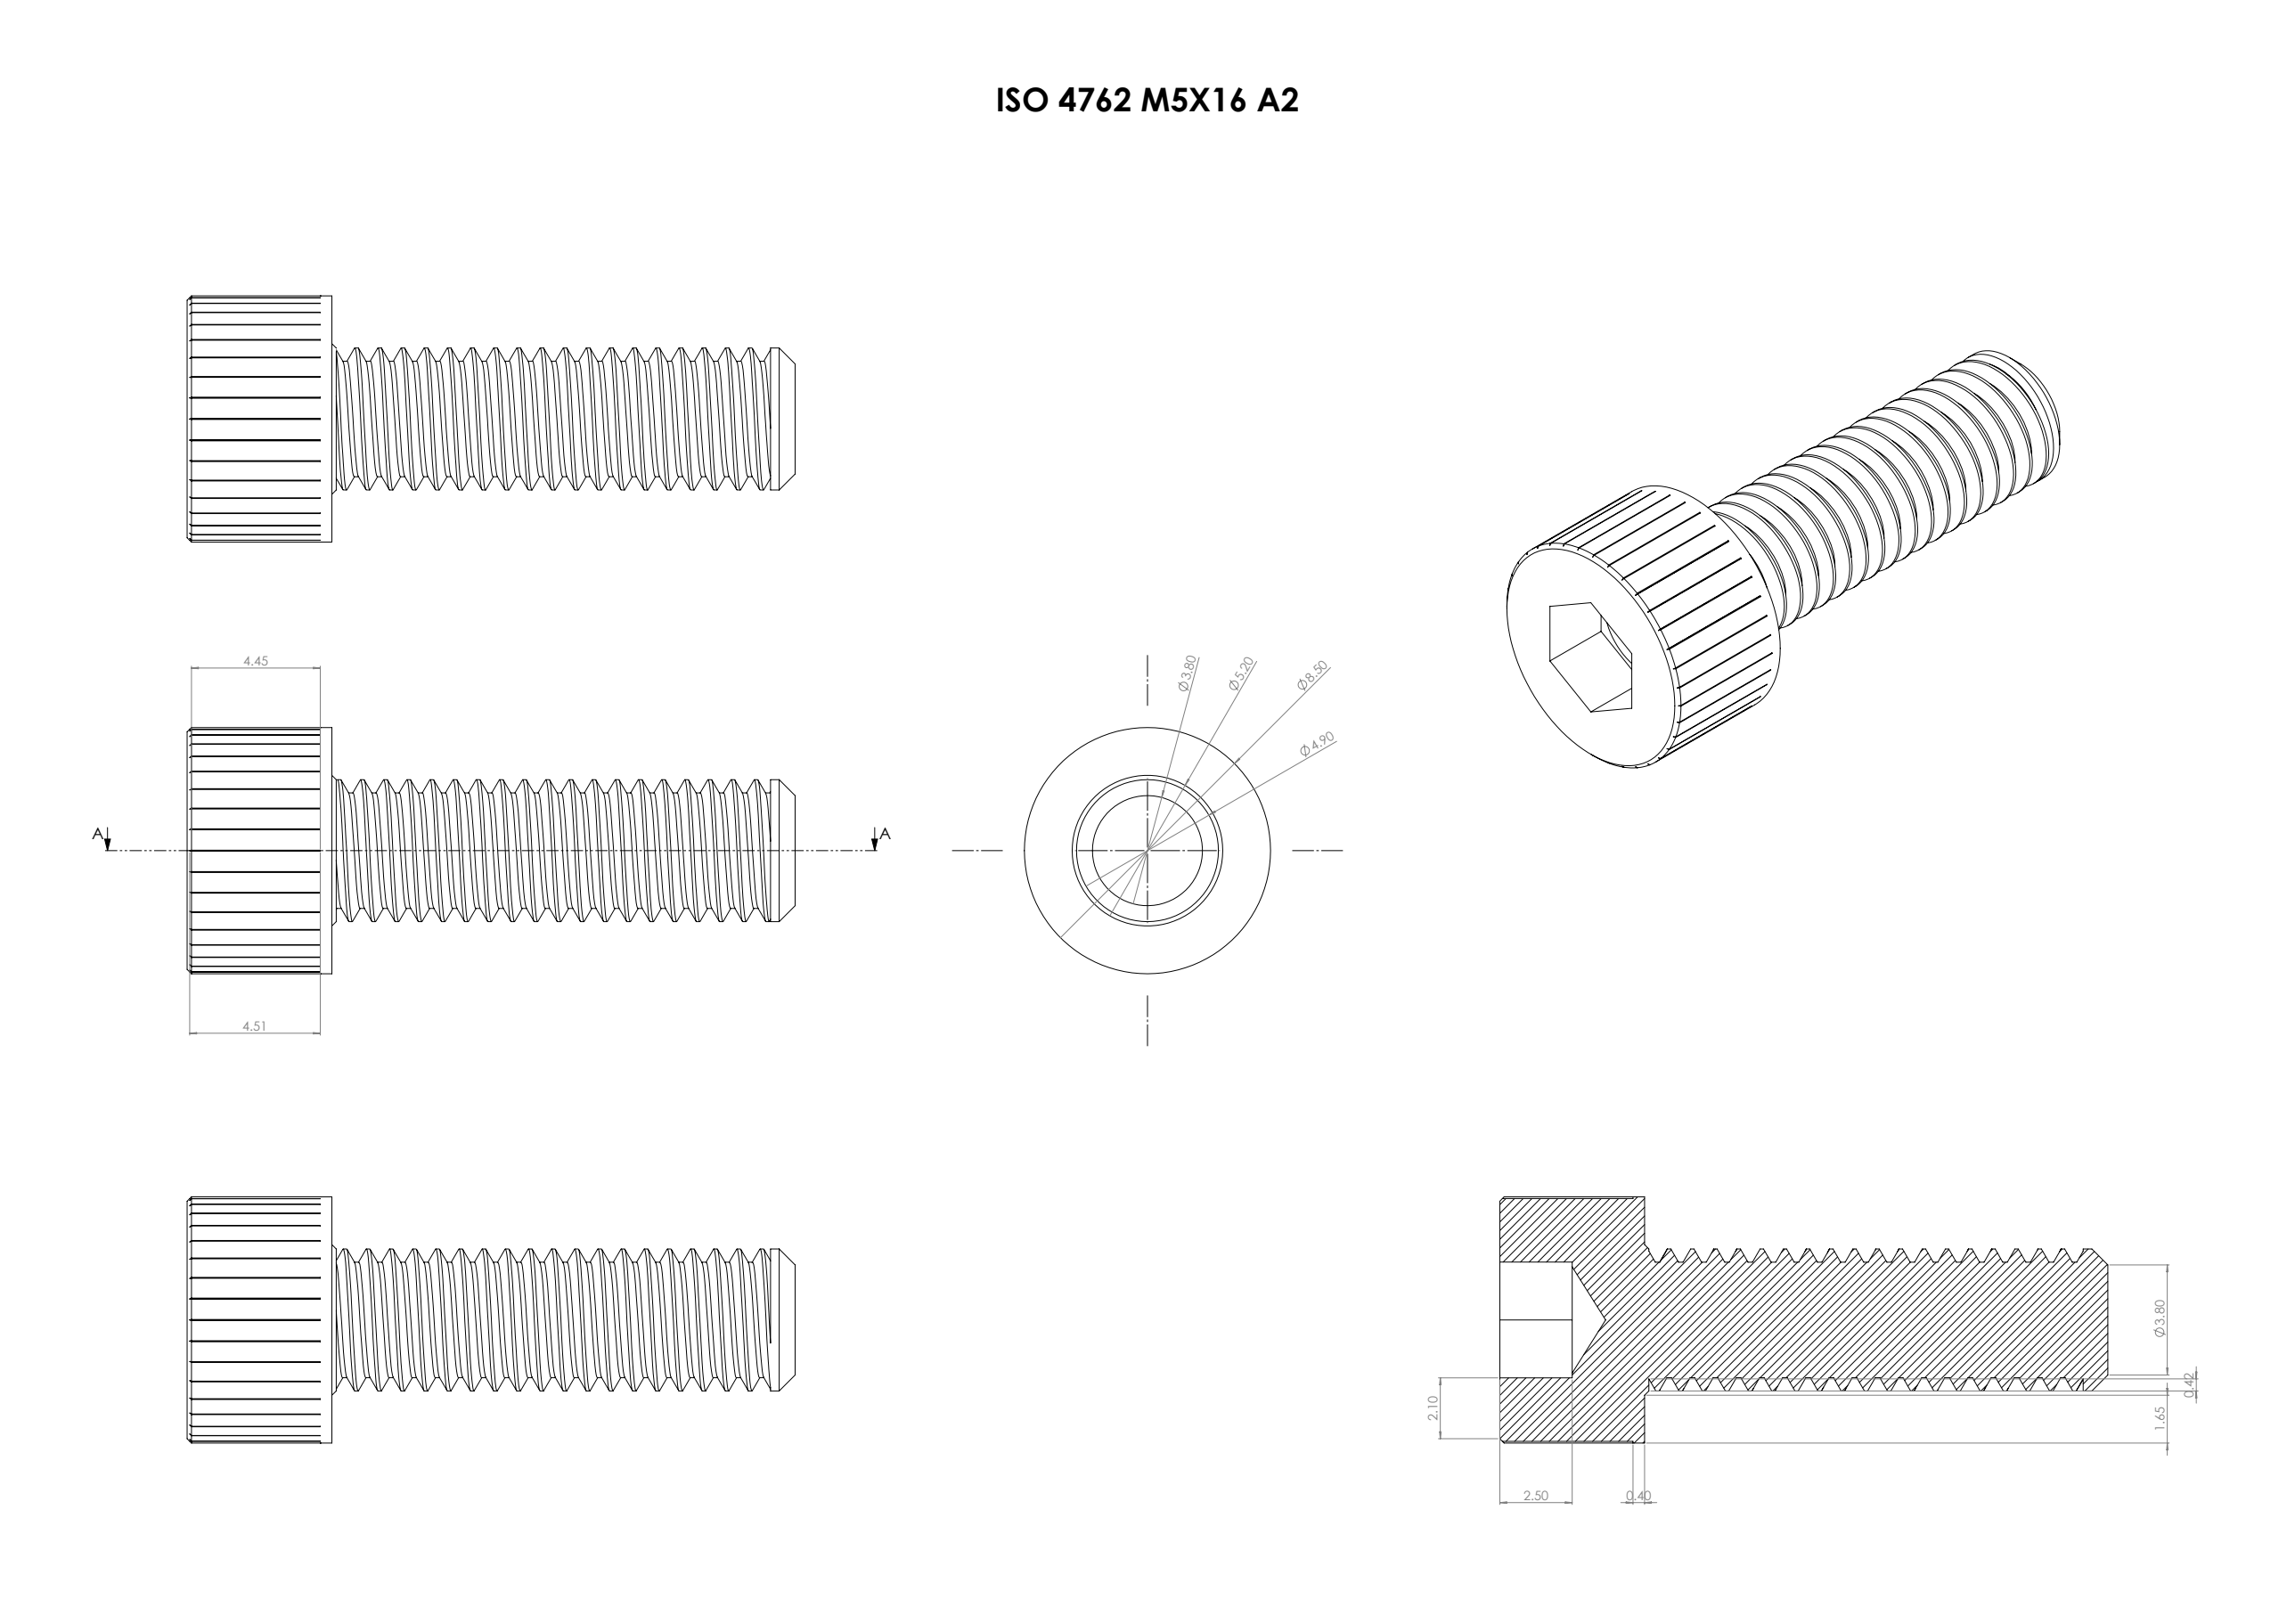
ISO-10303-21;
HEADER;
/* Generated by software containing ST-Developer
 * from STEP Tools, Inc. (www.steptools.com) 
 */

FILE_DESCRIPTION(
/* description */ (''),
/* implementation_level */ '2;1');

FILE_NAME(
/* name */ '16_ISO_4762_M5x16_A2.step',
/* time_stamp */ '2026-10-19T22:59:19-07:00',
/* author */ (''),
/* organization */ (''),
/* preprocessor_version */ 'ST-DEVELOPER v20.2',
/* originating_system */ 'Autodesk Translation Framework v15.15.0.0',
/* authorisation */ '');

FILE_SCHEMA (('AUTOMOTIVE_DESIGN { 1 0 10303 214 3 1 1 }'));
ENDSEC;

DATA;
#10=MECHANICAL_DESIGN_GEOMETRIC_PRESENTATION_REPRESENTATION('',(#926),#53650);
#291=(
BOUNDED_CURVE()
B_SPLINE_CURVE(2,(#52736,#52737,#52738),.UNSPECIFIED.,.F.,.F.)
B_SPLINE_CURVE_WITH_KNOTS((3,3),(0.,0.00853918025720996),.UNSPECIFIED.)
CURVE()
GEOMETRIC_REPRESENTATION_ITEM()
RATIONAL_B_SPLINE_CURVE((1.,1.00006847609056,1.000082803656))
REPRESENTATION_ITEM('')
);
#292=(
BOUNDED_CURVE()
B_SPLINE_CURVE(2,(#52742,#52743,#52744),.UNSPECIFIED.,.F.,.F.)
B_SPLINE_CURVE_WITH_KNOTS((3,3),(0.0130580720892981,0.0215972523464016),
 .UNSPECIFIED.)
CURVE()
GEOMETRIC_REPRESENTATION_ITEM()
RATIONAL_B_SPLINE_CURVE((1.0000828036589,1.00006847609296,1.))
REPRESENTATION_ITEM('')
);
#293=(
BOUNDED_CURVE()
B_SPLINE_CURVE(2,(#52757,#52758,#52759),.UNSPECIFIED.,.F.,.F.)
B_SPLINE_CURVE_WITH_KNOTS((3,3),(0.,0.00853918025691421),.UNSPECIFIED.)
CURVE()
GEOMETRIC_REPRESENTATION_ITEM()
RATIONAL_B_SPLINE_CURVE((1.,1.00006847609621,1.00008280366283))
REPRESENTATION_ITEM('')
);
#294=(
BOUNDED_CURVE()
B_SPLINE_CURVE(2,(#52763,#52764,#52765),.UNSPECIFIED.,.F.,.F.)
B_SPLINE_CURVE_WITH_KNOTS((3,3),(0.0130580720898257,0.0215972523464016),
 .UNSPECIFIED.)
CURVE()
GEOMETRIC_REPRESENTATION_ITEM()
RATIONAL_B_SPLINE_CURVE((1.00008280366765,1.00006847610019,1.))
REPRESENTATION_ITEM('')
);
#295=(
BOUNDED_CURVE()
B_SPLINE_CURVE(2,(#52778,#52779,#52780),.UNSPECIFIED.,.F.,.F.)
B_SPLINE_CURVE_WITH_KNOTS((3,3),(0.,0.00853918025697634),.UNSPECIFIED.)
CURVE()
GEOMETRIC_REPRESENTATION_ITEM()
RATIONAL_B_SPLINE_CURVE((1.,1.00006847609435,1.00008280366058))
REPRESENTATION_ITEM('')
);
#296=(
BOUNDED_CURVE()
B_SPLINE_CURVE(2,(#52784,#52785,#52786),.UNSPECIFIED.,.F.,.F.)
B_SPLINE_CURVE_WITH_KNOTS((3,3),(0.0130580720892075,0.0215972523464017),
 .UNSPECIFIED.)
CURVE()
GEOMETRIC_REPRESENTATION_ITEM()
RATIONAL_B_SPLINE_CURVE((1.00008280365926,1.00006847609326,1.))
REPRESENTATION_ITEM('')
);
#297=(
BOUNDED_CURVE()
B_SPLINE_CURVE(2,(#52799,#52800,#52801),.UNSPECIFIED.,.F.,.F.)
B_SPLINE_CURVE_WITH_KNOTS((3,3),(0.,0.00853918025740409),.UNSPECIFIED.)
CURVE()
GEOMETRIC_REPRESENTATION_ITEM()
RATIONAL_B_SPLINE_CURVE((1.,1.0000684761032,1.00008280367129))
REPRESENTATION_ITEM('')
);
#298=(
BOUNDED_CURVE()
B_SPLINE_CURVE(2,(#52805,#52806,#52807),.UNSPECIFIED.,.F.,.F.)
B_SPLINE_CURVE_WITH_KNOTS((3,3),(0.0130580720892825,0.0215972523464017),
 .UNSPECIFIED.)
CURVE()
GEOMETRIC_REPRESENTATION_ITEM()
RATIONAL_B_SPLINE_CURVE((1.00008280366617,1.00006847609897,1.))
REPRESENTATION_ITEM('')
);
#299=(
BOUNDED_CURVE()
B_SPLINE_CURVE(2,(#52820,#52821,#52822),.UNSPECIFIED.,.F.,.F.)
B_SPLINE_CURVE_WITH_KNOTS((3,3),(0.,0.00853918025766262),.UNSPECIFIED.)
CURVE()
GEOMETRIC_REPRESENTATION_ITEM()
RATIONAL_B_SPLINE_CURVE((1.,1.0000684761088,1.00008280367806))
REPRESENTATION_ITEM('')
);
#300=(
BOUNDED_CURVE()
B_SPLINE_CURVE(2,(#52826,#52827,#52828),.UNSPECIFIED.,.F.,.F.)
B_SPLINE_CURVE_WITH_KNOTS((3,3),(0.0130580720892071,0.0215972523464016),
 .UNSPECIFIED.)
CURVE()
GEOMETRIC_REPRESENTATION_ITEM()
RATIONAL_B_SPLINE_CURVE((1.00008280363157,1.00006847607036,1.))
REPRESENTATION_ITEM('')
);
#301=(
BOUNDED_CURVE()
B_SPLINE_CURVE(2,(#52841,#52842,#52843),.UNSPECIFIED.,.F.,.F.)
B_SPLINE_CURVE_WITH_KNOTS((3,3),(0.,0.00853918025670973),.UNSPECIFIED.)
CURVE()
GEOMETRIC_REPRESENTATION_ITEM()
RATIONAL_B_SPLINE_CURVE((1.,1.00006847609795,1.00008280366494))
REPRESENTATION_ITEM('')
);
#302=(
BOUNDED_CURVE()
B_SPLINE_CURVE(2,(#52847,#52848,#52849),.UNSPECIFIED.,.F.,.F.)
B_SPLINE_CURVE_WITH_KNOTS((3,3),(0.0130580720892956,0.0215972523464017),
 .UNSPECIFIED.)
CURVE()
GEOMETRIC_REPRESENTATION_ITEM()
RATIONAL_B_SPLINE_CURVE((1.00008280365344,1.00006847608844,1.))
REPRESENTATION_ITEM('')
);
#303=(
BOUNDED_CURVE()
B_SPLINE_CURVE(2,(#52862,#52863,#52864),.UNSPECIFIED.,.F.,.F.)
B_SPLINE_CURVE_WITH_KNOTS((3,3),(0.,0.00853918025748816),.UNSPECIFIED.)
CURVE()
GEOMETRIC_REPRESENTATION_ITEM()
RATIONAL_B_SPLINE_CURVE((1.,1.00006847611526,1.00008280368587))
REPRESENTATION_ITEM('')
);
#304=(
BOUNDED_CURVE()
B_SPLINE_CURVE(2,(#52868,#52869,#52870),.UNSPECIFIED.,.F.,.F.)
B_SPLINE_CURVE_WITH_KNOTS((3,3),(0.0130580720891411,0.0215972523464017),
 .UNSPECIFIED.)
CURVE()
GEOMETRIC_REPRESENTATION_ITEM()
RATIONAL_B_SPLINE_CURVE((1.00008280367274,1.00006847610441,1.))
REPRESENTATION_ITEM('')
);
#305=(
BOUNDED_CURVE()
B_SPLINE_CURVE(2,(#52883,#52884,#52885),.UNSPECIFIED.,.F.,.F.)
B_SPLINE_CURVE_WITH_KNOTS((3,3),(0.,0.00853918025712499),.UNSPECIFIED.)
CURVE()
GEOMETRIC_REPRESENTATION_ITEM()
RATIONAL_B_SPLINE_CURVE((1.,1.00006847609903,1.00008280366624))
REPRESENTATION_ITEM('')
);
#306=(
BOUNDED_CURVE()
B_SPLINE_CURVE(2,(#52889,#52890,#52891),.UNSPECIFIED.,.F.,.F.)
B_SPLINE_CURVE_WITH_KNOTS((3,3),(0.0130580720891696,0.0215972523464017),
 .UNSPECIFIED.)
CURVE()
GEOMETRIC_REPRESENTATION_ITEM()
RATIONAL_B_SPLINE_CURVE((1.00008280365716,1.00006847609152,1.))
REPRESENTATION_ITEM('')
);
#307=(
BOUNDED_CURVE()
B_SPLINE_CURVE(2,(#52904,#52905,#52906),.UNSPECIFIED.,.F.,.F.)
B_SPLINE_CURVE_WITH_KNOTS((3,3),(0.,0.00853918025650805),.UNSPECIFIED.)
CURVE()
GEOMETRIC_REPRESENTATION_ITEM()
RATIONAL_B_SPLINE_CURVE((1.,1.00006847611696,1.00008280368793))
REPRESENTATION_ITEM('')
);
#308=(
BOUNDED_CURVE()
B_SPLINE_CURVE(2,(#52910,#52911,#52912),.UNSPECIFIED.,.F.,.F.)
B_SPLINE_CURVE_WITH_KNOTS((3,3),(0.0130580720893445,0.0215972523464017),
 .UNSPECIFIED.)
CURVE()
GEOMETRIC_REPRESENTATION_ITEM()
RATIONAL_B_SPLINE_CURVE((1.00008280366859,1.00006847610097,1.))
REPRESENTATION_ITEM('')
);
#309=(
BOUNDED_CURVE()
B_SPLINE_CURVE(2,(#52925,#52926,#52927),.UNSPECIFIED.,.F.,.F.)
B_SPLINE_CURVE_WITH_KNOTS((3,3),(0.,0.00853918025671517),.UNSPECIFIED.)
CURVE()
GEOMETRIC_REPRESENTATION_ITEM()
RATIONAL_B_SPLINE_CURVE((1.,1.00006847609917,1.00008280366641))
REPRESENTATION_ITEM('')
);
#310=(
BOUNDED_CURVE()
B_SPLINE_CURVE(2,(#52931,#52932,#52933),.UNSPECIFIED.,.F.,.F.)
B_SPLINE_CURVE_WITH_KNOTS((3,3),(0.013058072089299,0.0215972523464016),
 .UNSPECIFIED.)
CURVE()
GEOMETRIC_REPRESENTATION_ITEM()
RATIONAL_B_SPLINE_CURVE((1.00008280365965,1.00006847609358,1.))
REPRESENTATION_ITEM('')
);
#311=(
BOUNDED_CURVE()
B_SPLINE_CURVE(2,(#52946,#52947,#52948),.UNSPECIFIED.,.F.,.F.)
B_SPLINE_CURVE_WITH_KNOTS((3,3),(0.,0.00853918025687022),.UNSPECIFIED.)
CURVE()
GEOMETRIC_REPRESENTATION_ITEM()
RATIONAL_B_SPLINE_CURVE((1.,1.0000684761112,1.00008280368096))
REPRESENTATION_ITEM('')
);
#312=(
BOUNDED_CURVE()
B_SPLINE_CURVE(2,(#52952,#52953,#52954),.UNSPECIFIED.,.F.,.F.)
B_SPLINE_CURVE_WITH_KNOTS((3,3),(0.0130580720898527,0.0215972523464016),
 .UNSPECIFIED.)
CURVE()
GEOMETRIC_REPRESENTATION_ITEM()
RATIONAL_B_SPLINE_CURVE((1.00008280367213,1.00006847610389,1.))
REPRESENTATION_ITEM('')
);
#313=(
BOUNDED_CURVE()
B_SPLINE_CURVE(2,(#52967,#52968,#52969),.UNSPECIFIED.,.F.,.F.)
B_SPLINE_CURVE_WITH_KNOTS((3,3),(0.,0.00853918025697634),.UNSPECIFIED.)
CURVE()
GEOMETRIC_REPRESENTATION_ITEM()
RATIONAL_B_SPLINE_CURVE((1.,1.00006847609435,1.00008280366058))
REPRESENTATION_ITEM('')
);
#314=(
BOUNDED_CURVE()
B_SPLINE_CURVE(2,(#52973,#52974,#52975),.UNSPECIFIED.,.F.,.F.)
B_SPLINE_CURVE_WITH_KNOTS((3,3),(0.0130580720892075,0.0215972523464017),
 .UNSPECIFIED.)
CURVE()
GEOMETRIC_REPRESENTATION_ITEM()
RATIONAL_B_SPLINE_CURVE((1.00008280365926,1.00006847609326,1.))
REPRESENTATION_ITEM('')
);
#315=(
BOUNDED_CURVE()
B_SPLINE_CURVE(2,(#52988,#52989,#52990),.UNSPECIFIED.,.F.,.F.)
B_SPLINE_CURVE_WITH_KNOTS((3,3),(0.,0.0085391802568594),.UNSPECIFIED.)
CURVE()
GEOMETRIC_REPRESENTATION_ITEM()
RATIONAL_B_SPLINE_CURVE((1.,1.00006847609064,1.00008280365609))
REPRESENTATION_ITEM('')
);
#316=(
BOUNDED_CURVE()
B_SPLINE_CURVE(2,(#52994,#52995,#52996),.UNSPECIFIED.,.F.,.F.)
B_SPLINE_CURVE_WITH_KNOTS((3,3),(0.0130580720892872,0.0215972523464017),
 .UNSPECIFIED.)
CURVE()
GEOMETRIC_REPRESENTATION_ITEM()
RATIONAL_B_SPLINE_CURVE((1.00008280366813,1.00006847610059,1.))
REPRESENTATION_ITEM('')
);
#317=(
BOUNDED_CURVE()
B_SPLINE_CURVE(2,(#53009,#53010,#53011),.UNSPECIFIED.,.F.,.F.)
B_SPLINE_CURVE_WITH_KNOTS((3,3),(0.,0.0085391802567755),.UNSPECIFIED.)
CURVE()
GEOMETRIC_REPRESENTATION_ITEM()
RATIONAL_B_SPLINE_CURVE((1.,1.00006847609773,1.00008280366467))
REPRESENTATION_ITEM('')
);
#318=(
BOUNDED_CURVE()
B_SPLINE_CURVE(2,(#53015,#53016,#53017),.UNSPECIFIED.,.F.,.F.)
B_SPLINE_CURVE_WITH_KNOTS((3,3),(0.0130580720893092,0.0215972523464017),
 .UNSPECIFIED.)
CURVE()
GEOMETRIC_REPRESENTATION_ITEM()
RATIONAL_B_SPLINE_CURVE((1.00008280366132,1.00006847609496,1.))
REPRESENTATION_ITEM('')
);
#319=(
BOUNDED_CURVE()
B_SPLINE_CURVE(2,(#53030,#53031,#53032),.UNSPECIFIED.,.F.,.F.)
B_SPLINE_CURVE_WITH_KNOTS((3,3),(0.,0.00853918025625497),.UNSPECIFIED.)
CURVE()
GEOMETRIC_REPRESENTATION_ITEM()
RATIONAL_B_SPLINE_CURVE((1.,1.00006847611021,1.00008280367977))
REPRESENTATION_ITEM('')
);
#320=(
BOUNDED_CURVE()
B_SPLINE_CURVE(2,(#53036,#53037,#53038),.UNSPECIFIED.,.F.,.F.)
B_SPLINE_CURVE_WITH_KNOTS((3,3),(0.0130580720899158,0.0215972523464017),
 .UNSPECIFIED.)
CURVE()
GEOMETRIC_REPRESENTATION_ITEM()
RATIONAL_B_SPLINE_CURVE((1.00008280367479,1.0000684761061,1.))
REPRESENTATION_ITEM('')
);
#321=(
BOUNDED_CURVE()
B_SPLINE_CURVE(2,(#53051,#53052,#53053),.UNSPECIFIED.,.F.,.F.)
B_SPLINE_CURVE_WITH_KNOTS((3,3),(0.,0.00853918025654146),.UNSPECIFIED.)
CURVE()
GEOMETRIC_REPRESENTATION_ITEM()
RATIONAL_B_SPLINE_CURVE((1.,1.00006847611225,1.00008280368223))
REPRESENTATION_ITEM('')
);
#322=(
BOUNDED_CURVE()
B_SPLINE_CURVE(2,(#53057,#53058,#53059),.UNSPECIFIED.,.F.,.F.)
B_SPLINE_CURVE_WITH_KNOTS((3,3),(0.0130580720890747,0.0215972523464017),
 .UNSPECIFIED.)
CURVE()
GEOMETRIC_REPRESENTATION_ITEM()
RATIONAL_B_SPLINE_CURVE((1.00008280366807,1.00006847610054,1.))
REPRESENTATION_ITEM('')
);
#323=(
BOUNDED_CURVE()
B_SPLINE_CURVE(2,(#53072,#53073,#53074),.UNSPECIFIED.,.F.,.F.)
B_SPLINE_CURVE_WITH_KNOTS((3,3),(0.,0.00853918025709599),.UNSPECIFIED.)
CURVE()
GEOMETRIC_REPRESENTATION_ITEM()
RATIONAL_B_SPLINE_CURVE((1.,1.00006847610924,1.00008280367859))
REPRESENTATION_ITEM('')
);
#324=(
BOUNDED_CURVE()
B_SPLINE_CURVE(2,(#53078,#53079,#53080),.UNSPECIFIED.,.F.,.F.)
B_SPLINE_CURVE_WITH_KNOTS((3,3),(0.0130580720900087,0.0215972523464017),
 .UNSPECIFIED.)
CURVE()
GEOMETRIC_REPRESENTATION_ITEM()
RATIONAL_B_SPLINE_CURVE((1.00008280365785,1.00006847609209,1.))
REPRESENTATION_ITEM('')
);
#325=(
BOUNDED_CURVE()
B_SPLINE_CURVE(2,(#53095,#53096,#53097),.UNSPECIFIED.,.F.,.F.)
B_SPLINE_CURVE_WITH_KNOTS((3,3),(0.,0.00853918025700788),.UNSPECIFIED.)
CURVE()
GEOMETRIC_REPRESENTATION_ITEM()
RATIONAL_B_SPLINE_CURVE((1.,1.00006847611371,1.000082803684))
REPRESENTATION_ITEM('')
);
#326=(
BOUNDED_CURVE()
B_SPLINE_CURVE(2,(#53101,#53102,#53103),.UNSPECIFIED.,.F.,.F.)
B_SPLINE_CURVE_WITH_KNOTS((3,3),(0.0130580720893571,0.0215972523464017),
 .UNSPECIFIED.)
CURVE()
GEOMETRIC_REPRESENTATION_ITEM()
RATIONAL_B_SPLINE_CURVE((1.00008280366365,1.00006847609689,1.))
REPRESENTATION_ITEM('')
);
#327=(
BOUNDED_CURVE()
B_SPLINE_CURVE(2,(#53116,#53117,#53118),.UNSPECIFIED.,.F.,.F.)
B_SPLINE_CURVE_WITH_KNOTS((3,3),(0.,0.0085391802571346),.UNSPECIFIED.)
CURVE()
GEOMETRIC_REPRESENTATION_ITEM()
RATIONAL_B_SPLINE_CURVE((1.,1.00006847610954,1.00008280367896))
REPRESENTATION_ITEM('')
);
#328=(
BOUNDED_CURVE()
B_SPLINE_CURVE(2,(#53122,#53123,#53124),.UNSPECIFIED.,.F.,.F.)
B_SPLINE_CURVE_WITH_KNOTS((3,3),(0.0130580720898028,0.0215972523464017),
 .UNSPECIFIED.)
CURVE()
GEOMETRIC_REPRESENTATION_ITEM()
RATIONAL_B_SPLINE_CURVE((1.00008280367741,1.00006847610826,1.))
REPRESENTATION_ITEM('')
);
#329=(
BOUNDED_CURVE()
B_SPLINE_CURVE(2,(#53137,#53138,#53139),.UNSPECIFIED.,.F.,.F.)
B_SPLINE_CURVE_WITH_KNOTS((3,3),(0.,0.00853918025673768),.UNSPECIFIED.)
CURVE()
GEOMETRIC_REPRESENTATION_ITEM()
RATIONAL_B_SPLINE_CURVE((1.,1.00006847610804,1.00008280367714))
REPRESENTATION_ITEM('')
);
#330=(
BOUNDED_CURVE()
B_SPLINE_CURVE(2,(#53143,#53144,#53145),.UNSPECIFIED.,.F.,.F.)
B_SPLINE_CURVE_WITH_KNOTS((3,3),(0.013058072089849,0.0215972523464017),
 .UNSPECIFIED.)
CURVE()
GEOMETRIC_REPRESENTATION_ITEM()
RATIONAL_B_SPLINE_CURVE((1.0000828036755,1.00006847610668,1.))
REPRESENTATION_ITEM('')
);
#331=(
BOUNDED_CURVE()
B_SPLINE_CURVE(2,(#53158,#53159,#53160),.UNSPECIFIED.,.F.,.F.)
B_SPLINE_CURVE_WITH_KNOTS((3,3),(0.,0.00853918025708019),.UNSPECIFIED.)
CURVE()
GEOMETRIC_REPRESENTATION_ITEM()
RATIONAL_B_SPLINE_CURVE((1.,1.00006847610096,1.00008280366858))
REPRESENTATION_ITEM('')
);
#332=(
BOUNDED_CURVE()
B_SPLINE_CURVE(2,(#53164,#53165,#53166),.UNSPECIFIED.,.F.,.F.)
B_SPLINE_CURVE_WITH_KNOTS((3,3),(0.0130580720886814,0.0215972523464017),
 .UNSPECIFIED.)
CURVE()
GEOMETRIC_REPRESENTATION_ITEM()
RATIONAL_B_SPLINE_CURVE((1.00008280364451,1.00006847608106,1.))
REPRESENTATION_ITEM('')
);
#333=(
BOUNDED_CURVE()
B_SPLINE_CURVE(2,(#53179,#53180,#53181),.UNSPECIFIED.,.F.,.F.)
B_SPLINE_CURVE_WITH_KNOTS((3,3),(0.,0.0085391802568594),.UNSPECIFIED.)
CURVE()
GEOMETRIC_REPRESENTATION_ITEM()
RATIONAL_B_SPLINE_CURVE((1.,1.00006847609064,1.00008280365609))
REPRESENTATION_ITEM('')
);
#334=(
BOUNDED_CURVE()
B_SPLINE_CURVE(2,(#53185,#53186,#53187),.UNSPECIFIED.,.F.,.F.)
B_SPLINE_CURVE_WITH_KNOTS((3,3),(0.0130580720892872,0.0215972523464017),
 .UNSPECIFIED.)
CURVE()
GEOMETRIC_REPRESENTATION_ITEM()
RATIONAL_B_SPLINE_CURVE((1.00008280366813,1.00006847610059,1.))
REPRESENTATION_ITEM('')
);
#335=(
BOUNDED_CURVE()
B_SPLINE_CURVE(2,(#53200,#53201,#53202),.UNSPECIFIED.,.F.,.F.)
B_SPLINE_CURVE_WITH_KNOTS((3,3),(0.,0.00853918025666453),.UNSPECIFIED.)
CURVE()
GEOMETRIC_REPRESENTATION_ITEM()
RATIONAL_B_SPLINE_CURVE((1.,1.0000684761013,1.00008280366899))
REPRESENTATION_ITEM('')
);
#336=(
BOUNDED_CURVE()
B_SPLINE_CURVE(2,(#53206,#53207,#53208),.UNSPECIFIED.,.F.,.F.)
B_SPLINE_CURVE_WITH_KNOTS((3,3),(0.013058072089416,0.0215972523464017),
 .UNSPECIFIED.)
CURVE()
GEOMETRIC_REPRESENTATION_ITEM()
RATIONAL_B_SPLINE_CURVE((1.00008280367373,1.00006847610522,1.))
REPRESENTATION_ITEM('')
);
#337=(
BOUNDED_CURVE()
B_SPLINE_CURVE(2,(#53221,#53222,#53223),.UNSPECIFIED.,.F.,.F.)
B_SPLINE_CURVE_WITH_KNOTS((3,3),(0.,0.00853918025670855),.UNSPECIFIED.)
CURVE()
GEOMETRIC_REPRESENTATION_ITEM()
RATIONAL_B_SPLINE_CURVE((1.,1.00006847610409,1.00008280367237))
REPRESENTATION_ITEM('')
);
#338=(
BOUNDED_CURVE()
B_SPLINE_CURVE(2,(#53227,#53228,#53229),.UNSPECIFIED.,.F.,.F.)
B_SPLINE_CURVE_WITH_KNOTS((3,3),(0.0130580720894821,0.0215972523464016),
 .UNSPECIFIED.)
CURVE()
GEOMETRIC_REPRESENTATION_ITEM()
RATIONAL_B_SPLINE_CURVE((1.00008280368423,1.00006847611391,1.))
REPRESENTATION_ITEM('')
);
#339=(
BOUNDED_CURVE()
B_SPLINE_CURVE(2,(#53242,#53243,#53244),.UNSPECIFIED.,.F.,.F.)
B_SPLINE_CURVE_WITH_KNOTS((3,3),(0.,0.00853918025654146),.UNSPECIFIED.)
CURVE()
GEOMETRIC_REPRESENTATION_ITEM()
RATIONAL_B_SPLINE_CURVE((1.,1.00006847611225,1.00008280368223))
REPRESENTATION_ITEM('')
);
#340=(
BOUNDED_CURVE()
B_SPLINE_CURVE(2,(#53248,#53249,#53250),.UNSPECIFIED.,.F.,.F.)
B_SPLINE_CURVE_WITH_KNOTS((3,3),(0.0130580720890747,0.0215972523464017),
 .UNSPECIFIED.)
CURVE()
GEOMETRIC_REPRESENTATION_ITEM()
RATIONAL_B_SPLINE_CURVE((1.00008280366807,1.00006847610054,1.))
REPRESENTATION_ITEM('')
);
#341=(
BOUNDED_CURVE()
B_SPLINE_CURVE(2,(#53263,#53264,#53265),.UNSPECIFIED.,.F.,.F.)
B_SPLINE_CURVE_WITH_KNOTS((3,3),(0.,0.00853918025706428),.UNSPECIFIED.)
CURVE()
GEOMETRIC_REPRESENTATION_ITEM()
RATIONAL_B_SPLINE_CURVE((1.,1.00006847610177,1.00008280366956))
REPRESENTATION_ITEM('')
);
#342=(
BOUNDED_CURVE()
B_SPLINE_CURVE(2,(#53269,#53270,#53271),.UNSPECIFIED.,.F.,.F.)
B_SPLINE_CURVE_WITH_KNOTS((3,3),(0.013058072089191,0.0215972523464017),
 .UNSPECIFIED.)
CURVE()
GEOMETRIC_REPRESENTATION_ITEM()
RATIONAL_B_SPLINE_CURVE((1.00008280366799,1.00006847610048,1.))
REPRESENTATION_ITEM('')
);
#343=(
BOUNDED_CURVE()
B_SPLINE_CURVE(2,(#53284,#53285,#53286),.UNSPECIFIED.,.F.,.F.)
B_SPLINE_CURVE_WITH_KNOTS((3,3),(0.,0.00853918025704869),.UNSPECIFIED.)
CURVE()
GEOMETRIC_REPRESENTATION_ITEM()
RATIONAL_B_SPLINE_CURVE((1.,1.00006847609971,1.00008280366706))
REPRESENTATION_ITEM('')
);
#344=(
BOUNDED_CURVE()
B_SPLINE_CURVE(2,(#53290,#53291,#53292),.UNSPECIFIED.,.F.,.F.)
B_SPLINE_CURVE_WITH_KNOTS((3,3),(0.0130580720893516,0.0215972523464017),
 .UNSPECIFIED.)
CURVE()
GEOMETRIC_REPRESENTATION_ITEM()
RATIONAL_B_SPLINE_CURVE((1.00008280366174,1.0000684760953,1.))
REPRESENTATION_ITEM('')
);
#345=(
BOUNDED_CURVE()
B_SPLINE_CURVE(2,(#53305,#53306,#53307),.UNSPECIFIED.,.F.,.F.)
B_SPLINE_CURVE_WITH_KNOTS((3,3),(0.,0.00853918025720127),.UNSPECIFIED.)
CURVE()
GEOMETRIC_REPRESENTATION_ITEM()
RATIONAL_B_SPLINE_CURVE((1.,1.0000684760941,1.00008280366028))
REPRESENTATION_ITEM('')
);
#346=(
BOUNDED_CURVE()
B_SPLINE_CURVE(2,(#53311,#53312,#53313),.UNSPECIFIED.,.F.,.F.)
B_SPLINE_CURVE_WITH_KNOTS((3,3),(0.0130580720897893,0.0215972523464017),
 .UNSPECIFIED.)
CURVE()
GEOMETRIC_REPRESENTATION_ITEM()
RATIONAL_B_SPLINE_CURVE((1.00008280367779,1.00006847610857,1.))
REPRESENTATION_ITEM('')
);
#347=(
BOUNDED_CURVE()
B_SPLINE_CURVE(2,(#53326,#53327,#53328),.UNSPECIFIED.,.F.,.F.)
B_SPLINE_CURVE_WITH_KNOTS((3,3),(0.,0.00853918025673768),.UNSPECIFIED.)
CURVE()
GEOMETRIC_REPRESENTATION_ITEM()
RATIONAL_B_SPLINE_CURVE((1.,1.00006847610804,1.00008280367714))
REPRESENTATION_ITEM('')
);
#348=(
BOUNDED_CURVE()
B_SPLINE_CURVE(2,(#53332,#53333,#53334),.UNSPECIFIED.,.F.,.F.)
B_SPLINE_CURVE_WITH_KNOTS((3,3),(0.013058072089849,0.0215972523464017),
 .UNSPECIFIED.)
CURVE()
GEOMETRIC_REPRESENTATION_ITEM()
RATIONAL_B_SPLINE_CURVE((1.0000828036755,1.00006847610668,1.))
REPRESENTATION_ITEM('')
);
#349=(
BOUNDED_CURVE()
B_SPLINE_CURVE(2,(#53347,#53348,#53349),.UNSPECIFIED.,.F.,.F.)
B_SPLINE_CURVE_WITH_KNOTS((3,3),(0.,0.00853918025648162),.UNSPECIFIED.)
CURVE()
GEOMETRIC_REPRESENTATION_ITEM()
RATIONAL_B_SPLINE_CURVE((1.,1.00006847611061,1.00008280368025))
REPRESENTATION_ITEM('')
);
#350=(
BOUNDED_CURVE()
B_SPLINE_CURVE(2,(#53353,#53354,#53355),.UNSPECIFIED.,.F.,.F.)
B_SPLINE_CURVE_WITH_KNOTS((3,3),(0.0130580720891761,0.0215972523464017),
 .UNSPECIFIED.)
CURVE()
GEOMETRIC_REPRESENTATION_ITEM()
RATIONAL_B_SPLINE_CURVE((1.00008280364825,1.00006847608415,1.))
REPRESENTATION_ITEM('')
);
#351=(
BOUNDED_CURVE()
B_SPLINE_CURVE(2,(#53368,#53369,#53370),.UNSPECIFIED.,.F.,.F.)
B_SPLINE_CURVE_WITH_KNOTS((3,3),(0.,0.00853918025753211),.UNSPECIFIED.)
CURVE()
GEOMETRIC_REPRESENTATION_ITEM()
RATIONAL_B_SPLINE_CURVE((1.,1.00006847610271,1.0000828036707))
REPRESENTATION_ITEM('')
);
#352=(
BOUNDED_CURVE()
B_SPLINE_CURVE(2,(#53374,#53375,#53376),.UNSPECIFIED.,.F.,.F.)
B_SPLINE_CURVE_WITH_KNOTS((3,3),(0.0130580720891711,0.0215972523464017),
 .UNSPECIFIED.)
CURVE()
GEOMETRIC_REPRESENTATION_ITEM()
RATIONAL_B_SPLINE_CURVE((1.00008280365529,1.00006847608997,1.))
REPRESENTATION_ITEM('')
);
#353=(
BOUNDED_CURVE()
B_SPLINE_CURVE(2,(#53389,#53390,#53391),.UNSPECIFIED.,.F.,.F.)
B_SPLINE_CURVE_WITH_KNOTS((3,3),(0.,0.0085391802567755),.UNSPECIFIED.)
CURVE()
GEOMETRIC_REPRESENTATION_ITEM()
RATIONAL_B_SPLINE_CURVE((1.,1.00006847609773,1.00008280366467))
REPRESENTATION_ITEM('')
);
#354=(
BOUNDED_CURVE()
B_SPLINE_CURVE(2,(#53395,#53396,#53397),.UNSPECIFIED.,.F.,.F.)
B_SPLINE_CURVE_WITH_KNOTS((3,3),(0.0130580720893092,0.0215972523464017),
 .UNSPECIFIED.)
CURVE()
GEOMETRIC_REPRESENTATION_ITEM()
RATIONAL_B_SPLINE_CURVE((1.00008280366132,1.00006847609496,1.))
REPRESENTATION_ITEM('')
);
#355=(
BOUNDED_CURVE()
B_SPLINE_CURVE(2,(#53410,#53411,#53412),.UNSPECIFIED.,.F.,.F.)
B_SPLINE_CURVE_WITH_KNOTS((3,3),(0.,0.00853918025675444),.UNSPECIFIED.)
CURVE()
GEOMETRIC_REPRESENTATION_ITEM()
RATIONAL_B_SPLINE_CURVE((1.,1.00006847610301,1.00008280367106))
REPRESENTATION_ITEM('')
);
#356=(
BOUNDED_CURVE()
B_SPLINE_CURVE(2,(#53416,#53417,#53418),.UNSPECIFIED.,.F.,.F.)
B_SPLINE_CURVE_WITH_KNOTS((3,3),(0.0130580720893406,0.0215972523464017),
 .UNSPECIFIED.)
CURVE()
GEOMETRIC_REPRESENTATION_ITEM()
RATIONAL_B_SPLINE_CURVE((1.00008280367253,1.00006847610423,1.))
REPRESENTATION_ITEM('')
);
#357=(
BOUNDED_CURVE()
B_SPLINE_CURVE(2,(#53431,#53432,#53433),.UNSPECIFIED.,.F.,.F.)
B_SPLINE_CURVE_WITH_KNOTS((3,3),(0.,0.00853918025654146),.UNSPECIFIED.)
CURVE()
GEOMETRIC_REPRESENTATION_ITEM()
RATIONAL_B_SPLINE_CURVE((1.,1.00006847611225,1.00008280368223))
REPRESENTATION_ITEM('')
);
#358=(
BOUNDED_CURVE()
B_SPLINE_CURVE(2,(#53437,#53438,#53439),.UNSPECIFIED.,.F.,.F.)
B_SPLINE_CURVE_WITH_KNOTS((3,3),(0.0130580720890747,0.0215972523464017),
 .UNSPECIFIED.)
CURVE()
GEOMETRIC_REPRESENTATION_ITEM()
RATIONAL_B_SPLINE_CURVE((1.00008280366807,1.00006847610054,1.))
REPRESENTATION_ITEM('')
);
#359=(
BOUNDED_CURVE()
B_SPLINE_CURVE(2,(#53452,#53453,#53454),.UNSPECIFIED.,.F.,.F.)
B_SPLINE_CURVE_WITH_KNOTS((3,3),(0.,0.00853918025712073),.UNSPECIFIED.)
CURVE()
GEOMETRIC_REPRESENTATION_ITEM()
RATIONAL_B_SPLINE_CURVE((1.,1.00006847609561,1.0000828036621))
REPRESENTATION_ITEM('')
);
#360=(
BOUNDED_CURVE()
B_SPLINE_CURVE(2,(#53458,#53459,#53460),.UNSPECIFIED.,.F.,.F.)
B_SPLINE_CURVE_WITH_KNOTS((3,3),(0.0130580720897129,0.0215972523464017),
 .UNSPECIFIED.)
CURVE()
GEOMETRIC_REPRESENTATION_ITEM()
RATIONAL_B_SPLINE_CURVE((1.00008280368364,1.00006847611341,1.))
REPRESENTATION_ITEM('')
);
#361=(
BOUNDED_CURVE()
B_SPLINE_CURVE(2,(#53513,#53514,#53515),.UNSPECIFIED.,.F.,.F.)
B_SPLINE_CURVE_WITH_KNOTS((3,3),(0.,0.00853918025702907),.UNSPECIFIED.)
CURVE()
GEOMETRIC_REPRESENTATION_ITEM()
RATIONAL_B_SPLINE_CURVE((1.,1.00006847610662,1.00008280367543))
REPRESENTATION_ITEM('')
);
#362=(
BOUNDED_CURVE()
B_SPLINE_CURVE(2,(#53517,#53518,#53519),.UNSPECIFIED.,.F.,.F.)
B_SPLINE_CURVE_WITH_KNOTS((3,3),(0.0130580720893726,0.0215972523464017),
 .UNSPECIFIED.)
CURVE()
GEOMETRIC_REPRESENTATION_ITEM()
RATIONAL_B_SPLINE_CURVE((1.00008280367543,1.00006847610662,1.))
REPRESENTATION_ITEM('')
);
#371=B_SPLINE_SURFACE_WITH_KNOTS('',3,3,((#51566,#51567,#51568,#51569,#51570,
#51571,#51572,#51573,#51574,#51575,#51576,#51577,#51578,#51579,#51580,#51581,
#51582,#51583,#51584,#51585,#51586,#51587,#51588,#51589,#51590,#51591,#51592,
#51593,#51594,#51595,#51596,#51597,#51598,#51599,#51600,#51601,#51602,#51603,
#51604,#51605,#51606,#51607,#51608,#51609,#51610,#51611,#51612,#51613,#51614,
#51615,#51616,#51617,#51618,#51619,#51620,#51621,#51622,#51623,#51624,#51625,
#51626,#51627,#51628,#51629,#51630,#51631,#51632,#51633,#51634,#51635,#51636,
#51637,#51638,#51639,#51640,#51641,#51642,#51643,#51644,#51645,#51646,#51647,
#51648,#51649,#51650,#51651,#51652,#51653,#51654,#51655,#51656,#51657,#51658,
#51659,#51660,#51661,#51662,#51663,#51664,#51665,#51666,#51667,#51668,#51669,
#51670,#51671,#51672,#51673,#51674,#51675,#51676,#51677,#51678,#51679,#51680,
#51681,#51682,#51683,#51684,#51685,#51686,#51687,#51688),(#51689,#51690,
#51691,#51692,#51693,#51694,#51695,#51696,#51697,#51698,#51699,#51700,#51701,
#51702,#51703,#51704,#51705,#51706,#51707,#51708,#51709,#51710,#51711,#51712,
#51713,#51714,#51715,#51716,#51717,#51718,#51719,#51720,#51721,#51722,#51723,
#51724,#51725,#51726,#51727,#51728,#51729,#51730,#51731,#51732,#51733,#51734,
#51735,#51736,#51737,#51738,#51739,#51740,#51741,#51742,#51743,#51744,#51745,
#51746,#51747,#51748,#51749,#51750,#51751,#51752,#51753,#51754,#51755,#51756,
#51757,#51758,#51759,#51760,#51761,#51762,#51763,#51764,#51765,#51766,#51767,
#51768,#51769,#51770,#51771,#51772,#51773,#51774,#51775,#51776,#51777,#51778,
#51779,#51780,#51781,#51782,#51783,#51784,#51785,#51786,#51787,#51788,#51789,
#51790,#51791,#51792,#51793,#51794,#51795,#51796,#51797,#51798,#51799,#51800,
#51801,#51802,#51803,#51804,#51805,#51806,#51807,#51808,#51809,#51810,#51811),
(#51812,#51813,#51814,#51815,#51816,#51817,#51818,#51819,#51820,#51821,
#51822,#51823,#51824,#51825,#51826,#51827,#51828,#51829,#51830,#51831,#51832,
#51833,#51834,#51835,#51836,#51837,#51838,#51839,#51840,#51841,#51842,#51843,
#51844,#51845,#51846,#51847,#51848,#51849,#51850,#51851,#51852,#51853,#51854,
#51855,#51856,#51857,#51858,#51859,#51860,#51861,#51862,#51863,#51864,#51865,
#51866,#51867,#51868,#51869,#51870,#51871,#51872,#51873,#51874,#51875,#51876,
#51877,#51878,#51879,#51880,#51881,#51882,#51883,#51884,#51885,#51886,#51887,
#51888,#51889,#51890,#51891,#51892,#51893,#51894,#51895,#51896,#51897,#51898,
#51899,#51900,#51901,#51902,#51903,#51904,#51905,#51906,#51907,#51908,#51909,
#51910,#51911,#51912,#51913,#51914,#51915,#51916,#51917,#51918,#51919,#51920,
#51921,#51922,#51923,#51924,#51925,#51926,#51927,#51928,#51929,#51930,#51931,
#51932,#51933,#51934),(#51935,#51936,#51937,#51938,#51939,#51940,#51941,
#51942,#51943,#51944,#51945,#51946,#51947,#51948,#51949,#51950,#51951,#51952,
#51953,#51954,#51955,#51956,#51957,#51958,#51959,#51960,#51961,#51962,#51963,
#51964,#51965,#51966,#51967,#51968,#51969,#51970,#51971,#51972,#51973,#51974,
#51975,#51976,#51977,#51978,#51979,#51980,#51981,#51982,#51983,#51984,#51985,
#51986,#51987,#51988,#51989,#51990,#51991,#51992,#51993,#51994,#51995,#51996,
#51997,#51998,#51999,#52000,#52001,#52002,#52003,#52004,#52005,#52006,#52007,
#52008,#52009,#52010,#52011,#52012,#52013,#52014,#52015,#52016,#52017,#52018,
#52019,#52020,#52021,#52022,#52023,#52024,#52025,#52026,#52027,#52028,#52029,
#52030,#52031,#52032,#52033,#52034,#52035,#52036,#52037,#52038,#52039,#52040,
#52041,#52042,#52043,#52044,#52045,#52046,#52047,#52048,#52049,#52050,#52051,
#52052,#52053,#52054,#52055,#52056,#52057)),.UNSPECIFIED.,.F.,.F.,.F.,(4,
4),(4,1,1,1,1,1,1,1,1,1,1,1,1,1,1,1,1,1,1,1,1,1,1,1,1,1,1,1,1,1,1,1,1,1,
1,1,1,1,1,1,1,1,1,1,1,1,1,1,1,1,1,1,1,1,1,1,1,1,1,1,1,1,1,1,1,1,1,1,1,1,
1,1,1,1,1,1,1,1,1,1,1,1,1,1,1,1,1,1,1,1,1,1,1,1,1,1,1,1,1,1,1,1,1,1,1,1,
1,1,1,1,1,1,1,1,1,1,1,1,1,1,4),(0.,0.0526254770366343),(10.6643522173549,
11.6633215686903,12.6622909200256,13.661260271361,14.6602296226963,15.6591989740317,
16.658168325367,17.6571376767024,18.6561070280377,19.6550763793731,20.6540457307084,
21.6530150820438,22.6519844333791,23.6509537847144,24.6499231360498,25.6488924873851,
26.6478618387205,27.6468311900558,28.6458005413912,29.6447698927265,30.6437392440619,
31.6427085953972,32.6416779467326,33.6406472980679,34.6396166494033,35.6385860007386,
36.6375553520739,37.6365247034093,38.6354940547446,39.63446340608,40.6334327574153,
41.6324021087507,42.631371460086,43.6303408114214,44.6293101627567,45.6282795140921,
46.6272488654274,47.6262182167628,48.6251875680981,49.6241569194335,50.6231262707688,
51.6220956221041,52.6210649734395,53.6200343247748,54.6190036761102,55.6179730274455,
56.6169423787809,57.6159117301162,58.6148810814516,59.6138504327869,60.6128197841223,
61.6117891354576,62.610758486793,63.6097278381283,64.6086971894637,65.607666540799,
66.6066358921343,67.6056052434697,68.604574594805,69.6035439461404,70.6025132974757,
71.6014826488111,72.6004520001464,73.5994213514818,74.5983907028171,75.5973600541525,
76.5963294054878,77.5952987568232,78.5942681081585,79.5932374594938,80.5922068108292,
81.5911761621645,82.5901455134999,83.5891148648352,84.5880842161706,85.5870535675059,
86.5860229188413,87.5849922701766,88.583961621512,89.5829309728473,90.5819003241827,
91.580869675518,92.5798390268534,93.5788083781887,94.5777777295241,95.5767470808594,
96.5757164321948,97.5746857835301,98.5736551348654,99.5726244862008,100.571593837536,
101.570563188871,102.569532540207,103.568501891542,104.567471242878,105.566440594213,
106.565409945548,107.564379296884,108.563348648219,109.562317999554,110.56128735089,
111.560256702225,112.55922605356,113.558195404896,114.557164756231,115.556134107566,
116.555103458902,117.554072810237,118.553042161572,119.552011512908,120.550980864243,
121.549950215578,122.548919566914,123.547888918249,124.546858269584,125.54582762092,
126.544796972255,127.54376632359,128.542735674926,129.541705026261,130.540674377597),
 .UNSPECIFIED.);
#372=B_SPLINE_SURFACE_WITH_KNOTS('',3,3,((#52213,#52214,#52215,#52216,#52217,
#52218,#52219,#52220,#52221,#52222,#52223,#52224,#52225,#52226,#52227,#52228,
#52229,#52230,#52231,#52232,#52233,#52234,#52235,#52236,#52237,#52238,#52239,
#52240,#52241,#52242,#52243,#52244,#52245,#52246,#52247,#52248,#52249,#52250,
#52251,#52252,#52253,#52254,#52255,#52256,#52257,#52258,#52259,#52260,#52261,
#52262,#52263,#52264,#52265,#52266,#52267,#52268,#52269,#52270,#52271,#52272,
#52273,#52274,#52275,#52276,#52277,#52278,#52279,#52280,#52281,#52282,#52283,
#52284,#52285,#52286,#52287,#52288,#52289,#52290,#52291,#52292,#52293,#52294,
#52295,#52296,#52297,#52298,#52299,#52300,#52301,#52302,#52303,#52304,#52305,
#52306,#52307,#52308,#52309,#52310,#52311,#52312,#52313,#52314,#52315,#52316,
#52317,#52318,#52319,#52320,#52321,#52322,#52323,#52324,#52325,#52326,#52327,
#52328,#52329,#52330,#52331,#52332,#52333,#52334,#52335),(#52336,#52337,
#52338,#52339,#52340,#52341,#52342,#52343,#52344,#52345,#52346,#52347,#52348,
#52349,#52350,#52351,#52352,#52353,#52354,#52355,#52356,#52357,#52358,#52359,
#52360,#52361,#52362,#52363,#52364,#52365,#52366,#52367,#52368,#52369,#52370,
#52371,#52372,#52373,#52374,#52375,#52376,#52377,#52378,#52379,#52380,#52381,
#52382,#52383,#52384,#52385,#52386,#52387,#52388,#52389,#52390,#52391,#52392,
#52393,#52394,#52395,#52396,#52397,#52398,#52399,#52400,#52401,#52402,#52403,
#52404,#52405,#52406,#52407,#52408,#52409,#52410,#52411,#52412,#52413,#52414,
#52415,#52416,#52417,#52418,#52419,#52420,#52421,#52422,#52423,#52424,#52425,
#52426,#52427,#52428,#52429,#52430,#52431,#52432,#52433,#52434,#52435,#52436,
#52437,#52438,#52439,#52440,#52441,#52442,#52443,#52444,#52445,#52446,#52447,
#52448,#52449,#52450,#52451,#52452,#52453,#52454,#52455,#52456,#52457,#52458),
(#52459,#52460,#52461,#52462,#52463,#52464,#52465,#52466,#52467,#52468,
#52469,#52470,#52471,#52472,#52473,#52474,#52475,#52476,#52477,#52478,#52479,
#52480,#52481,#52482,#52483,#52484,#52485,#52486,#52487,#52488,#52489,#52490,
#52491,#52492,#52493,#52494,#52495,#52496,#52497,#52498,#52499,#52500,#52501,
#52502,#52503,#52504,#52505,#52506,#52507,#52508,#52509,#52510,#52511,#52512,
#52513,#52514,#52515,#52516,#52517,#52518,#52519,#52520,#52521,#52522,#52523,
#52524,#52525,#52526,#52527,#52528,#52529,#52530,#52531,#52532,#52533,#52534,
#52535,#52536,#52537,#52538,#52539,#52540,#52541,#52542,#52543,#52544,#52545,
#52546,#52547,#52548,#52549,#52550,#52551,#52552,#52553,#52554,#52555,#52556,
#52557,#52558,#52559,#52560,#52561,#52562,#52563,#52564,#52565,#52566,#52567,
#52568,#52569,#52570,#52571,#52572,#52573,#52574,#52575,#52576,#52577,#52578,
#52579,#52580,#52581),(#52582,#52583,#52584,#52585,#52586,#52587,#52588,
#52589,#52590,#52591,#52592,#52593,#52594,#52595,#52596,#52597,#52598,#52599,
#52600,#52601,#52602,#52603,#52604,#52605,#52606,#52607,#52608,#52609,#52610,
#52611,#52612,#52613,#52614,#52615,#52616,#52617,#52618,#52619,#52620,#52621,
#52622,#52623,#52624,#52625,#52626,#52627,#52628,#52629,#52630,#52631,#52632,
#52633,#52634,#52635,#52636,#52637,#52638,#52639,#52640,#52641,#52642,#52643,
#52644,#52645,#52646,#52647,#52648,#52649,#52650,#52651,#52652,#52653,#52654,
#52655,#52656,#52657,#52658,#52659,#52660,#52661,#52662,#52663,#52664,#52665,
#52666,#52667,#52668,#52669,#52670,#52671,#52672,#52673,#52674,#52675,#52676,
#52677,#52678,#52679,#52680,#52681,#52682,#52683,#52684,#52685,#52686,#52687,
#52688,#52689,#52690,#52691,#52692,#52693,#52694,#52695,#52696,#52697,#52698,
#52699,#52700,#52701,#52702,#52703,#52704)),.UNSPECIFIED.,.F.,.F.,.F.,(4,
4),(4,1,1,1,1,1,1,1,1,1,1,1,1,1,1,1,1,1,1,1,1,1,1,1,1,1,1,1,1,1,1,1,1,1,
1,1,1,1,1,1,1,1,1,1,1,1,1,1,1,1,1,1,1,1,1,1,1,1,1,1,1,1,1,1,1,1,1,1,1,1,
1,1,1,1,1,1,1,1,1,1,1,1,1,1,1,1,1,1,1,1,1,1,1,1,1,1,1,1,1,1,1,1,1,1,1,1,
1,1,1,1,1,1,1,1,1,1,1,1,1,1,4),(0.,0.0526254770366343),(13.9725876875337,
14.9715570388691,15.9705263902044,16.9694957415398,17.9684650928751,18.9674344442105,
19.9664037955458,20.9653731468812,21.9643424982165,22.9633118495519,23.9622812008872,
24.9612505522226,25.9602199035579,26.9591892548932,27.9581586062286,28.9571279575639,
29.9560973088993,30.9550666602346,31.95403601157,32.9530053629053,33.9519747142407,
34.950944065576,35.9499134169114,36.9488827682467,37.9478521195821,38.9468214709174,
39.9457908222528,40.9447601735881,41.9437295249234,42.9426988762588,43.9416682275941,
44.9406375789295,45.9396069302648,46.9385762816002,47.9375456329355,48.9365149842709,
49.9354843356062,50.9344536869416,51.9334230382769,52.9323923896123,53.9313617409476,
54.930331092283,55.9293004436183,56.9282697949536,57.927239146289,58.9262084976243,
59.9251778489597,60.924147200295,61.9231165516304,62.9220859029657,63.9210552543011,
64.9200246056364,65.9189939569718,66.9179633083071,67.9169326596425,68.9159020109778,
69.9148713623132,70.9138407136485,71.9128100649839,72.9117794163192,73.9107487676546,
74.9097181189899,75.9086874703252,76.9076568216606,77.9066261729959,78.9055955243313,
79.9045648756666,80.903534227002,81.9025035783373,82.9014729296727,83.900442281008,
84.8994116323434,85.8983809836787,86.8973503350141,87.8963196863494,88.8952890376847,
89.8942583890201,90.8932277403554,91.8921970916908,92.8911664430261,93.8901357943615,
94.8891051456968,95.8880744970322,96.8870438483675,97.8860131997029,98.8849825510382,
99.8839519023736,100.882921253709,101.881890605044,102.88085995638,103.879829307715,
104.87879865905,105.877768010386,106.876737361721,107.875706713056,108.874676064392,
109.873645415727,110.872614767062,111.871584118398,112.870553469733,113.869522821068,
114.868492172404,115.867461523739,116.866430875074,117.86540022641,118.864369577745,
119.863338929081,120.862308280416,121.861277631751,122.860246983087,123.859216334422,
124.858185685757,125.857155037093,126.856124388428,127.855093739763,128.854063091099,
129.853032442434,130.852001793769,131.850971145105,132.84994049644,133.848909847775),
 .UNSPECIFIED.);
#797=B_SPLINE_CURVE_WITH_KNOTS('',3,(#50095,#50096,#50097,#50098,#50099,
#50100,#50101,#50102,#50103,#50104,#50105,#50106,#50107,#50108,#50109,#50110,
#50111,#50112,#50113,#50114,#50115,#50116),.UNSPECIFIED.,.F.,.F.,(4,3,3,
3,3,3,3,4),(-8.01856088759472,-7.99175481068278,-6.99278545934743,-5.99381610801208,
-4.99484675667673,-3.99587740534139,-2.99690805400604,-2.06659765062437),
 .UNSPECIFIED.);
#798=B_SPLINE_CURVE_WITH_KNOTS('',3,(#50124,#50125,#50126,#50127,#50128,
#50129,#50130,#50131,#50132,#50133,#50134,#50135,#50136,#50137,#50138,#50139,
#50140,#50141,#50142),.UNSPECIFIED.,.F.,.F.,(4,3,3,3,3,3,4),(0.,0.99896935133533,
1.99793870267068,2.99690805400603,3.99587740534138,4.99484675667673,5.04361105059381),
 .UNSPECIFIED.);
#799=B_SPLINE_CURVE_WITH_KNOTS('',3,(#50147,#50148,#50149,#50150,#50151,
#50152,#50153,#50154,#50155,#50156,#50157,#50158,#50159,#50160,#50161,#50162,
#50163,#50164,#50165,#50166,#50167,#50168),.UNSPECIFIED.,.F.,.F.,(4,3,3,
3,3,3,3,4),(-14.3017461947743,-13.9855709186949,-12.9866015673595,-11.9876322160242,
-10.9886628646888,-9.98969351335347,-8.99072416201812,-8.01856088759472),
 .UNSPECIFIED.);
#800=B_SPLINE_CURVE_WITH_KNOTS('',3,(#50169,#50170,#50171,#50172,#50173,
#50174,#50175,#50176,#50177,#50178,#50179,#50180,#50181,#50182,#50183,#50184,
#50185,#50186,#50187,#50188,#50189,#50190),.UNSPECIFIED.,.F.,.F.,(4,3,3,
3,3,3,3,4),(5.04361105059381,5.99381610801208,6.99278545934743,7.99175481068277,
8.99072416201812,9.98969351335347,10.9886628646888,11.3267963577734),
 .UNSPECIFIED.);
#801=B_SPLINE_CURVE_WITH_KNOTS('',3,(#50195,#50196,#50197,#50198,#50199,
#50200,#50201,#50202,#50203,#50204,#50205,#50206,#50207,#50208,#50209,#50210,
#50211,#50212,#50213,#50214,#50215,#50216),.UNSPECIFIED.,.F.,.F.,(4,3,3,
3,3,3,3,4),(-20.5849315019539,-19.9793870267069,-18.9804176753716,-17.9814483240362,
-16.9824789727009,-15.9835096213656,-14.9845402700302,-14.3017461947743),
 .UNSPECIFIED.);
#802=B_SPLINE_CURVE_WITH_KNOTS('',3,(#50217,#50218,#50219,#50220,#50221,
#50222,#50223,#50224,#50225,#50226,#50227,#50228,#50229,#50230,#50231,#50232,
#50233,#50234,#50235,#50236,#50237,#50238),.UNSPECIFIED.,.F.,.F.,(4,3,3,
3,3,3,3,4),(11.3267963577734,11.9876322160242,12.9866015673595,13.9855709186949,
14.9845402700302,15.9835096213656,16.9824789727009,17.609981664953),
 .UNSPECIFIED.);
#803=B_SPLINE_CURVE_WITH_KNOTS('',3,(#50243,#50244,#50245,#50246,#50247,
#50248,#50249,#50250,#50251,#50252,#50253,#50254,#50255,#50256,#50257,#50258,
#50259,#50260,#50261,#50262,#50263,#50264),.UNSPECIFIED.,.F.,.F.,(4,3,3,
3,3,3,3,4),(-26.8681168091335,-25.973203134719,-24.9742337833837,-23.9752644320483,
-22.976295080713,-21.9773257293776,-20.9783563780423,-20.5849315019539),
 .UNSPECIFIED.);
#804=B_SPLINE_CURVE_WITH_KNOTS('',3,(#50265,#50266,#50267,#50268,#50269,
#50270,#50271,#50272,#50273,#50274,#50275,#50276,#50277,#50278,#50279,#50280,
#50281,#50282,#50283,#50284,#50285,#50286),.UNSPECIFIED.,.F.,.F.,(4,3,3,
3,3,3,3,4),(17.609981664953,17.9814483240363,18.9804176753716,19.9793870267069,
20.9783563780423,21.9773257293776,22.976295080713,23.8931669721326),
 .UNSPECIFIED.);
#805=B_SPLINE_CURVE_WITH_KNOTS('',3,(#50291,#50292,#50293,#50294,#50295,
#50296,#50297,#50298,#50299,#50300,#50301,#50302,#50303,#50304,#50305,#50306,
#50307,#50308,#50309,#50310,#50311,#50312,#50313,#50314,#50315),
 .UNSPECIFIED.,.F.,.F.,(4,3,3,3,3,3,3,3,4),(-33.1513021163131,-32.9659885940664,
-31.9670192427311,-30.9680498913958,-29.9690805400604,-28.9701111887251,
-27.9711418373897,-26.9721724860544,-26.8681168091335),.UNSPECIFIED.);
#806=B_SPLINE_CURVE_WITH_KNOTS('',3,(#50316,#50317,#50318,#50319,#50320,
#50321,#50322,#50323,#50324,#50325,#50326,#50327,#50328,#50329,#50330,#50331,
#50332,#50333,#50334,#50335,#50336,#50337,#50338,#50339,#50340),
 .UNSPECIFIED.,.F.,.F.,(4,3,3,3,3,3,3,3,4),(23.8931669721326,23.9752644320483,
24.9742337833837,25.973203134719,26.9721724860544,27.9711418373897,28.970111188725,
29.9690805400604,30.1763522793122),.UNSPECIFIED.);
#807=B_SPLINE_CURVE_WITH_KNOTS('',3,(#50345,#50346,#50347,#50348,#50349,
#50350,#50351,#50352,#50353,#50354,#50355,#50356,#50357,#50358,#50359,#50360,
#50361,#50362,#50363,#50364,#50365,#50366),.UNSPECIFIED.,.F.,.F.,(4,3,3,
3,3,3,3,4),(-39.4344874234927,-38.9598047020785,-37.9608353507432,-36.9618659994078,
-35.9628966480725,-34.9639272967371,-33.9649579454018,-33.1513021163131),
 .UNSPECIFIED.);
#808=B_SPLINE_CURVE_WITH_KNOTS('',3,(#50367,#50368,#50369,#50370,#50371,
#50372,#50373,#50374,#50375,#50376,#50377,#50378,#50379,#50380,#50381,#50382,
#50383,#50384,#50385,#50386,#50387,#50388),.UNSPECIFIED.,.F.,.F.,(4,3,3,
3,3,3,3,4),(30.1763522793122,30.9680498913957,31.9670192427311,32.9659885940664,
33.9649579454018,34.9639272967371,35.9628966480725,36.4595375864917),
 .UNSPECIFIED.);
#809=B_SPLINE_CURVE_WITH_KNOTS('',3,(#50393,#50394,#50395,#50396,#50397,
#50398,#50399,#50400,#50401,#50402,#50403,#50404,#50405,#50406,#50407,#50408,
#50409,#50410,#50411,#50412,#50413,#50414),.UNSPECIFIED.,.F.,.F.,(4,3,3,
3,3,3,3,4),(-45.7176727306722,-44.9536208100906,-43.9546514587553,-42.9556821074199,
-41.9567127560846,-40.9577434047492,-39.9587740534139,-39.4344874234927),
 .UNSPECIFIED.);
#810=B_SPLINE_CURVE_WITH_KNOTS('',3,(#50415,#50416,#50417,#50418,#50419,
#50420,#50421,#50422,#50423,#50424,#50425,#50426,#50427,#50428,#50429,#50430,
#50431,#50432,#50433,#50434,#50435,#50436),.UNSPECIFIED.,.F.,.F.,(4,3,3,
3,3,3,3,4),(36.4595375864917,36.9618659994078,37.9608353507432,38.9598047020785,
39.9587740534139,40.9577434047492,41.9567127560846,42.7427228936713),
 .UNSPECIFIED.);
#811=B_SPLINE_CURVE_WITH_KNOTS('',3,(#50441,#50442,#50443,#50444,#50445,
#50446,#50447,#50448,#50449,#50450,#50451,#50452,#50453,#50454,#50455,#50456,
#50457,#50458,#50459,#50460,#50461,#50462,#50463,#50464,#50465),
 .UNSPECIFIED.,.F.,.F.,(4,3,3,3,3,3,3,3,4),(-52.0008580378518,-51.946406269438,
-50.9474369181027,-49.9484675667673,-48.949498215432,-47.9505288640967,
-46.9515595127613,-45.952590161426,-45.7176727306722),.UNSPECIFIED.);
#812=B_SPLINE_CURVE_WITH_KNOTS('',3,(#50466,#50467,#50468,#50469,#50470,
#50471,#50472,#50473,#50474,#50475,#50476,#50477,#50478,#50479,#50480,#50481,
#50482,#50483,#50484,#50485,#50486,#50487,#50488,#50489,#50490),
 .UNSPECIFIED.,.F.,.F.,(4,3,3,3,3,3,3,3,4),(42.7427228936713,42.9556821074199,
43.9546514587553,44.9536208100906,45.9525901614259,46.9515595127613,47.9505288640966,
48.949498215432,49.0259082008509),.UNSPECIFIED.);
#813=B_SPLINE_CURVE_WITH_KNOTS('',3,(#50495,#50496,#50497,#50498,#50499,
#50500,#50501,#50502,#50503,#50504,#50505,#50506,#50507,#50508,#50509,#50510,
#50511,#50512,#50513,#50514,#50515,#50516),.UNSPECIFIED.,.F.,.F.,(4,3,3,
3,3,3,3,4),(-58.2840433450314,-57.9402223774501,-56.9412530261148,-55.9422836747794,
-54.9433143234441,-53.9443449721087,-52.9453756207734,-52.0008580378518),
 .UNSPECIFIED.);
#814=B_SPLINE_CURVE_WITH_KNOTS('',3,(#50517,#50518,#50519,#50520,#50521,
#50522,#50523,#50524,#50525,#50526,#50527,#50528,#50529,#50530,#50531,#50532,
#50533,#50534,#50535,#50536,#50537,#50538),.UNSPECIFIED.,.F.,.F.,(4,3,3,
3,3,3,3,4),(49.0259082008509,49.9484675667673,50.9474369181027,51.946406269438,
52.9453756207734,53.9443449721087,54.9433143234441,55.3090935080305),
 .UNSPECIFIED.);
#815=B_SPLINE_CURVE_WITH_KNOTS('',3,(#50543,#50544,#50545,#50546,#50547,
#50548,#50549,#50550,#50551,#50552,#50553,#50554,#50555,#50556,#50557,#50558,
#50559,#50560,#50561,#50562,#50563,#50564),.UNSPECIFIED.,.F.,.F.,(4,3,3,
3,3,3,3,4),(-64.567228652211,-63.9340384854622,-62.9350691341269,-61.9360997827915,
-60.9371304314562,-59.9381610801208,-58.9391917287855,-58.2840433450314),
 .UNSPECIFIED.);
#816=B_SPLINE_CURVE_WITH_KNOTS('',3,(#50565,#50566,#50567,#50568,#50569,
#50570,#50571,#50572,#50573,#50574,#50575,#50576,#50577,#50578,#50579,#50580,
#50581,#50582,#50583,#50584,#50585,#50586),.UNSPECIFIED.,.F.,.F.,(4,3,3,
3,3,3,3,4),(55.3090935080305,55.9422836747794,56.9412530261148,57.9402223774501,
58.9391917287854,59.9381610801208,60.9371304314561,61.5922788152101),
 .UNSPECIFIED.);
#817=B_SPLINE_CURVE_WITH_KNOTS('',3,(#50591,#50592,#50593,#50594,#50595,
#50596,#50597,#50598,#50599,#50600,#50601,#50602,#50603,#50604,#50605,#50606,
#50607,#50608,#50609,#50610,#50611,#50612),.UNSPECIFIED.,.F.,.F.,(4,3,3,
3,3,3,3,4),(-70.8504139593906,-69.9278545934743,-68.9288852421389,-67.9299158908036,
-66.9309465394682,-65.9319771881329,-64.9330078367975,-64.567228652211),
 .UNSPECIFIED.);
#818=B_SPLINE_CURVE_WITH_KNOTS('',3,(#50613,#50614,#50615,#50616,#50617,
#50618,#50619,#50620,#50621,#50622,#50623,#50624,#50625,#50626,#50627,#50628,
#50629,#50630,#50631,#50632,#50633,#50634),.UNSPECIFIED.,.F.,.F.,(4,3,3,
3,3,3,3,4),(61.5922788152101,61.9360997827915,62.9350691341268,63.9340384854622,
64.9330078367975,65.9319771881329,66.9309465394682,67.8754641223897),
 .UNSPECIFIED.);
#819=B_SPLINE_CURVE_WITH_KNOTS('',3,(#50639,#50640,#50641,#50642,#50643,
#50644,#50645,#50646,#50647,#50648,#50649,#50650,#50651,#50652,#50653,#50654,
#50655,#50656,#50657,#50658,#50659,#50660,#50661,#50662,#50663),
 .UNSPECIFIED.,.F.,.F.,(4,3,3,3,3,3,3,3,4),(-77.1335992665702,-76.9206400528217,
-75.9216707014863,-74.922701350151,-73.9237319988157,-72.9247626474803,
-71.925793296145,-70.9268239448096,-70.8504139593906),.UNSPECIFIED.);
#820=B_SPLINE_CURVE_WITH_KNOTS('',3,(#50664,#50665,#50666,#50667,#50668,
#50669,#50670,#50671,#50672,#50673,#50674,#50675,#50676,#50677,#50678,#50679,
#50680,#50681,#50682,#50683,#50684,#50685,#50686,#50687,#50688),
 .UNSPECIFIED.,.F.,.F.,(4,3,3,3,3,3,3,3,4),(67.8754641223897,67.9299158908036,
68.9288852421389,69.9278545934743,70.9268239448096,71.9257932961449,72.9247626474803,
73.9237319988156,74.1586494295693),.UNSPECIFIED.);
#821=B_SPLINE_CURVE_WITH_KNOTS('',3,(#50693,#50694,#50695,#50696,#50697,
#50698,#50699,#50700,#50701,#50702,#50703,#50704,#50705,#50706,#50707,#50708,
#50709,#50710,#50711,#50712,#50713,#50714),.UNSPECIFIED.,.F.,.F.,(4,3,3,
3,3,3,3,4),(-83.4167845737498,-82.9144561608338,-81.9154868094984,-80.9165174581631,
-79.9175481068278,-78.9185787554924,-77.9196094041571,-77.1335992665702),
 .UNSPECIFIED.);
#822=B_SPLINE_CURVE_WITH_KNOTS('',3,(#50715,#50716,#50717,#50718,#50719,
#50720,#50721,#50722,#50723,#50724,#50725,#50726,#50727,#50728,#50729,#50730,
#50731,#50732,#50733,#50734,#50735,#50736),.UNSPECIFIED.,.F.,.F.,(4,3,3,
3,3,3,3,4),(74.1586494295693,74.922701350151,75.9216707014863,76.9206400528217,
77.919609404157,78.9185787554924,79.9175481068277,80.4418347367489),
 .UNSPECIFIED.);
#823=B_SPLINE_CURVE_WITH_KNOTS('',3,(#50741,#50742,#50743,#50744,#50745,
#50746,#50747,#50748,#50749,#50750,#50751,#50752,#50753,#50754,#50755,#50756,
#50757,#50758,#50759,#50760,#50761,#50762),.UNSPECIFIED.,.F.,.F.,(4,3,3,
3,3,3,3,4),(-89.6999698809294,-88.9082722688459,-87.9093029175105,-86.9103335661752,
-85.9113642148398,-84.9123948635045,-83.9134255121691,-83.4167845737498),
 .UNSPECIFIED.);
#824=B_SPLINE_CURVE_WITH_KNOTS('',3,(#50763,#50764,#50765,#50766,#50767,
#50768,#50769,#50770,#50771,#50772,#50773,#50774,#50775,#50776,#50777,#50778,
#50779,#50780,#50781,#50782,#50783,#50784),.UNSPECIFIED.,.F.,.F.,(4,3,3,
3,3,3,3,4),(80.4418347367489,80.9165174581631,81.9154868094984,82.9144561608338,
83.9134255121691,84.9123948635045,85.9113642148398,86.7250200439285),
 .UNSPECIFIED.);
#825=B_SPLINE_CURVE_WITH_KNOTS('',3,(#50789,#50790,#50791,#50792,#50793,
#50794,#50795,#50796,#50797,#50798,#50799,#50800,#50801,#50802,#50803,#50804,
#50805,#50806,#50807,#50808,#50809,#50810,#50811,#50812,#50813),
 .UNSPECIFIED.,.F.,.F.,(4,3,3,3,3,3,3,3,4),(-95.983155188109,-95.9010577281933,
-94.902088376858,-93.9031190255226,-92.9041496741873,-91.9051803228519,
-90.9062109715166,-89.9072416201812,-89.6999698809294),.UNSPECIFIED.);
#826=B_SPLINE_CURVE_WITH_KNOTS('',3,(#50814,#50815,#50816,#50817,#50818,
#50819,#50820,#50821,#50822,#50823,#50824,#50825,#50826,#50827,#50828,#50829,
#50830,#50831,#50832,#50833,#50834,#50835,#50836,#50837,#50838),
 .UNSPECIFIED.,.F.,.F.,(4,3,3,3,3,3,3,3,4),(86.7250200439285,86.9103335661752,
87.9093029175105,88.9082722688459,89.9072416201812,90.9062109715166,91.9051803228519,
92.9041496741873,93.0082053511081),.UNSPECIFIED.);
#827=B_SPLINE_CURVE_WITH_KNOTS('',3,(#50843,#50844,#50845,#50846,#50847,
#50848,#50849,#50850,#50851,#50852,#50853,#50854,#50855,#50856,#50857,#50858,
#50859,#50860,#50861,#50862,#50863,#50864),.UNSPECIFIED.,.F.,.F.,(4,3,3,
3,3,3,3,4),(-102.266340495289,-101.894873836205,-100.89590448487,-99.8969351335347,
-98.8979657821993,-97.898996430864,-96.9000270795287,-95.983155188109),
 .UNSPECIFIED.);
#828=B_SPLINE_CURVE_WITH_KNOTS('',3,(#50865,#50866,#50867,#50868,#50869,
#50870,#50871,#50872,#50873,#50874,#50875,#50876,#50877,#50878,#50879,#50880,
#50881,#50882,#50883,#50884,#50885,#50886),.UNSPECIFIED.,.F.,.F.,(4,3,3,
3,3,3,3,4),(93.0082053511081,93.9031190255226,94.9020883768579,95.9010577281933,
96.9000270795286,97.8989964308639,98.8979657821993,99.2913906582877),
 .UNSPECIFIED.);
#829=B_SPLINE_CURVE_WITH_KNOTS('',3,(#50891,#50892,#50893,#50894,#50895,
#50896,#50897,#50898,#50899,#50900,#50901,#50902,#50903,#50904,#50905,#50906,
#50907,#50908,#50909,#50910,#50911,#50912),.UNSPECIFIED.,.F.,.F.,(4,3,3,
3,3,3,3,4),(-108.549525802468,-107.888689944217,-106.889720592882,-105.890751241547,
-104.891781890211,-103.892812538876,-102.893843187541,-102.266340495289),
 .UNSPECIFIED.);
#830=B_SPLINE_CURVE_WITH_KNOTS('',3,(#50913,#50914,#50915,#50916,#50917,
#50918,#50919,#50920,#50921,#50922,#50923,#50924,#50925,#50926,#50927,#50928,
#50929,#50930,#50931,#50932,#50933,#50934),.UNSPECIFIED.,.F.,.F.,(4,3,3,
3,3,3,3,4),(99.2913906582877,99.8969351335346,100.89590448487,101.894873836205,
102.893843187541,103.892812538876,104.891781890211,105.574575965467),
 .UNSPECIFIED.);
#831=B_SPLINE_CURVE_WITH_KNOTS('',3,(#50939,#50940,#50941,#50942,#50943,
#50944,#50945,#50946,#50947,#50948,#50949,#50950,#50951,#50952,#50953,#50954,
#50955,#50956,#50957,#50958,#50959,#50960),.UNSPECIFIED.,.F.,.F.,(4,3,3,
3,3,3,3,4),(-114.832711109648,-113.88250605223,-112.883536700894,-111.884567349559,
-110.885597998224,-109.886628646888,-108.887659295553,-108.549525802468),
 .UNSPECIFIED.);
#832=B_SPLINE_CURVE_WITH_KNOTS('',3,(#50961,#50962,#50963,#50964,#50965,
#50966,#50967,#50968,#50969,#50970,#50971,#50972,#50973,#50974,#50975,#50976,
#50977,#50978,#50979,#50980,#50981,#50982),.UNSPECIFIED.,.F.,.F.,(4,3,3,
3,3,3,3,4),(105.574575965467,105.890751241547,106.889720592882,107.888689944217,
108.887659295553,109.886628646888,110.885597998223,111.857761272647),
 .UNSPECIFIED.);
#833=B_SPLINE_CURVE_WITH_KNOTS('',3,(#50988,#50989,#50990,#50991,#50992,
#50993,#50994),.UNSPECIFIED.,.F.,.F.,(4,1,1,1,4),(128.805298797182,128.854063091099,
129.853032442434,130.852001793769,131.782312197151),.UNSPECIFIED.);
#834=B_SPLINE_CURVE_WITH_KNOTS('',3,(#50997,#50998,#50999,#51000,#51001),
 .UNSPECIFIED.,.F.,.F.,(4,1,4),(128.805298797182,129.541705026261,130.540674377597),
 .UNSPECIFIED.);
#835=B_SPLINE_CURVE_WITH_KNOTS('',3,(#51006,#51007,#51008,#51009,#51010,
#51011,#51012,#51013,#51014,#51015),.UNSPECIFIED.,.F.,.F.,(4,1,1,1,1,1,
1,4),(122.522113490002,122.860246983087,123.859216334422,124.858185685757,
125.857155037093,126.856124388428,127.855093739763,128.805298797182),
 .UNSPECIFIED.);
#836=B_SPLINE_CURVE_WITH_KNOTS('',3,(#51016,#51017,#51018,#51019,#51020,
#51021,#51022,#51023,#51024,#51025,#51026),.UNSPECIFIED.,.F.,.F.,(4,1,1,
1,1,1,1,1,4),(122.522113490002,122.548919566914,123.547888918249,124.546858269584,
125.54582762092,126.544796972255,127.54376632359,128.542735674926,128.805298797182),
 .UNSPECIFIED.);
#837=B_SPLINE_CURVE_WITH_KNOTS('',3,(#51031,#51032,#51033,#51034,#51035,
#51036,#51037,#51038,#51039,#51040),.UNSPECIFIED.,.F.,.F.,(4,1,1,1,1,1,
1,4),(116.238928182822,116.866430875074,117.86540022641,118.864369577745,
119.863338929081,120.862308280416,121.861277631751,122.522113490002),
 .UNSPECIFIED.);
#838=B_SPLINE_CURVE_WITH_KNOTS('',3,(#51041,#51042,#51043,#51044,#51045,
#51046,#51047,#51048,#51049,#51050),.UNSPECIFIED.,.F.,.F.,(4,1,1,1,1,1,
1,4),(116.238928182822,116.555103458902,117.554072810237,118.553042161572,
119.552011512908,120.550980864243,121.549950215578,122.522113490002),
 .UNSPECIFIED.);
#839=B_SPLINE_CURVE_WITH_KNOTS('',3,(#51055,#51056,#51057,#51058,#51059,
#51060,#51061,#51062,#51063,#51064),.UNSPECIFIED.,.F.,.F.,(4,1,1,1,1,1,
1,4),(109.955742875643,110.872614767062,111.871584118398,112.870553469733,
113.869522821068,114.868492172404,115.867461523739,116.238928182822),
 .UNSPECIFIED.);
#840=B_SPLINE_CURVE_WITH_KNOTS('',3,(#51065,#51066,#51067,#51068,#51069,
#51070,#51071,#51072,#51073,#51074),.UNSPECIFIED.,.F.,.F.,(4,1,1,1,1,1,
1,4),(109.955742875643,110.56128735089,111.560256702225,112.55922605356,
113.558195404896,114.557164756231,115.556134107566,116.238928182822),
 .UNSPECIFIED.);
#841=B_SPLINE_CURVE_WITH_KNOTS('',3,(#51079,#51080,#51081,#51082,#51083,
#51084,#51085,#51086,#51087,#51088,#51089),.UNSPECIFIED.,.F.,.F.,(4,1,1,
1,1,1,1,1,4),(103.672557568463,103.879829307715,104.87879865905,105.877768010386,
106.876737361721,107.875706713056,108.874676064392,109.873645415727,109.955742875643),
 .UNSPECIFIED.);
#842=B_SPLINE_CURVE_WITH_KNOTS('',3,(#51090,#51091,#51092,#51093,#51094,
#51095,#51096,#51097,#51098,#51099),.UNSPECIFIED.,.F.,.F.,(4,1,1,1,1,1,
1,4),(103.672557568463,104.567471242878,105.566440594213,106.565409945548,
107.564379296884,108.563348648219,109.562317999554,109.955742875643),
 .UNSPECIFIED.);
#843=B_SPLINE_CURVE_WITH_KNOTS('',3,(#51104,#51105,#51106,#51107,#51108,
#51109,#51110,#51111,#51112,#51113),.UNSPECIFIED.,.F.,.F.,(4,1,1,1,1,1,
1,4),(97.3893722612835,97.8860131997029,98.8849825510382,99.8839519023736,
100.882921253709,101.881890605044,102.88085995638,103.672557568463),
 .UNSPECIFIED.);
#844=B_SPLINE_CURVE_WITH_KNOTS('',3,(#51114,#51115,#51116,#51117,#51118,
#51119,#51120,#51121,#51122,#51123,#51124),.UNSPECIFIED.,.F.,.F.,(4,1,1,
1,1,1,1,1,4),(97.3893722612835,97.5746857835301,98.5736551348654,99.5726244862008,
100.571593837536,101.570563188871,102.569532540207,103.568501891542,103.672557568463),
 .UNSPECIFIED.);
#845=B_SPLINE_CURVE_WITH_KNOTS('',3,(#51129,#51130,#51131,#51132,#51133,
#51134,#51135,#51136,#51137,#51138),.UNSPECIFIED.,.F.,.F.,(4,1,1,1,1,1,
1,4),(91.106186954104,91.8921970916908,92.8911664430261,93.8901357943615,
94.8891051456968,95.8880744970322,96.8870438483675,97.3893722612835),
 .UNSPECIFIED.);
#846=B_SPLINE_CURVE_WITH_KNOTS('',3,(#51139,#51140,#51141,#51142,#51143,
#51144,#51145,#51146,#51147,#51148),.UNSPECIFIED.,.F.,.F.,(4,1,1,1,1,1,
1,4),(91.1061869541039,91.580869675518,92.5798390268534,93.5788083781887,
94.5777777295241,95.5767470808594,96.5757164321948,97.3893722612835),
 .UNSPECIFIED.);
#847=B_SPLINE_CURVE_WITH_KNOTS('',3,(#51153,#51154,#51155,#51156,#51157,
#51158,#51159,#51160,#51161,#51162,#51163),.UNSPECIFIED.,.F.,.F.,(4,1,1,
1,1,1,1,1,4),(84.8230016469244,84.8994116323434,85.8983809836787,86.8973503350141,
87.8963196863494,88.8952890376847,89.8942583890201,90.8932277403554,91.106186954104),
 .UNSPECIFIED.);
#848=B_SPLINE_CURVE_WITH_KNOTS('',3,(#51164,#51165,#51166,#51167,#51168,
#51169,#51170,#51171,#51172,#51173),.UNSPECIFIED.,.F.,.F.,(4,1,1,1,1,1,
1,4),(84.8230016469243,85.5870535675059,86.5860229188413,87.5849922701766,
88.583961621512,89.5829309728473,90.5819003241827,91.1061869541039),
 .UNSPECIFIED.);
#849=B_SPLINE_CURVE_WITH_KNOTS('',3,(#51178,#51179,#51180,#51181,#51182,
#51183,#51184,#51185,#51186,#51187),.UNSPECIFIED.,.F.,.F.,(4,1,1,1,1,1,
1,4),(78.5398163397448,78.9055955243313,79.9045648756666,80.903534227002,
81.9025035783373,82.9014729296727,83.900442281008,84.8230016469244),
 .UNSPECIFIED.);
#850=B_SPLINE_CURVE_WITH_KNOTS('',3,(#51188,#51189,#51190,#51191,#51192,
#51193,#51194,#51195,#51196,#51197,#51198),.UNSPECIFIED.,.F.,.F.,(4,1,1,
1,1,1,1,1,4),(78.5398163397448,78.5942681081585,79.5932374594938,80.5922068108292,
81.5911761621645,82.5901455134999,83.5891148648352,84.5880842161706,84.8230016469243),
 .UNSPECIFIED.);
#851=B_SPLINE_CURVE_WITH_KNOTS('',3,(#51203,#51204,#51205,#51206,#51207,
#51208,#51209,#51210,#51211,#51212),.UNSPECIFIED.,.F.,.F.,(4,1,1,1,1,1,
1,4),(72.2566310325652,72.9117794163192,73.9107487676546,74.9097181189899,
75.9086874703252,76.9076568216606,77.9066261729959,78.5398163397448),
 .UNSPECIFIED.);
#852=B_SPLINE_CURVE_WITH_KNOTS('',3,(#51213,#51214,#51215,#51216,#51217,
#51218,#51219,#51220,#51221,#51222),.UNSPECIFIED.,.F.,.F.,(4,1,1,1,1,1,
1,4),(72.2566310325652,72.6004520001464,73.5994213514818,74.5983907028171,
75.5973600541525,76.5963294054878,77.5952987568232,78.5398163397448),
 .UNSPECIFIED.);
#853=B_SPLINE_CURVE_WITH_KNOTS('',3,(#51227,#51228,#51229,#51230,#51231,
#51232,#51233,#51234,#51235,#51236),.UNSPECIFIED.,.F.,.F.,(4,1,1,1,1,1,
1,4),(65.9734457253856,66.9179633083071,67.9169326596425,68.9159020109778,
69.9148713623132,70.9138407136485,71.9128100649839,72.2566310325652),
 .UNSPECIFIED.);
#854=B_SPLINE_CURVE_WITH_KNOTS('',3,(#51237,#51238,#51239,#51240,#51241,
#51242,#51243,#51244,#51245,#51246),.UNSPECIFIED.,.F.,.F.,(4,1,1,1,1,1,
1,4),(65.9734457253856,66.6066358921343,67.6056052434697,68.604574594805,
69.6035439461404,70.6025132974757,71.6014826488111,72.2566310325652),
 .UNSPECIFIED.);
#855=B_SPLINE_CURVE_WITH_KNOTS('',3,(#51251,#51252,#51253,#51254,#51255,
#51256,#51257,#51258,#51259,#51260,#51261),.UNSPECIFIED.,.F.,.F.,(4,1,1,
1,1,1,1,1,4),(59.690260418206,59.9251778489597,60.924147200295,61.9231165516304,
62.9220859029657,63.9210552543011,64.9200246056364,65.9189939569718,65.9734457253856),
 .UNSPECIFIED.);
#856=B_SPLINE_CURVE_WITH_KNOTS('',3,(#51262,#51263,#51264,#51265,#51266,
#51267,#51268,#51269,#51270,#51271),.UNSPECIFIED.,.F.,.F.,(4,1,1,1,1,1,
1,4),(59.690260418206,60.6128197841223,61.6117891354576,62.610758486793,
63.6097278381283,64.6086971894637,65.607666540799,65.9734457253856),
 .UNSPECIFIED.);
#857=B_SPLINE_CURVE_WITH_KNOTS('',3,(#51276,#51277,#51278,#51279,#51280,
#51281,#51282,#51283,#51284,#51285),.UNSPECIFIED.,.F.,.F.,(4,1,1,1,1,1,
1,4),(53.4070751110264,53.9313617409476,54.930331092283,55.9293004436183,
56.9282697949536,57.927239146289,58.9262084976243,59.690260418206),
 .UNSPECIFIED.);
#858=B_SPLINE_CURVE_WITH_KNOTS('',3,(#51286,#51287,#51288,#51289,#51290,
#51291,#51292,#51293,#51294,#51295,#51296),.UNSPECIFIED.,.F.,.F.,(4,1,1,
1,1,1,1,1,4),(53.4070751110264,53.6200343247748,54.6190036761102,55.6179730274455,
56.6169423787809,57.6159117301162,58.6148810814516,59.6138504327869,59.690260418206),
 .UNSPECIFIED.);
#859=B_SPLINE_CURVE_WITH_KNOTS('',3,(#51301,#51302,#51303,#51304,#51305,
#51306,#51307,#51308,#51309,#51310),.UNSPECIFIED.,.F.,.F.,(4,1,1,1,1,1,
1,4),(47.1238898038468,47.9375456329355,48.9365149842709,49.9354843356062,
50.9344536869416,51.9334230382769,52.9323923896123,53.4070751110264),
 .UNSPECIFIED.);
#860=B_SPLINE_CURVE_WITH_KNOTS('',3,(#51311,#51312,#51313,#51314,#51315,
#51316,#51317,#51318,#51319,#51320),.UNSPECIFIED.,.F.,.F.,(4,1,1,1,1,1,
1,4),(47.1238898038468,47.6262182167628,48.6251875680981,49.6241569194335,
50.6231262707688,51.6220956221041,52.6210649734395,53.4070751110264),
 .UNSPECIFIED.);
#861=B_SPLINE_CURVE_WITH_KNOTS('',3,(#51325,#51326,#51327,#51328,#51329,
#51330,#51331,#51332,#51333,#51334,#51335),.UNSPECIFIED.,.F.,.F.,(4,1,1,
1,1,1,1,1,4),(40.8407044966672,40.9447601735881,41.9437295249234,42.9426988762588,
43.9416682275941,44.9406375789295,45.9396069302648,46.9385762816002,47.1238898038468),
 .UNSPECIFIED.);
#862=B_SPLINE_CURVE_WITH_KNOTS('',3,(#51336,#51337,#51338,#51339,#51340,
#51341,#51342,#51343,#51344,#51345),.UNSPECIFIED.,.F.,.F.,(4,1,1,1,1,1,
1,4),(40.8407044966672,41.6324021087507,42.631371460086,43.6303408114214,
44.6293101627567,45.6282795140921,46.6272488654274,47.1238898038468),
 .UNSPECIFIED.);
#863=B_SPLINE_CURVE_WITH_KNOTS('',3,(#51350,#51351,#51352,#51353,#51354,
#51355,#51356,#51357,#51358,#51359),.UNSPECIFIED.,.F.,.F.,(4,1,1,1,1,1,
1,4),(34.5575191894876,34.950944065576,35.9499134169114,36.9488827682467,
37.9478521195821,38.9468214709174,39.9457908222528,40.8407044966672),
 .UNSPECIFIED.);
#864=B_SPLINE_CURVE_WITH_KNOTS('',3,(#51360,#51361,#51362,#51363,#51364,
#51365,#51366,#51367,#51368,#51369,#51370),.UNSPECIFIED.,.F.,.F.,(4,1,1,
1,1,1,1,1,4),(34.5575191894876,34.6396166494033,35.6385860007386,36.6375553520739,
37.6365247034093,38.6354940547446,39.63446340608,40.6334327574153,40.8407044966672),
 .UNSPECIFIED.);
#865=B_SPLINE_CURVE_WITH_KNOTS('',3,(#51375,#51376,#51377,#51378,#51379,
#51380,#51381,#51382,#51383,#51384),.UNSPECIFIED.,.F.,.F.,(4,1,1,1,1,1,
1,4),(28.2743338823081,28.9571279575639,29.9560973088993,30.9550666602346,
31.95403601157,32.9530053629053,33.9519747142407,34.5575191894876),
 .UNSPECIFIED.);
#866=B_SPLINE_CURVE_WITH_KNOTS('',3,(#51385,#51386,#51387,#51388,#51389,
#51390,#51391,#51392,#51393,#51394),.UNSPECIFIED.,.F.,.F.,(4,1,1,1,1,1,
1,4),(28.274333882308,28.6458005413912,29.6447698927265,30.6437392440619,
31.6427085953972,32.6416779467326,33.6406472980679,34.5575191894876),
 .UNSPECIFIED.);
#867=B_SPLINE_CURVE_WITH_KNOTS('',3,(#51399,#51400,#51401,#51402,#51403,
#51404,#51405,#51406,#51407,#51408),.UNSPECIFIED.,.F.,.F.,(4,1,1,1,1,1,
1,4),(21.9911485751285,22.9633118495519,23.9622812008872,24.9612505522226,
25.9602199035579,26.9591892548932,27.9581586062286,28.2743338823081),
 .UNSPECIFIED.);
#868=B_SPLINE_CURVE_WITH_KNOTS('',3,(#51409,#51410,#51411,#51412,#51413,
#51414,#51415,#51416,#51417,#51418),.UNSPECIFIED.,.F.,.F.,(4,1,1,1,1,1,
1,4),(21.9911485751284,22.6519844333791,23.6509537847144,24.6499231360498,
25.6488924873851,26.6478618387205,27.6468311900558,28.274333882308),
 .UNSPECIFIED.);
#869=B_SPLINE_CURVE_WITH_KNOTS('',3,(#51423,#51424,#51425,#51426,#51427,
#51428,#51429,#51430,#51431,#51432,#51433),.UNSPECIFIED.,.F.,.F.,(4,1,1,
1,1,1,1,1,4),(15.7079632679489,15.9705263902044,16.9694957415398,17.9684650928751,
18.9674344442105,19.9664037955458,20.9653731468812,21.9643424982165,21.9911485751285),
 .UNSPECIFIED.);
#870=B_SPLINE_CURVE_WITH_KNOTS('',3,(#51434,#51435,#51436,#51437,#51438,
#51439,#51440,#51441,#51442,#51443),.UNSPECIFIED.,.F.,.F.,(4,1,1,1,1,1,
1,4),(15.7079632679489,16.658168325367,17.6571376767024,18.6561070280377,
19.6550763793731,20.6540457307084,21.6530150820438,21.9911485751284),
 .UNSPECIFIED.);
#871=B_SPLINE_CURVE_WITH_KNOTS('',3,(#51446,#51447,#51448,#51449,#51450,
#51451,#51452,#51453,#51454,#51455,#51456,#51457,#51458,#51459,#51460,#51461,
#51462,#51463,#51464,#51465,#51466,#51467,#51468,#51469,#51470,#51471,#51472,
#51473,#51474,#51475,#51476,#51477,#51478,#51479,#51480,#51481,#51482,#51483,
#51484,#51485,#51486,#51487,#51488,#51489,#51490,#51491,#51492,#51493,#51494,
#51495,#51496,#51497,#51498,#51499,#51500,#51501,#51502,#51503),
 .UNSPECIFIED.,.F.,.F.,(4,3,3,3,3,3,3,3,3,3,3,3,3,3,3,3,3,3,3,4),(-0.463803050843755,
-0.449907398794694,-0.418031857702381,-0.400337768208314,-0.372896888686324,
-0.358221213465045,-0.345421670140428,-0.303252356142987,-0.273478234693713,
-0.262474993370258,-0.235827691279064,-0.206349229869181,-0.190332836617136,
-0.175380554584644,-0.131535415938483,-0.108450622298565,-0.0944456675460115,
-0.0816634290814505,-0.0359771892759535,0.),.UNSPECIFIED.);
#872=B_SPLINE_CURVE_WITH_KNOTS('',3,(#51508,#51509,#51510,#51511,#51512,
#51513,#51514,#51515,#51516,#51517,#51518,#51519,#51520,#51521,#51522,#51523,
#51524,#51525,#51526,#51527,#51528,#51529,#51530,#51531,#51532,#51533,#51534,
#51535,#51536,#51537,#51538,#51539,#51540,#51541,#51542,#51543,#51544,#51545,
#51546,#51547,#51548,#51549,#51550,#51551,#51552,#51553,#51554,#51555,#51556,
#51557,#51558,#51559,#51560,#51561,#51562,#51563,#51564,#51565),
 .UNSPECIFIED.,.F.,.F.,(4,3,3,3,3,3,3,3,3,3,3,3,3,3,3,3,3,3,3,4),(-0.461788964899843,
-0.444996338453757,-0.413305262598462,-0.398720954647667,-0.383442254293799,
-0.356179300230217,-0.336984284953546,-0.32270401518387,-0.279139696516272,
-0.260144406012141,-0.247531499300344,-0.235347705780398,-0.211863769192623,
-0.169080986415294,-0.153240163194338,-0.114930122395753,-0.0804234717365801,
-0.0679412143129863,-0.0289558983189821,0.),.UNSPECIFIED.);
#873=B_SPLINE_CURVE_WITH_KNOTS('',3,(#52058,#52059,#52060,#52061,#52062,
#52063,#52064,#52065,#52066,#52067,#52068,#52069,#52070,#52071,#52072,#52073,
#52074,#52075,#52076,#52077,#52078,#52079),.UNSPECIFIED.,.F.,.F.,(4,3,3,
3,3,3,3,4),(111.857761272647,111.884567349559,112.883536700894,113.88250605223,
114.881475403565,115.8804447549,116.879414106236,117.809724509617),
 .UNSPECIFIED.);
#874=B_SPLINE_CURVE_WITH_KNOTS('',3,(#52081,#52082,#52083,#52084,#52085,
#52086,#52087,#52088,#52089,#52090,#52091,#52092,#52093,#52094,#52095,#52096,
#52097,#52098,#52099,#52100,#52101,#52102,#52103,#52104,#52105,#52106,#52107,
#52108,#52109,#52110,#52111,#52112,#52113,#52114,#52115,#52116,#52117,#52118,
#52119,#52120,#52121,#52122,#52123,#52124,#52125,#52126,#52127,#52128,#52129,
#52130,#52131,#52132,#52133,#52134,#52135,#52136,#52137,#52138),
 .UNSPECIFIED.,.F.,.F.,(4,3,3,3,3,3,3,3,3,3,3,3,3,3,3,3,3,3,3,4),(-0.46380305084371,
-0.449907398794639,-0.418031858716818,-0.400337770850382,-0.372897098979116,
-0.358225636990301,-0.345427365771652,-0.303258135833885,-0.273481221790439,
-0.262481185322834,-0.235827691279055,-0.206349229869174,-0.190332831578201,
-0.175380551365677,-0.131535413524257,-0.108450616220395,-0.09444564303348,
-0.0816634226200209,-0.0359771748293766,0.),.UNSPECIFIED.);
#875=B_SPLINE_CURVE_WITH_KNOTS('',3,(#52139,#52140,#52141,#52142,#52143,
#52144,#52145),.UNSPECIFIED.,.F.,.F.,(4,1,1,1,4),(12.7309498679793,13.661260271361,
14.6602296226963,15.6591989740317,15.7079632679489),.UNSPECIFIED.);
#876=B_SPLINE_CURVE_WITH_KNOTS('',3,(#52148,#52149,#52150,#52151,#52152,
#52153,#52154,#52155,#52156,#52157,#52158,#52159,#52160,#52161,#52162,#52163,
#52164,#52165,#52166,#52167,#52168,#52169,#52170,#52171,#52172,#52173,#52174,
#52175,#52176,#52177,#52178,#52179,#52180,#52181,#52182,#52183,#52184,#52185,
#52186,#52187,#52188,#52189,#52190,#52191,#52192,#52193,#52194,#52195,#52196,
#52197,#52198,#52199,#52200,#52201,#52202,#52203,#52204,#52205),
 .UNSPECIFIED.,.F.,.F.,(4,3,3,3,3,3,3,3,3,3,3,3,3,3,3,3,3,3,3,4),(-0.461788964899765,
-0.444996338453673,-0.413305257846947,-0.398720941271075,-0.38344224790616,
-0.356179268364253,-0.33698399566128,-0.32270394349123,-0.279139618915834,
-0.260144344795765,-0.247531524843875,-0.235347708885629,-0.211863769192592,
-0.16908098381302,-0.153240164163327,-0.114930123122496,-0.08042347380898,
-0.0679412157174702,-0.028955921834972,0.),.UNSPECIFIED.);
#877=B_SPLINE_CURVE_WITH_KNOTS('',3,(#52208,#52209,#52210,#52211,#52212),
 .UNSPECIFIED.,.F.,.F.,(4,1,4),(13.9725876875337,14.9715570388691,15.7079632679489),
 .UNSPECIFIED.);
#878=B_SPLINE_CURVE_WITH_KNOTS('',3,(#52705,#52706,#52707,#52708,#52709,
#52710,#52711,#52712,#52713,#52714,#52715,#52716,#52717,#52718,#52719,#52720,
#52721,#52722,#52723),.UNSPECIFIED.,.F.,.F.,(4,3,3,3,3,3,4),(-119.876322160242,
-118.877352808906,-117.878383457571,-116.879414106236,-115.8804447549,-114.881475403565,
-114.832711109648),.UNSPECIFIED.);
#894=SHAPE_REPRESENTATION_RELATIONSHIP('SRR','None',#53739,#910);
#910=ADVANCED_BREP_SHAPE_REPRESENTATION('',(#942),#53649);
#926=STYLED_ITEM('',(#53965),#942);
#942=MANIFOLD_SOLID_BREP('ISO_4762_M5x16_A2',#23318);
#1237=CYLINDRICAL_SURFACE('',#25370,0.24505);
#1238=CYLINDRICAL_SURFACE('',#25374,0.24505);
#1239=CYLINDRICAL_SURFACE('',#25375,0.24505);
#1240=CYLINDRICAL_SURFACE('',#25376,0.24505);
#1241=CYLINDRICAL_SURFACE('',#25377,0.24505);
#1242=CYLINDRICAL_SURFACE('',#25378,0.24505);
#1243=CYLINDRICAL_SURFACE('',#25379,0.24505);
#1244=CYLINDRICAL_SURFACE('',#25380,0.24505);
#1245=CYLINDRICAL_SURFACE('',#25381,0.24505);
#1246=CYLINDRICAL_SURFACE('',#25382,0.24505);
#1247=CYLINDRICAL_SURFACE('',#25383,0.24505);
#1248=CYLINDRICAL_SURFACE('',#25384,0.24505);
#1249=CYLINDRICAL_SURFACE('',#25385,0.24505);
#1250=CYLINDRICAL_SURFACE('',#25386,0.24505);
#1251=CYLINDRICAL_SURFACE('',#25387,0.24505);
#1252=CYLINDRICAL_SURFACE('',#25388,0.24505);
#1253=CYLINDRICAL_SURFACE('',#25389,0.24505);
#1254=CYLINDRICAL_SURFACE('',#25390,0.24505);
#1255=CYLINDRICAL_SURFACE('',#25391,0.199475);
#1256=CYLINDRICAL_SURFACE('',#25393,0.199475);
#1257=CYLINDRICAL_SURFACE('',#25394,0.199475);
#1258=CYLINDRICAL_SURFACE('',#25395,0.199475);
#1259=CYLINDRICAL_SURFACE('',#25396,0.199475);
#1260=CYLINDRICAL_SURFACE('',#25397,0.199475);
#1261=CYLINDRICAL_SURFACE('',#25398,0.199475);
#1262=CYLINDRICAL_SURFACE('',#25399,0.199475);
#1263=CYLINDRICAL_SURFACE('',#25400,0.199475);
#1264=CYLINDRICAL_SURFACE('',#25401,0.199475);
#1265=CYLINDRICAL_SURFACE('',#25402,0.199475);
#1266=CYLINDRICAL_SURFACE('',#25403,0.199475);
#1267=CYLINDRICAL_SURFACE('',#25404,0.199475);
#1268=CYLINDRICAL_SURFACE('',#25405,0.199475);
#1269=CYLINDRICAL_SURFACE('',#25406,0.199475);
#1270=CYLINDRICAL_SURFACE('',#25407,0.199475);
#1271=CYLINDRICAL_SURFACE('',#25408,0.199475);
#1272=CYLINDRICAL_SURFACE('',#25409,0.199475);
#1273=CYLINDRICAL_SURFACE('',#25410,0.199475);
#1274=CYLINDRICAL_SURFACE('',#25416,0.199475);
#1275=CYLINDRICAL_SURFACE('',#25558,0.425);
#1276=CYLINDRICAL_SURFACE('',#25614,0.24505);
#1445=FACE_BOUND('',#5054,.T.);
#1446=FACE_BOUND('',#5060,.T.);
#1447=FACE_BOUND('',#5062,.T.);
#2116=PLANE('',#25411);
#2117=PLANE('',#25414);
#2118=PLANE('',#25417);
#2119=PLANE('',#25419);
#2120=PLANE('',#25420);
#2121=PLANE('',#25421);
#2122=PLANE('',#25423);
#2123=PLANE('',#25424);
#2124=PLANE('',#25425);
#2125=PLANE('',#25427);
#2126=PLANE('',#25428);
#2127=PLANE('',#25429);
#2128=PLANE('',#25431);
#2129=PLANE('',#25432);
#2130=PLANE('',#25433);
#2131=PLANE('',#25435);
#2132=PLANE('',#25436);
#2133=PLANE('',#25437);
#2134=PLANE('',#25439);
#2135=PLANE('',#25440);
#2136=PLANE('',#25441);
#2137=PLANE('',#25443);
#2138=PLANE('',#25444);
#2139=PLANE('',#25445);
#2140=PLANE('',#25447);
#2141=PLANE('',#25448);
#2142=PLANE('',#25449);
#2143=PLANE('',#25451);
#2144=PLANE('',#25452);
#2145=PLANE('',#25453);
#2146=PLANE('',#25455);
#2147=PLANE('',#25456);
#2148=PLANE('',#25457);
#2149=PLANE('',#25459);
#2150=PLANE('',#25460);
#2151=PLANE('',#25461);
#2152=PLANE('',#25463);
#2153=PLANE('',#25464);
#2154=PLANE('',#25465);
#2155=PLANE('',#25467);
#2156=PLANE('',#25468);
#2157=PLANE('',#25469);
#2158=PLANE('',#25471);
#2159=PLANE('',#25472);
#2160=PLANE('',#25473);
#2161=PLANE('',#25475);
#2162=PLANE('',#25476);
#2163=PLANE('',#25477);
#2164=PLANE('',#25479);
#2165=PLANE('',#25480);
#2166=PLANE('',#25481);
#2167=PLANE('',#25483);
#2168=PLANE('',#25484);
#2169=PLANE('',#25485);
#2170=PLANE('',#25488);
#2171=PLANE('',#25489);
#2172=PLANE('',#25490);
#2173=PLANE('',#25492);
#2174=PLANE('',#25493);
#2175=PLANE('',#25494);
#2176=PLANE('',#25496);
#2177=PLANE('',#25497);
#2178=PLANE('',#25498);
#2179=PLANE('',#25500);
#2180=PLANE('',#25501);
#2181=PLANE('',#25502);
#2182=PLANE('',#25504);
#2183=PLANE('',#25505);
#2184=PLANE('',#25506);
#2185=PLANE('',#25508);
#2186=PLANE('',#25509);
#2187=PLANE('',#25510);
#2188=PLANE('',#25512);
#2189=PLANE('',#25513);
#2190=PLANE('',#25514);
#2191=PLANE('',#25516);
#2192=PLANE('',#25517);
#2193=PLANE('',#25518);
#2194=PLANE('',#25520);
#2195=PLANE('',#25521);
#2196=PLANE('',#25522);
#2197=PLANE('',#25524);
#2198=PLANE('',#25525);
#2199=PLANE('',#25526);
#2200=PLANE('',#25528);
#2201=PLANE('',#25529);
#2202=PLANE('',#25530);
#2203=PLANE('',#25532);
#2204=PLANE('',#25533);
#2205=PLANE('',#25534);
#2206=PLANE('',#25536);
#2207=PLANE('',#25537);
#2208=PLANE('',#25538);
#2209=PLANE('',#25540);
#2210=PLANE('',#25541);
#2211=PLANE('',#25542);
#2212=PLANE('',#25544);
#2213=PLANE('',#25545);
#2214=PLANE('',#25546);
#2215=PLANE('',#25548);
#2216=PLANE('',#25549);
#2217=PLANE('',#25550);
#2218=PLANE('',#25552);
#2219=PLANE('',#25553);
#2220=PLANE('',#25554);
#2221=PLANE('',#25556);
#2222=PLANE('',#25557);
#2223=PLANE('',#25597);
#2224=PLANE('',#25598);
#2225=PLANE('',#25599);
#2226=PLANE('',#25604);
#2227=PLANE('',#25605);
#2228=PLANE('',#25606);
#2229=PLANE('',#25607);
#2230=PLANE('',#25608);
#2231=PLANE('',#25609);
#2232=PLANE('',#25610);
#2233=PLANE('',#25611);
#2234=PLANE('',#25618);
#2235=PLANE('',#25619);
#3398=FACE_OUTER_BOUND('',#4894,.T.);
#3399=FACE_OUTER_BOUND('',#4895,.T.);
#3400=FACE_OUTER_BOUND('',#4896,.T.);
#3401=FACE_OUTER_BOUND('',#4897,.T.);
#3402=FACE_OUTER_BOUND('',#4898,.T.);
#3403=FACE_OUTER_BOUND('',#4899,.T.);
#3404=FACE_OUTER_BOUND('',#4900,.T.);
#3405=FACE_OUTER_BOUND('',#4901,.T.);
#3406=FACE_OUTER_BOUND('',#4902,.T.);
#3407=FACE_OUTER_BOUND('',#4903,.T.);
#3408=FACE_OUTER_BOUND('',#4904,.T.);
#3409=FACE_OUTER_BOUND('',#4905,.T.);
#3410=FACE_OUTER_BOUND('',#4906,.T.);
#3411=FACE_OUTER_BOUND('',#4907,.T.);
#3412=FACE_OUTER_BOUND('',#4908,.T.);
#3413=FACE_OUTER_BOUND('',#4909,.T.);
#3414=FACE_OUTER_BOUND('',#4910,.T.);
#3415=FACE_OUTER_BOUND('',#4911,.T.);
#3416=FACE_OUTER_BOUND('',#4912,.T.);
#3417=FACE_OUTER_BOUND('',#4913,.T.);
#3418=FACE_OUTER_BOUND('',#4914,.T.);
#3419=FACE_OUTER_BOUND('',#4915,.T.);
#3420=FACE_OUTER_BOUND('',#4916,.T.);
#3421=FACE_OUTER_BOUND('',#4917,.T.);
#3422=FACE_OUTER_BOUND('',#4918,.T.);
#3423=FACE_OUTER_BOUND('',#4919,.T.);
#3424=FACE_OUTER_BOUND('',#4920,.T.);
#3425=FACE_OUTER_BOUND('',#4921,.T.);
#3426=FACE_OUTER_BOUND('',#4922,.T.);
#3427=FACE_OUTER_BOUND('',#4923,.T.);
#3428=FACE_OUTER_BOUND('',#4924,.T.);
#3429=FACE_OUTER_BOUND('',#4925,.T.);
#3430=FACE_OUTER_BOUND('',#4926,.T.);
#3431=FACE_OUTER_BOUND('',#4927,.T.);
#3432=FACE_OUTER_BOUND('',#4928,.T.);
#3433=FACE_OUTER_BOUND('',#4929,.T.);
#3434=FACE_OUTER_BOUND('',#4930,.T.);
#3435=FACE_OUTER_BOUND('',#4931,.T.);
#3436=FACE_OUTER_BOUND('',#4932,.T.);
#3437=FACE_OUTER_BOUND('',#4933,.T.);
#3438=FACE_OUTER_BOUND('',#4934,.T.);
#3439=FACE_OUTER_BOUND('',#4935,.T.);
#3440=FACE_OUTER_BOUND('',#4936,.T.);
#3441=FACE_OUTER_BOUND('',#4937,.T.);
#3442=FACE_OUTER_BOUND('',#4938,.T.);
#3443=FACE_OUTER_BOUND('',#4939,.T.);
#3444=FACE_OUTER_BOUND('',#4940,.T.);
#3445=FACE_OUTER_BOUND('',#4941,.T.);
#3446=FACE_OUTER_BOUND('',#4942,.T.);
#3447=FACE_OUTER_BOUND('',#4943,.T.);
#3448=FACE_OUTER_BOUND('',#4944,.T.);
#3449=FACE_OUTER_BOUND('',#4945,.T.);
#3450=FACE_OUTER_BOUND('',#4946,.T.);
#3451=FACE_OUTER_BOUND('',#4947,.T.);
#3452=FACE_OUTER_BOUND('',#4948,.T.);
#3453=FACE_OUTER_BOUND('',#4949,.T.);
#3454=FACE_OUTER_BOUND('',#4950,.T.);
#3455=FACE_OUTER_BOUND('',#4951,.T.);
#3456=FACE_OUTER_BOUND('',#4952,.T.);
#3457=FACE_OUTER_BOUND('',#4953,.T.);
#3458=FACE_OUTER_BOUND('',#4954,.T.);
#3459=FACE_OUTER_BOUND('',#4955,.T.);
#3460=FACE_OUTER_BOUND('',#4956,.T.);
#3461=FACE_OUTER_BOUND('',#4957,.T.);
#3462=FACE_OUTER_BOUND('',#4958,.T.);
#3463=FACE_OUTER_BOUND('',#4959,.T.);
#3464=FACE_OUTER_BOUND('',#4960,.T.);
#3465=FACE_OUTER_BOUND('',#4961,.T.);
#3466=FACE_OUTER_BOUND('',#4962,.T.);
#3467=FACE_OUTER_BOUND('',#4963,.T.);
#3468=FACE_OUTER_BOUND('',#4964,.T.);
#3469=FACE_OUTER_BOUND('',#4965,.T.);
#3470=FACE_OUTER_BOUND('',#4966,.T.);
#3471=FACE_OUTER_BOUND('',#4967,.T.);
#3472=FACE_OUTER_BOUND('',#4968,.T.);
#3473=FACE_OUTER_BOUND('',#4969,.T.);
#3474=FACE_OUTER_BOUND('',#4970,.T.);
#3475=FACE_OUTER_BOUND('',#4971,.T.);
#3476=FACE_OUTER_BOUND('',#4972,.T.);
#3477=FACE_OUTER_BOUND('',#4973,.T.);
#3478=FACE_OUTER_BOUND('',#4974,.T.);
#3479=FACE_OUTER_BOUND('',#4975,.T.);
#3480=FACE_OUTER_BOUND('',#4976,.T.);
#3481=FACE_OUTER_BOUND('',#4977,.T.);
#3482=FACE_OUTER_BOUND('',#4978,.T.);
#3483=FACE_OUTER_BOUND('',#4979,.T.);
#3484=FACE_OUTER_BOUND('',#4980,.T.);
#3485=FACE_OUTER_BOUND('',#4981,.T.);
#3486=FACE_OUTER_BOUND('',#4982,.T.);
#3487=FACE_OUTER_BOUND('',#4983,.T.);
#3488=FACE_OUTER_BOUND('',#4984,.T.);
#3489=FACE_OUTER_BOUND('',#4985,.T.);
#3490=FACE_OUTER_BOUND('',#4986,.T.);
#3491=FACE_OUTER_BOUND('',#4987,.T.);
#3492=FACE_OUTER_BOUND('',#4988,.T.);
#3493=FACE_OUTER_BOUND('',#4989,.T.);
#3494=FACE_OUTER_BOUND('',#4990,.T.);
#3495=FACE_OUTER_BOUND('',#4991,.T.);
#3496=FACE_OUTER_BOUND('',#4992,.T.);
#3497=FACE_OUTER_BOUND('',#4993,.T.);
#3498=FACE_OUTER_BOUND('',#4994,.T.);
#3499=FACE_OUTER_BOUND('',#4995,.T.);
#3500=FACE_OUTER_BOUND('',#4996,.T.);
#3501=FACE_OUTER_BOUND('',#4997,.T.);
#3502=FACE_OUTER_BOUND('',#4998,.T.);
#3503=FACE_OUTER_BOUND('',#4999,.T.);
#3504=FACE_OUTER_BOUND('',#5000,.T.);
#3505=FACE_OUTER_BOUND('',#5001,.T.);
#3506=FACE_OUTER_BOUND('',#5002,.T.);
#3507=FACE_OUTER_BOUND('',#5003,.T.);
#3508=FACE_OUTER_BOUND('',#5004,.T.);
#3509=FACE_OUTER_BOUND('',#5005,.T.);
#3510=FACE_OUTER_BOUND('',#5006,.T.);
#3511=FACE_OUTER_BOUND('',#5007,.T.);
#3512=FACE_OUTER_BOUND('',#5008,.T.);
#3513=FACE_OUTER_BOUND('',#5009,.T.);
#3514=FACE_OUTER_BOUND('',#5010,.T.);
#3515=FACE_OUTER_BOUND('',#5011,.T.);
#3516=FACE_OUTER_BOUND('',#5012,.T.);
#3517=FACE_OUTER_BOUND('',#5013,.T.);
#3518=FACE_OUTER_BOUND('',#5014,.T.);
#3519=FACE_OUTER_BOUND('',#5015,.T.);
#3520=FACE_OUTER_BOUND('',#5016,.T.);
#3521=FACE_OUTER_BOUND('',#5017,.T.);
#3522=FACE_OUTER_BOUND('',#5018,.T.);
#3523=FACE_OUTER_BOUND('',#5019,.T.);
#3524=FACE_OUTER_BOUND('',#5020,.T.);
#3525=FACE_OUTER_BOUND('',#5021,.T.);
#3526=FACE_OUTER_BOUND('',#5022,.T.);
#3527=FACE_OUTER_BOUND('',#5023,.T.);
#3528=FACE_OUTER_BOUND('',#5024,.T.);
#3529=FACE_OUTER_BOUND('',#5025,.T.);
#3530=FACE_OUTER_BOUND('',#5026,.T.);
#3531=FACE_OUTER_BOUND('',#5027,.T.);
#3532=FACE_OUTER_BOUND('',#5028,.T.);
#3533=FACE_OUTER_BOUND('',#5029,.T.);
#3534=FACE_OUTER_BOUND('',#5030,.T.);
#3535=FACE_OUTER_BOUND('',#5031,.T.);
#3536=FACE_OUTER_BOUND('',#5032,.T.);
#3537=FACE_OUTER_BOUND('',#5033,.T.);
#3538=FACE_OUTER_BOUND('',#5034,.T.);
#3539=FACE_OUTER_BOUND('',#5035,.T.);
#3540=FACE_OUTER_BOUND('',#5036,.T.);
#3541=FACE_OUTER_BOUND('',#5037,.T.);
#3542=FACE_OUTER_BOUND('',#5038,.T.);
#3543=FACE_OUTER_BOUND('',#5039,.T.);
#3544=FACE_OUTER_BOUND('',#5040,.T.);
#3545=FACE_OUTER_BOUND('',#5041,.T.);
#3546=FACE_OUTER_BOUND('',#5042,.T.);
#3547=FACE_OUTER_BOUND('',#5043,.T.);
#3548=FACE_OUTER_BOUND('',#5044,.T.);
#3549=FACE_OUTER_BOUND('',#5045,.T.);
#3550=FACE_OUTER_BOUND('',#5046,.T.);
#3551=FACE_OUTER_BOUND('',#5047,.T.);
#3552=FACE_OUTER_BOUND('',#5048,.T.);
#3553=FACE_OUTER_BOUND('',#5049,.T.);
#3554=FACE_OUTER_BOUND('',#5050,.T.);
#3555=FACE_OUTER_BOUND('',#5051,.T.);
#3556=FACE_OUTER_BOUND('',#5052,.T.);
#3557=FACE_OUTER_BOUND('',#5053,.T.);
#3558=FACE_OUTER_BOUND('',#5055,.T.);
#3559=FACE_OUTER_BOUND('',#5056,.T.);
#3560=FACE_OUTER_BOUND('',#5057,.T.);
#3561=FACE_OUTER_BOUND('',#5058,.T.);
#3562=FACE_OUTER_BOUND('',#5059,.T.);
#3563=FACE_OUTER_BOUND('',#5061,.T.);
#4894=EDGE_LOOP('',(#20817,#20818,#20819,#20820,#20821,#20822,#20823,#20824));
#4895=EDGE_LOOP('',(#20825,#20826,#20827,#20828));
#4896=EDGE_LOOP('',(#20829,#20830,#20831,#20832));
#4897=EDGE_LOOP('',(#20833,#20834,#20835,#20836));
#4898=EDGE_LOOP('',(#20837,#20838,#20839,#20840));
#4899=EDGE_LOOP('',(#20841,#20842,#20843,#20844));
#4900=EDGE_LOOP('',(#20845,#20846,#20847,#20848));
#4901=EDGE_LOOP('',(#20849,#20850,#20851,#20852));
#4902=EDGE_LOOP('',(#20853,#20854,#20855,#20856));
#4903=EDGE_LOOP('',(#20857,#20858,#20859,#20860));
#4904=EDGE_LOOP('',(#20861,#20862,#20863,#20864));
#4905=EDGE_LOOP('',(#20865,#20866,#20867,#20868));
#4906=EDGE_LOOP('',(#20869,#20870,#20871,#20872));
#4907=EDGE_LOOP('',(#20873,#20874,#20875,#20876));
#4908=EDGE_LOOP('',(#20877,#20878,#20879,#20880));
#4909=EDGE_LOOP('',(#20881,#20882,#20883,#20884));
#4910=EDGE_LOOP('',(#20885,#20886,#20887,#20888));
#4911=EDGE_LOOP('',(#20889,#20890,#20891,#20892));
#4912=EDGE_LOOP('',(#20893,#20894,#20895,#20896));
#4913=EDGE_LOOP('',(#20897,#20898,#20899,#20900));
#4914=EDGE_LOOP('',(#20901,#20902,#20903,#20904));
#4915=EDGE_LOOP('',(#20905,#20906,#20907,#20908));
#4916=EDGE_LOOP('',(#20909,#20910,#20911,#20912));
#4917=EDGE_LOOP('',(#20913,#20914,#20915,#20916));
#4918=EDGE_LOOP('',(#20917,#20918,#20919,#20920));
#4919=EDGE_LOOP('',(#20921,#20922,#20923,#20924));
#4920=EDGE_LOOP('',(#20925,#20926,#20927,#20928));
#4921=EDGE_LOOP('',(#20929,#20930,#20931,#20932));
#4922=EDGE_LOOP('',(#20933,#20934,#20935,#20936));
#4923=EDGE_LOOP('',(#20937,#20938,#20939,#20940));
#4924=EDGE_LOOP('',(#20941,#20942,#20943,#20944));
#4925=EDGE_LOOP('',(#20945,#20946,#20947,#20948));
#4926=EDGE_LOOP('',(#20949,#20950,#20951,#20952));
#4927=EDGE_LOOP('',(#20953,#20954,#20955,#20956));
#4928=EDGE_LOOP('',(#20957,#20958,#20959,#20960));
#4929=EDGE_LOOP('',(#20961,#20962,#20963,#20964));
#4930=EDGE_LOOP('',(#20965,#20966,#20967,#20968));
#4931=EDGE_LOOP('',(#20969,#20970,#20971,#20972,#20973));
#4932=EDGE_LOOP('',(#20974,#20975,#20976,#20977,#20978,#20979,#20980,#20981,
#20982,#20983,#20984,#20985,#20986,#20987,#20988,#20989,#20990,#20991,#20992,
#20993,#20994,#20995,#20996,#20997,#20998,#20999,#21000,#21001,#21002,#21003,
#21004,#21005,#21006,#21007,#21008,#21009,#21010,#21011,#21012,#21013,#21014));
#4933=EDGE_LOOP('',(#21015,#21016,#21017,#21018,#21019));
#4934=EDGE_LOOP('',(#21020,#21021,#21022,#21023));
#4935=EDGE_LOOP('',(#21024,#21025,#21026,#21027,#21028,#21029,#21030,#21031,
#21032,#21033,#21034,#21035,#21036,#21037,#21038,#21039,#21040,#21041,#21042,
#21043,#21044,#21045,#21046,#21047,#21048,#21049,#21050,#21051,#21052,#21053,
#21054,#21055,#21056,#21057,#21058,#21059,#21060,#21061,#21062,#21063,#21064));
#4936=EDGE_LOOP('',(#21065,#21066,#21067));
#4937=EDGE_LOOP('',(#21068,#21069,#21070,#21071));
#4938=EDGE_LOOP('',(#21072,#21073,#21074,#21075));
#4939=EDGE_LOOP('',(#21076,#21077,#21078));
#4940=EDGE_LOOP('',(#21079,#21080,#21081,#21082));
#4941=EDGE_LOOP('',(#21083,#21084,#21085,#21086));
#4942=EDGE_LOOP('',(#21087,#21088,#21089));
#4943=EDGE_LOOP('',(#21090,#21091,#21092,#21093));
#4944=EDGE_LOOP('',(#21094,#21095,#21096,#21097));
#4945=EDGE_LOOP('',(#21098,#21099,#21100));
#4946=EDGE_LOOP('',(#21101,#21102,#21103,#21104));
#4947=EDGE_LOOP('',(#21105,#21106,#21107,#21108));
#4948=EDGE_LOOP('',(#21109,#21110,#21111));
#4949=EDGE_LOOP('',(#21112,#21113,#21114,#21115));
#4950=EDGE_LOOP('',(#21116,#21117,#21118,#21119));
#4951=EDGE_LOOP('',(#21120,#21121,#21122));
#4952=EDGE_LOOP('',(#21123,#21124,#21125,#21126));
#4953=EDGE_LOOP('',(#21127,#21128,#21129,#21130));
#4954=EDGE_LOOP('',(#21131,#21132,#21133));
#4955=EDGE_LOOP('',(#21134,#21135,#21136,#21137));
#4956=EDGE_LOOP('',(#21138,#21139,#21140,#21141));
#4957=EDGE_LOOP('',(#21142,#21143,#21144));
#4958=EDGE_LOOP('',(#21145,#21146,#21147,#21148));
#4959=EDGE_LOOP('',(#21149,#21150,#21151,#21152));
#4960=EDGE_LOOP('',(#21153,#21154,#21155));
#4961=EDGE_LOOP('',(#21156,#21157,#21158,#21159));
#4962=EDGE_LOOP('',(#21160,#21161,#21162,#21163));
#4963=EDGE_LOOP('',(#21164,#21165,#21166));
#4964=EDGE_LOOP('',(#21167,#21168,#21169,#21170));
#4965=EDGE_LOOP('',(#21171,#21172,#21173,#21174));
#4966=EDGE_LOOP('',(#21175,#21176,#21177));
#4967=EDGE_LOOP('',(#21178,#21179,#21180,#21181));
#4968=EDGE_LOOP('',(#21182,#21183,#21184,#21185));
#4969=EDGE_LOOP('',(#21186,#21187,#21188));
#4970=EDGE_LOOP('',(#21189,#21190,#21191,#21192));
#4971=EDGE_LOOP('',(#21193,#21194,#21195,#21196));
#4972=EDGE_LOOP('',(#21197,#21198,#21199));
#4973=EDGE_LOOP('',(#21200,#21201,#21202,#21203));
#4974=EDGE_LOOP('',(#21204,#21205,#21206,#21207));
#4975=EDGE_LOOP('',(#21208,#21209,#21210));
#4976=EDGE_LOOP('',(#21211,#21212,#21213,#21214));
#4977=EDGE_LOOP('',(#21215,#21216,#21217,#21218));
#4978=EDGE_LOOP('',(#21219,#21220,#21221));
#4979=EDGE_LOOP('',(#21222,#21223,#21224,#21225));
#4980=EDGE_LOOP('',(#21226,#21227,#21228,#21229));
#4981=EDGE_LOOP('',(#21230,#21231,#21232));
#4982=EDGE_LOOP('',(#21233,#21234,#21235,#21236));
#4983=EDGE_LOOP('',(#21237,#21238,#21239,#21240));
#4984=EDGE_LOOP('',(#21241,#21242,#21243));
#4985=EDGE_LOOP('',(#21244,#21245,#21246,#21247));
#4986=EDGE_LOOP('',(#21248,#21249,#21250,#21251));
#4987=EDGE_LOOP('',(#21252,#21253,#21254,#21255));
#4988=EDGE_LOOP('',(#21256,#21257,#21258,#21259));
#4989=EDGE_LOOP('',(#21260,#21261,#21262,#21263));
#4990=EDGE_LOOP('',(#21264,#21265,#21266));
#4991=EDGE_LOOP('',(#21267,#21268,#21269,#21270));
#4992=EDGE_LOOP('',(#21271,#21272,#21273,#21274));
#4993=EDGE_LOOP('',(#21275,#21276,#21277));
#4994=EDGE_LOOP('',(#21278,#21279,#21280,#21281));
#4995=EDGE_LOOP('',(#21282,#21283,#21284,#21285));
#4996=EDGE_LOOP('',(#21286,#21287,#21288));
#4997=EDGE_LOOP('',(#21289,#21290,#21291,#21292));
#4998=EDGE_LOOP('',(#21293,#21294,#21295,#21296));
#4999=EDGE_LOOP('',(#21297,#21298,#21299));
#5000=EDGE_LOOP('',(#21300,#21301,#21302,#21303));
#5001=EDGE_LOOP('',(#21304,#21305,#21306,#21307));
#5002=EDGE_LOOP('',(#21308,#21309,#21310));
#5003=EDGE_LOOP('',(#21311,#21312,#21313,#21314));
#5004=EDGE_LOOP('',(#21315,#21316,#21317,#21318));
#5005=EDGE_LOOP('',(#21319,#21320,#21321));
#5006=EDGE_LOOP('',(#21322,#21323,#21324,#21325));
#5007=EDGE_LOOP('',(#21326,#21327,#21328,#21329));
#5008=EDGE_LOOP('',(#21330,#21331,#21332));
#5009=EDGE_LOOP('',(#21333,#21334,#21335,#21336));
#5010=EDGE_LOOP('',(#21337,#21338,#21339,#21340));
#5011=EDGE_LOOP('',(#21341,#21342,#21343));
#5012=EDGE_LOOP('',(#21344,#21345,#21346,#21347));
#5013=EDGE_LOOP('',(#21348,#21349,#21350,#21351));
#5014=EDGE_LOOP('',(#21352,#21353,#21354));
#5015=EDGE_LOOP('',(#21355,#21356,#21357,#21358));
#5016=EDGE_LOOP('',(#21359,#21360,#21361,#21362));
#5017=EDGE_LOOP('',(#21363,#21364,#21365));
#5018=EDGE_LOOP('',(#21366,#21367,#21368,#21369));
#5019=EDGE_LOOP('',(#21370,#21371,#21372,#21373));
#5020=EDGE_LOOP('',(#21374,#21375,#21376));
#5021=EDGE_LOOP('',(#21377,#21378,#21379,#21380));
#5022=EDGE_LOOP('',(#21381,#21382,#21383,#21384));
#5023=EDGE_LOOP('',(#21385,#21386,#21387));
#5024=EDGE_LOOP('',(#21388,#21389,#21390,#21391));
#5025=EDGE_LOOP('',(#21392,#21393,#21394,#21395));
#5026=EDGE_LOOP('',(#21396,#21397,#21398));
#5027=EDGE_LOOP('',(#21399,#21400,#21401,#21402));
#5028=EDGE_LOOP('',(#21403,#21404,#21405,#21406));
#5029=EDGE_LOOP('',(#21407,#21408,#21409));
#5030=EDGE_LOOP('',(#21410,#21411,#21412,#21413));
#5031=EDGE_LOOP('',(#21414,#21415,#21416,#21417));
#5032=EDGE_LOOP('',(#21418,#21419,#21420));
#5033=EDGE_LOOP('',(#21421,#21422,#21423,#21424));
#5034=EDGE_LOOP('',(#21425,#21426,#21427,#21428));
#5035=EDGE_LOOP('',(#21429,#21430,#21431));
#5036=EDGE_LOOP('',(#21432,#21433,#21434,#21435));
#5037=EDGE_LOOP('',(#21436,#21437,#21438,#21439));
#5038=EDGE_LOOP('',(#21440,#21441,#21442));
#5039=EDGE_LOOP('',(#21443,#21444,#21445,#21446));
#5040=EDGE_LOOP('',(#21447,#21448,#21449,#21450));
#5041=EDGE_LOOP('',(#21451,#21452,#21453,#21454,#21455,#21456,#21457,#21458,
#21459,#21460,#21461,#21462,#21463,#21464,#21465,#21466,#21467,#21468,#21469,
#21470,#21471,#21472,#21473,#21474,#21475,#21476,#21477,#21478,#21479,#21480,
#21481,#21482,#21483,#21484,#21485,#21486,#21487,#21488,#21489,#21490,#21491,
#21492,#21493,#21494,#21495,#21496,#21497,#21498,#21499,#21500,#21501,#21502,
#21503,#21504,#21505,#21506,#21507,#21508,#21509,#21510,#21511,#21512,#21513,
#21514,#21515,#21516,#21517,#21518,#21519,#21520,#21521,#21522,#21523,#21524,
#21525,#21526,#21527,#21528,#21529,#21530,#21531,#21532,#21533,#21534,#21535,
#21536,#21537,#21538,#21539,#21540,#21541,#21542,#21543,#21544,#21545,#21546,
#21547,#21548,#21549,#21550,#21551,#21552,#21553,#21554,#21555,#21556,#21557,
#21558,#21559,#21560,#21561,#21562,#21563,#21564,#21565,#21566,#21567,#21568,
#21569,#21570,#21571,#21572,#21573,#21574,#21575,#21576,#21577,#21578,#21579,
#21580,#21581,#21582,#21583,#21584,#21585,#21586,#21587,#21588,#21589,#21590,
#21591,#21592,#21593,#21594,#21595,#21596,#21597,#21598));
#5042=EDGE_LOOP('',(#21599,#21600,#21601,#21602));
#5043=EDGE_LOOP('',(#21603,#21604,#21605,#21606));
#5044=EDGE_LOOP('',(#21607,#21608,#21609));
#5045=EDGE_LOOP('',(#21610,#21611,#21612,#21613,#21614,#21615,#21616,#21617,
#21618,#21619,#21620,#21621,#21622,#21623,#21624,#21625,#21626,#21627,#21628,
#21629,#21630,#21631,#21632,#21633,#21634,#21635,#21636,#21637,#21638,#21639,
#21640,#21641,#21642,#21643,#21644,#21645,#21646,#21647,#21648,#21649,#21650,
#21651,#21652,#21653,#21654,#21655,#21656,#21657,#21658,#21659,#21660,#21661,
#21662,#21663,#21664,#21665,#21666,#21667,#21668,#21669,#21670,#21671,#21672,
#21673,#21674,#21675,#21676,#21677,#21678,#21679,#21680,#21681,#21682,#21683,
#21684,#21685,#21686,#21687,#21688,#21689,#21690,#21691,#21692,#21693,#21694,
#21695,#21696,#21697,#21698,#21699,#21700,#21701,#21702,#21703,#21704,#21705,
#21706,#21707,#21708,#21709,#21710,#21711,#21712,#21713,#21714,#21715,#21716,
#21717,#21718,#21719,#21720));
#5046=EDGE_LOOP('',(#21721,#21722,#21723));
#5047=EDGE_LOOP('',(#21724,#21725,#21726,#21727));
#5048=EDGE_LOOP('',(#21728,#21729,#21730,#21731));
#5049=EDGE_LOOP('',(#21732,#21733,#21734,#21735));
#5050=EDGE_LOOP('',(#21736,#21737,#21738,#21739));
#5051=EDGE_LOOP('',(#21740,#21741,#21742,#21743));
#5052=EDGE_LOOP('',(#21744,#21745,#21746,#21747));
#5053=EDGE_LOOP('',(#21748,#21749,#21750,#21751,#21752,#21753));
#5054=EDGE_LOOP('',(#21754));
#5055=EDGE_LOOP('',(#21755));
#5056=EDGE_LOOP('',(#21756,#21757,#21758,#21759));
#5057=EDGE_LOOP('',(#21760,#21761,#21762,#21763));
#5058=EDGE_LOOP('',(#21764,#21765,#21766,#21767,#21768,#21769));
#5059=EDGE_LOOP('',(#21770));
#5060=EDGE_LOOP('',(#21771));
#5061=EDGE_LOOP('',(#21772));
#5062=EDGE_LOOP('',(#21773,#21774,#21775,#21776,#21777,#21778));
#5766=CIRCLE('',#25371,0.24505);
#5767=CIRCLE('',#25372,0.24505);
#5768=CIRCLE('',#25373,0.24505);
#5769=CIRCLE('',#25392,0.199475);
#5770=CIRCLE('',#25412,0.24505);
#5771=CIRCLE('',#25413,0.24505);
#5772=CIRCLE('',#25415,0.199475);
#5773=CIRCLE('',#25418,0.425);
#5774=CIRCLE('',#25422,0.425);
#5775=CIRCLE('',#25426,0.425);
#5776=CIRCLE('',#25430,0.425);
#5777=CIRCLE('',#25434,0.425);
#5778=CIRCLE('',#25438,0.425);
#5779=CIRCLE('',#25442,0.425);
#5780=CIRCLE('',#25446,0.425);
#5781=CIRCLE('',#25450,0.425);
#5782=CIRCLE('',#25454,0.425);
#5783=CIRCLE('',#25458,0.425);
#5784=CIRCLE('',#25462,0.425);
#5785=CIRCLE('',#25466,0.425);
#5786=CIRCLE('',#25470,0.425);
#5787=CIRCLE('',#25474,0.425);
#5788=CIRCLE('',#25478,0.425);
#5789=CIRCLE('',#25482,0.425);
#5790=CIRCLE('',#25486,0.425);
#5791=CIRCLE('',#25487,0.425);
#5792=CIRCLE('',#25491,0.425);
#5793=CIRCLE('',#25495,0.425);
#5794=CIRCLE('',#25499,0.425);
#5795=CIRCLE('',#25503,0.425);
#5796=CIRCLE('',#25507,0.425);
#5797=CIRCLE('',#25511,0.425);
#5798=CIRCLE('',#25515,0.425);
#5799=CIRCLE('',#25519,0.425);
#5800=CIRCLE('',#25523,0.425);
#5801=CIRCLE('',#25527,0.425);
#5802=CIRCLE('',#25531,0.425);
#5803=CIRCLE('',#25535,0.425);
#5804=CIRCLE('',#25539,0.425);
#5805=CIRCLE('',#25543,0.425);
#5806=CIRCLE('',#25547,0.425);
#5807=CIRCLE('',#25551,0.425);
#5808=CIRCLE('',#25555,0.425);
#5809=CIRCLE('',#25559,0.425);
#5810=CIRCLE('',#25560,0.425);
#5811=CIRCLE('',#25561,0.425);
#5812=CIRCLE('',#25562,0.425);
#5813=CIRCLE('',#25563,0.425);
#5814=CIRCLE('',#25564,0.425);
#5815=CIRCLE('',#25565,0.425);
#5816=CIRCLE('',#25566,0.425);
#5817=CIRCLE('',#25567,0.425);
#5818=CIRCLE('',#25568,0.425);
#5819=CIRCLE('',#25569,0.425);
#5820=CIRCLE('',#25570,0.425);
#5821=CIRCLE('',#25571,0.425);
#5822=CIRCLE('',#25572,0.425);
#5823=CIRCLE('',#25573,0.425);
#5824=CIRCLE('',#25574,0.425);
#5825=CIRCLE('',#25575,0.425);
#5826=CIRCLE('',#25576,0.425);
#5827=CIRCLE('',#25577,0.425);
#5828=CIRCLE('',#25578,0.425);
#5829=CIRCLE('',#25579,0.425);
#5830=CIRCLE('',#25580,0.425);
#5831=CIRCLE('',#25581,0.425);
#5832=CIRCLE('',#25582,0.425);
#5833=CIRCLE('',#25583,0.425);
#5834=CIRCLE('',#25584,0.425);
#5835=CIRCLE('',#25585,0.425);
#5836=CIRCLE('',#25586,0.425);
#5837=CIRCLE('',#25587,0.425);
#5838=CIRCLE('',#25588,0.425);
#5839=CIRCLE('',#25589,0.425);
#5840=CIRCLE('',#25590,0.425);
#5841=CIRCLE('',#25591,0.425);
#5842=CIRCLE('',#25592,0.425);
#5843=CIRCLE('',#25593,0.425);
#5844=CIRCLE('',#25594,0.425);
#5845=CIRCLE('',#25595,0.425);
#5846=CIRCLE('',#25596,0.425);
#5847=CIRCLE('',#25601,0.41);
#5848=CIRCLE('',#25603,0.183165823577449);
#5849=CIRCLE('',#25612,0.19);
#5850=CIRCLE('',#25615,0.24505);
#5851=CIRCLE('',#25617,0.26);
#7456=LINE('',#50093,#9301);
#7457=LINE('',#50120,#9302);
#7458=LINE('',#50146,#9303);
#7459=LINE('',#50194,#9304);
#7460=LINE('',#50242,#9305);
#7461=LINE('',#50290,#9306);
#7462=LINE('',#50344,#9307);
#7463=LINE('',#50392,#9308);
#7464=LINE('',#50440,#9309);
#7465=LINE('',#50494,#9310);
#7466=LINE('',#50542,#9311);
#7467=LINE('',#50590,#9312);
#7468=LINE('',#50638,#9313);
#7469=LINE('',#50692,#9314);
#7470=LINE('',#50740,#9315);
#7471=LINE('',#50788,#9316);
#7472=LINE('',#50842,#9317);
#7473=LINE('',#50890,#9318);
#7474=LINE('',#50938,#9319);
#7475=LINE('',#50986,#9320);
#7476=LINE('',#51005,#9321);
#7477=LINE('',#51030,#9322);
#7478=LINE('',#51054,#9323);
#7479=LINE('',#51078,#9324);
#7480=LINE('',#51103,#9325);
#7481=LINE('',#51128,#9326);
#7482=LINE('',#51152,#9327);
#7483=LINE('',#51177,#9328);
#7484=LINE('',#51202,#9329);
#7485=LINE('',#51226,#9330);
#7486=LINE('',#51250,#9331);
#7487=LINE('',#51275,#9332);
#7488=LINE('',#51300,#9333);
#7489=LINE('',#51324,#9334);
#7490=LINE('',#51349,#9335);
#7491=LINE('',#51374,#9336);
#7492=LINE('',#51398,#9337);
#7493=LINE('',#51422,#9338);
#7494=LINE('',#52729,#9339);
#7495=LINE('',#52730,#9340);
#7496=LINE('',#52733,#9341);
#7497=LINE('',#52735,#9342);
#7498=LINE('',#52741,#9343);
#7499=LINE('',#52750,#9344);
#7500=LINE('',#52751,#9345);
#7501=LINE('',#52754,#9346);
#7502=LINE('',#52756,#9347);
#7503=LINE('',#52762,#9348);
#7504=LINE('',#52771,#9349);
#7505=LINE('',#52772,#9350);
#7506=LINE('',#52775,#9351);
#7507=LINE('',#52777,#9352);
#7508=LINE('',#52783,#9353);
#7509=LINE('',#52792,#9354);
#7510=LINE('',#52793,#9355);
#7511=LINE('',#52796,#9356);
#7512=LINE('',#52798,#9357);
#7513=LINE('',#52804,#9358);
#7514=LINE('',#52813,#9359);
#7515=LINE('',#52814,#9360);
#7516=LINE('',#52817,#9361);
#7517=LINE('',#52819,#9362);
#7518=LINE('',#52825,#9363);
#7519=LINE('',#52834,#9364);
#7520=LINE('',#52835,#9365);
#7521=LINE('',#52838,#9366);
#7522=LINE('',#52840,#9367);
#7523=LINE('',#52846,#9368);
#7524=LINE('',#52855,#9369);
#7525=LINE('',#52856,#9370);
#7526=LINE('',#52859,#9371);
#7527=LINE('',#52861,#9372);
#7528=LINE('',#52867,#9373);
#7529=LINE('',#52876,#9374);
#7530=LINE('',#52877,#9375);
#7531=LINE('',#52880,#9376);
#7532=LINE('',#52882,#9377);
#7533=LINE('',#52888,#9378);
#7534=LINE('',#52897,#9379);
#7535=LINE('',#52898,#9380);
#7536=LINE('',#52901,#9381);
#7537=LINE('',#52903,#9382);
#7538=LINE('',#52909,#9383);
#7539=LINE('',#52918,#9384);
#7540=LINE('',#52919,#9385);
#7541=LINE('',#52922,#9386);
#7542=LINE('',#52924,#9387);
#7543=LINE('',#52930,#9388);
#7544=LINE('',#52939,#9389);
#7545=LINE('',#52940,#9390);
#7546=LINE('',#52943,#9391);
#7547=LINE('',#52945,#9392);
#7548=LINE('',#52951,#9393);
#7549=LINE('',#52960,#9394);
#7550=LINE('',#52961,#9395);
#7551=LINE('',#52964,#9396);
#7552=LINE('',#52966,#9397);
#7553=LINE('',#52972,#9398);
#7554=LINE('',#52981,#9399);
#7555=LINE('',#52982,#9400);
#7556=LINE('',#52985,#9401);
#7557=LINE('',#52987,#9402);
#7558=LINE('',#52993,#9403);
#7559=LINE('',#53002,#9404);
#7560=LINE('',#53003,#9405);
#7561=LINE('',#53006,#9406);
#7562=LINE('',#53008,#9407);
#7563=LINE('',#53014,#9408);
#7564=LINE('',#53023,#9409);
#7565=LINE('',#53024,#9410);
#7566=LINE('',#53027,#9411);
#7567=LINE('',#53029,#9412);
#7568=LINE('',#53035,#9413);
#7569=LINE('',#53044,#9414);
#7570=LINE('',#53045,#9415);
#7571=LINE('',#53048,#9416);
#7572=LINE('',#53050,#9417);
#7573=LINE('',#53056,#9418);
#7574=LINE('',#53065,#9419);
#7575=LINE('',#53066,#9420);
#7576=LINE('',#53069,#9421);
#7577=LINE('',#53071,#9422);
#7578=LINE('',#53077,#9423);
#7579=LINE('',#53086,#9424);
#7580=LINE('',#53088,#9425);
#7581=LINE('',#53092,#9426);
#7582=LINE('',#53094,#9427);
#7583=LINE('',#53100,#9428);
#7584=LINE('',#53109,#9429);
#7585=LINE('',#53110,#9430);
#7586=LINE('',#53113,#9431);
#7587=LINE('',#53115,#9432);
#7588=LINE('',#53121,#9433);
#7589=LINE('',#53130,#9434);
#7590=LINE('',#53131,#9435);
#7591=LINE('',#53134,#9436);
#7592=LINE('',#53136,#9437);
#7593=LINE('',#53142,#9438);
#7594=LINE('',#53151,#9439);
#7595=LINE('',#53152,#9440);
#7596=LINE('',#53155,#9441);
#7597=LINE('',#53157,#9442);
#7598=LINE('',#53163,#9443);
#7599=LINE('',#53172,#9444);
#7600=LINE('',#53173,#9445);
#7601=LINE('',#53176,#9446);
#7602=LINE('',#53178,#9447);
#7603=LINE('',#53184,#9448);
#7604=LINE('',#53193,#9449);
#7605=LINE('',#53194,#9450);
#7606=LINE('',#53197,#9451);
#7607=LINE('',#53199,#9452);
#7608=LINE('',#53205,#9453);
#7609=LINE('',#53214,#9454);
#7610=LINE('',#53215,#9455);
#7611=LINE('',#53218,#9456);
#7612=LINE('',#53220,#9457);
#7613=LINE('',#53226,#9458);
#7614=LINE('',#53235,#9459);
#7615=LINE('',#53236,#9460);
#7616=LINE('',#53239,#9461);
#7617=LINE('',#53241,#9462);
#7618=LINE('',#53247,#9463);
#7619=LINE('',#53256,#9464);
#7620=LINE('',#53257,#9465);
#7621=LINE('',#53260,#9466);
#7622=LINE('',#53262,#9467);
#7623=LINE('',#53268,#9468);
#7624=LINE('',#53277,#9469);
#7625=LINE('',#53278,#9470);
#7626=LINE('',#53281,#9471);
#7627=LINE('',#53283,#9472);
#7628=LINE('',#53289,#9473);
#7629=LINE('',#53298,#9474);
#7630=LINE('',#53299,#9475);
#7631=LINE('',#53302,#9476);
#7632=LINE('',#53304,#9477);
#7633=LINE('',#53310,#9478);
#7634=LINE('',#53319,#9479);
#7635=LINE('',#53320,#9480);
#7636=LINE('',#53323,#9481);
#7637=LINE('',#53325,#9482);
#7638=LINE('',#53331,#9483);
#7639=LINE('',#53340,#9484);
#7640=LINE('',#53341,#9485);
#7641=LINE('',#53344,#9486);
#7642=LINE('',#53346,#9487);
#7643=LINE('',#53352,#9488);
#7644=LINE('',#53361,#9489);
#7645=LINE('',#53362,#9490);
#7646=LINE('',#53365,#9491);
#7647=LINE('',#53367,#9492);
#7648=LINE('',#53373,#9493);
#7649=LINE('',#53382,#9494);
#7650=LINE('',#53383,#9495);
#7651=LINE('',#53386,#9496);
#7652=LINE('',#53388,#9497);
#7653=LINE('',#53394,#9498);
#7654=LINE('',#53403,#9499);
#7655=LINE('',#53404,#9500);
#7656=LINE('',#53407,#9501);
#7657=LINE('',#53409,#9502);
#7658=LINE('',#53415,#9503);
#7659=LINE('',#53424,#9504);
#7660=LINE('',#53425,#9505);
#7661=LINE('',#53428,#9506);
#7662=LINE('',#53430,#9507);
#7663=LINE('',#53436,#9508);
#7664=LINE('',#53445,#9509);
#7665=LINE('',#53446,#9510);
#7666=LINE('',#53449,#9511);
#7667=LINE('',#53451,#9512);
#7668=LINE('',#53457,#9513);
#7669=LINE('',#53480,#9514);
#7670=LINE('',#53502,#9515);
#7671=LINE('',#53506,#9516);
#7672=LINE('',#53510,#9517);
#7673=LINE('',#53512,#9518);
#7674=LINE('',#53520,#9519);
#7675=LINE('',#53525,#9520);
#7676=LINE('',#53529,#9521);
#7677=LINE('',#53534,#9522);
#7678=LINE('',#53536,#9523);
#7679=LINE('',#53538,#9524);
#7680=LINE('',#53539,#9525);
#7681=LINE('',#53542,#9526);
#7682=LINE('',#53544,#9527);
#7683=LINE('',#53545,#9528);
#7684=LINE('',#53548,#9529);
#7685=LINE('',#53550,#9530);
#7686=LINE('',#53551,#9531);
#7687=LINE('',#53554,#9532);
#7688=LINE('',#53556,#9533);
#7689=LINE('',#53557,#9534);
#7690=LINE('',#53560,#9535);
#7691=LINE('',#53562,#9536);
#7692=LINE('',#53563,#9537);
#7693=LINE('',#53565,#9538);
#7694=LINE('',#53566,#9539);
#7695=LINE('',#53572,#9540);
#7696=LINE('',#53578,#9541);
#9301=VECTOR('',#31008,0.25);
#9302=VECTOR('',#31011,0.25);
#9303=VECTOR('',#31018,0.25);
#9304=VECTOR('',#31021,0.25);
#9305=VECTOR('',#31024,0.25);
#9306=VECTOR('',#31027,0.25);
#9307=VECTOR('',#31030,0.25);
#9308=VECTOR('',#31033,0.25);
#9309=VECTOR('',#31036,0.25);
#9310=VECTOR('',#31039,0.25);
#9311=VECTOR('',#31042,0.25);
#9312=VECTOR('',#31045,0.25);
#9313=VECTOR('',#31048,0.25);
#9314=VECTOR('',#31051,0.25);
#9315=VECTOR('',#31054,0.25);
#9316=VECTOR('',#31057,0.25);
#9317=VECTOR('',#31060,0.25);
#9318=VECTOR('',#31063,0.25);
#9319=VECTOR('',#31066,0.25);
#9320=VECTOR('',#31069,0.199475);
#9321=VECTOR('',#31074,0.199475);
#9322=VECTOR('',#31077,0.199475);
#9323=VECTOR('',#31080,0.199475);
#9324=VECTOR('',#31083,0.199475);
#9325=VECTOR('',#31086,0.199475);
#9326=VECTOR('',#31089,0.199475);
#9327=VECTOR('',#31092,0.199475);
#9328=VECTOR('',#31095,0.199475);
#9329=VECTOR('',#31098,0.199475);
#9330=VECTOR('',#31101,0.199475);
#9331=VECTOR('',#31104,0.199475);
#9332=VECTOR('',#31107,0.199475);
#9333=VECTOR('',#31110,0.199475);
#9334=VECTOR('',#31113,0.199475);
#9335=VECTOR('',#31116,0.199475);
#9336=VECTOR('',#31119,0.199475);
#9337=VECTOR('',#31122,0.199475);
#9338=VECTOR('',#31125,0.199475);
#9339=VECTOR('',#31142,1.);
#9340=VECTOR('',#31143,1.);
#9341=VECTOR('',#31146,1.);
#9342=VECTOR('',#31147,1.);
#9343=VECTOR('',#31150,1.);
#9344=VECTOR('',#31155,1.);
#9345=VECTOR('',#31156,1.);
#9346=VECTOR('',#31159,1.);
#9347=VECTOR('',#31160,1.);
#9348=VECTOR('',#31163,1.);
#9349=VECTOR('',#31168,1.);
#9350=VECTOR('',#31169,1.);
#9351=VECTOR('',#31172,1.);
#9352=VECTOR('',#31173,1.);
#9353=VECTOR('',#31176,1.);
#9354=VECTOR('',#31181,1.);
#9355=VECTOR('',#31182,1.);
#9356=VECTOR('',#31185,1.);
#9357=VECTOR('',#31186,1.);
#9358=VECTOR('',#31189,1.);
#9359=VECTOR('',#31194,1.);
#9360=VECTOR('',#31195,1.);
#9361=VECTOR('',#31198,1.);
#9362=VECTOR('',#31199,1.);
#9363=VECTOR('',#31202,1.);
#9364=VECTOR('',#31207,1.);
#9365=VECTOR('',#31208,1.);
#9366=VECTOR('',#31211,1.);
#9367=VECTOR('',#31212,1.);
#9368=VECTOR('',#31215,1.);
#9369=VECTOR('',#31220,1.);
#9370=VECTOR('',#31221,1.);
#9371=VECTOR('',#31224,1.);
#9372=VECTOR('',#31225,1.);
#9373=VECTOR('',#31228,1.);
#9374=VECTOR('',#31233,1.);
#9375=VECTOR('',#31234,1.);
#9376=VECTOR('',#31237,1.);
#9377=VECTOR('',#31238,1.);
#9378=VECTOR('',#31241,1.);
#9379=VECTOR('',#31246,1.);
#9380=VECTOR('',#31247,1.);
#9381=VECTOR('',#31250,1.);
#9382=VECTOR('',#31251,1.);
#9383=VECTOR('',#31254,1.);
#9384=VECTOR('',#31259,1.);
#9385=VECTOR('',#31260,1.);
#9386=VECTOR('',#31263,1.);
#9387=VECTOR('',#31264,1.);
#9388=VECTOR('',#31267,1.);
#9389=VECTOR('',#31272,1.);
#9390=VECTOR('',#31273,1.);
#9391=VECTOR('',#31276,1.);
#9392=VECTOR('',#31277,1.);
#9393=VECTOR('',#31280,1.);
#9394=VECTOR('',#31285,1.);
#9395=VECTOR('',#31286,1.);
#9396=VECTOR('',#31289,1.);
#9397=VECTOR('',#31290,1.);
#9398=VECTOR('',#31293,1.);
#9399=VECTOR('',#31298,1.);
#9400=VECTOR('',#31299,1.);
#9401=VECTOR('',#31302,1.);
#9402=VECTOR('',#31303,1.);
#9403=VECTOR('',#31306,1.);
#9404=VECTOR('',#31311,1.);
#9405=VECTOR('',#31312,1.);
#9406=VECTOR('',#31315,1.);
#9407=VECTOR('',#31316,1.);
#9408=VECTOR('',#31319,1.);
#9409=VECTOR('',#31324,1.);
#9410=VECTOR('',#31325,1.);
#9411=VECTOR('',#31328,1.);
#9412=VECTOR('',#31329,1.);
#9413=VECTOR('',#31332,1.);
#9414=VECTOR('',#31337,1.);
#9415=VECTOR('',#31338,1.);
#9416=VECTOR('',#31341,1.);
#9417=VECTOR('',#31342,1.);
#9418=VECTOR('',#31345,1.);
#9419=VECTOR('',#31350,1.);
#9420=VECTOR('',#31351,1.);
#9421=VECTOR('',#31354,1.);
#9422=VECTOR('',#31355,1.);
#9423=VECTOR('',#31358,1.);
#9424=VECTOR('',#31363,1.);
#9425=VECTOR('',#31364,1.);
#9426=VECTOR('',#31369,1.);
#9427=VECTOR('',#31370,1.);
#9428=VECTOR('',#31373,1.);
#9429=VECTOR('',#31378,1.);
#9430=VECTOR('',#31379,1.);
#9431=VECTOR('',#31382,1.);
#9432=VECTOR('',#31383,1.);
#9433=VECTOR('',#31386,1.);
#9434=VECTOR('',#31391,1.);
#9435=VECTOR('',#31392,1.);
#9436=VECTOR('',#31395,1.);
#9437=VECTOR('',#31396,1.);
#9438=VECTOR('',#31399,1.);
#9439=VECTOR('',#31404,1.);
#9440=VECTOR('',#31405,1.);
#9441=VECTOR('',#31408,1.);
#9442=VECTOR('',#31409,1.);
#9443=VECTOR('',#31412,1.);
#9444=VECTOR('',#31417,1.);
#9445=VECTOR('',#31418,1.);
#9446=VECTOR('',#31421,1.);
#9447=VECTOR('',#31422,1.);
#9448=VECTOR('',#31425,1.);
#9449=VECTOR('',#31430,1.);
#9450=VECTOR('',#31431,1.);
#9451=VECTOR('',#31434,1.);
#9452=VECTOR('',#31435,1.);
#9453=VECTOR('',#31438,1.);
#9454=VECTOR('',#31443,1.);
#9455=VECTOR('',#31444,1.);
#9456=VECTOR('',#31447,1.);
#9457=VECTOR('',#31448,1.);
#9458=VECTOR('',#31451,1.);
#9459=VECTOR('',#31456,1.);
#9460=VECTOR('',#31457,1.);
#9461=VECTOR('',#31460,1.);
#9462=VECTOR('',#31461,1.);
#9463=VECTOR('',#31464,1.);
#9464=VECTOR('',#31469,1.);
#9465=VECTOR('',#31470,1.);
#9466=VECTOR('',#31473,1.);
#9467=VECTOR('',#31474,1.);
#9468=VECTOR('',#31477,1.);
#9469=VECTOR('',#31482,1.);
#9470=VECTOR('',#31483,1.);
#9471=VECTOR('',#31486,1.);
#9472=VECTOR('',#31487,1.);
#9473=VECTOR('',#31490,1.);
#9474=VECTOR('',#31495,1.);
#9475=VECTOR('',#31496,1.);
#9476=VECTOR('',#31499,1.);
#9477=VECTOR('',#31500,1.);
#9478=VECTOR('',#31503,1.);
#9479=VECTOR('',#31508,1.);
#9480=VECTOR('',#31509,1.);
#9481=VECTOR('',#31512,1.);
#9482=VECTOR('',#31513,1.);
#9483=VECTOR('',#31516,1.);
#9484=VECTOR('',#31521,1.);
#9485=VECTOR('',#31522,1.);
#9486=VECTOR('',#31525,1.);
#9487=VECTOR('',#31526,1.);
#9488=VECTOR('',#31529,1.);
#9489=VECTOR('',#31534,1.);
#9490=VECTOR('',#31535,1.);
#9491=VECTOR('',#31538,1.);
#9492=VECTOR('',#31539,1.);
#9493=VECTOR('',#31542,1.);
#9494=VECTOR('',#31547,1.);
#9495=VECTOR('',#31548,1.);
#9496=VECTOR('',#31551,1.);
#9497=VECTOR('',#31552,1.);
#9498=VECTOR('',#31555,1.);
#9499=VECTOR('',#31560,1.);
#9500=VECTOR('',#31561,1.);
#9501=VECTOR('',#31564,1.);
#9502=VECTOR('',#31565,1.);
#9503=VECTOR('',#31568,1.);
#9504=VECTOR('',#31573,1.);
#9505=VECTOR('',#31574,1.);
#9506=VECTOR('',#31577,1.);
#9507=VECTOR('',#31578,1.);
#9508=VECTOR('',#31581,1.);
#9509=VECTOR('',#31586,1.);
#9510=VECTOR('',#31587,1.);
#9511=VECTOR('',#31590,1.);
#9512=VECTOR('',#31591,1.);
#9513=VECTOR('',#31594,1.);
#9514=VECTOR('',#31631,0.425);
#9515=VECTOR('',#31670,1.);
#9516=VECTOR('',#31673,1.);
#9517=VECTOR('',#31678,1.);
#9518=VECTOR('',#31679,1.);
#9519=VECTOR('',#31682,1.);
#9520=VECTOR('',#31689,0.4175);
#9521=VECTOR('',#31692,0.0923760430703401);
#9522=VECTOR('',#31697,1.);
#9523=VECTOR('',#31698,1.);
#9524=VECTOR('',#31699,1.);
#9525=VECTOR('',#31700,1.);
#9526=VECTOR('',#31703,1.);
#9527=VECTOR('',#31704,1.);
#9528=VECTOR('',#31705,1.);
#9529=VECTOR('',#31708,1.);
#9530=VECTOR('',#31709,1.);
#9531=VECTOR('',#31710,1.);
#9532=VECTOR('',#31713,1.);
#9533=VECTOR('',#31714,1.);
#9534=VECTOR('',#31715,1.);
#9535=VECTOR('',#31718,1.);
#9536=VECTOR('',#31719,1.);
#9537=VECTOR('',#31720,1.);
#9538=VECTOR('',#31723,1.);
#9539=VECTOR('',#31724,1.);
#9540=VECTOR('',#31733,0.22);
#9541=VECTOR('',#31742,0.255);
#11391=VERTEX_POINT('',#50091);
#11392=VERTEX_POINT('',#50092);
#11393=VERTEX_POINT('',#50094);
#11394=VERTEX_POINT('',#50117);
#11395=VERTEX_POINT('',#50119);
#11396=VERTEX_POINT('',#50122);
#11397=VERTEX_POINT('',#50144);
#11398=VERTEX_POINT('',#50145);
#11399=VERTEX_POINT('',#50192);
#11400=VERTEX_POINT('',#50193);
#11401=VERTEX_POINT('',#50240);
#11402=VERTEX_POINT('',#50241);
#11403=VERTEX_POINT('',#50288);
#11404=VERTEX_POINT('',#50289);
#11405=VERTEX_POINT('',#50342);
#11406=VERTEX_POINT('',#50343);
#11407=VERTEX_POINT('',#50390);
#11408=VERTEX_POINT('',#50391);
#11409=VERTEX_POINT('',#50438);
#11410=VERTEX_POINT('',#50439);
#11411=VERTEX_POINT('',#50492);
#11412=VERTEX_POINT('',#50493);
#11413=VERTEX_POINT('',#50540);
#11414=VERTEX_POINT('',#50541);
#11415=VERTEX_POINT('',#50588);
#11416=VERTEX_POINT('',#50589);
#11417=VERTEX_POINT('',#50636);
#11418=VERTEX_POINT('',#50637);
#11419=VERTEX_POINT('',#50690);
#11420=VERTEX_POINT('',#50691);
#11421=VERTEX_POINT('',#50738);
#11422=VERTEX_POINT('',#50739);
#11423=VERTEX_POINT('',#50786);
#11424=VERTEX_POINT('',#50787);
#11425=VERTEX_POINT('',#50840);
#11426=VERTEX_POINT('',#50841);
#11427=VERTEX_POINT('',#50888);
#11428=VERTEX_POINT('',#50889);
#11429=VERTEX_POINT('',#50936);
#11430=VERTEX_POINT('',#50937);
#11431=VERTEX_POINT('',#50984);
#11432=VERTEX_POINT('',#50985);
#11433=VERTEX_POINT('',#50987);
#11434=VERTEX_POINT('',#50995);
#11435=VERTEX_POINT('',#51003);
#11436=VERTEX_POINT('',#51004);
#11437=VERTEX_POINT('',#51028);
#11438=VERTEX_POINT('',#51029);
#11439=VERTEX_POINT('',#51052);
#11440=VERTEX_POINT('',#51053);
#11441=VERTEX_POINT('',#51076);
#11442=VERTEX_POINT('',#51077);
#11443=VERTEX_POINT('',#51101);
#11444=VERTEX_POINT('',#51102);
#11445=VERTEX_POINT('',#51126);
#11446=VERTEX_POINT('',#51127);
#11447=VERTEX_POINT('',#51150);
#11448=VERTEX_POINT('',#51151);
#11449=VERTEX_POINT('',#51175);
#11450=VERTEX_POINT('',#51176);
#11451=VERTEX_POINT('',#51200);
#11452=VERTEX_POINT('',#51201);
#11453=VERTEX_POINT('',#51224);
#11454=VERTEX_POINT('',#51225);
#11455=VERTEX_POINT('',#51248);
#11456=VERTEX_POINT('',#51249);
#11457=VERTEX_POINT('',#51273);
#11458=VERTEX_POINT('',#51274);
#11459=VERTEX_POINT('',#51298);
#11460=VERTEX_POINT('',#51299);
#11461=VERTEX_POINT('',#51322);
#11462=VERTEX_POINT('',#51323);
#11463=VERTEX_POINT('',#51347);
#11464=VERTEX_POINT('',#51348);
#11465=VERTEX_POINT('',#51372);
#11466=VERTEX_POINT('',#51373);
#11467=VERTEX_POINT('',#51396);
#11468=VERTEX_POINT('',#51397);
#11469=VERTEX_POINT('',#51420);
#11470=VERTEX_POINT('',#51421);
#11471=VERTEX_POINT('',#51445);
#11472=VERTEX_POINT('',#51504);
#11473=VERTEX_POINT('',#51506);
#11474=VERTEX_POINT('',#52080);
#11475=VERTEX_POINT('',#52147);
#11476=VERTEX_POINT('',#52725);
#11477=VERTEX_POINT('',#52726);
#11478=VERTEX_POINT('',#52728);
#11479=VERTEX_POINT('',#52732);
#11480=VERTEX_POINT('',#52734);
#11481=VERTEX_POINT('',#52740);
#11482=VERTEX_POINT('',#52746);
#11483=VERTEX_POINT('',#52747);
#11484=VERTEX_POINT('',#52749);
#11485=VERTEX_POINT('',#52753);
#11486=VERTEX_POINT('',#52755);
#11487=VERTEX_POINT('',#52761);
#11488=VERTEX_POINT('',#52767);
#11489=VERTEX_POINT('',#52768);
#11490=VERTEX_POINT('',#52770);
#11491=VERTEX_POINT('',#52774);
#11492=VERTEX_POINT('',#52776);
#11493=VERTEX_POINT('',#52782);
#11494=VERTEX_POINT('',#52788);
#11495=VERTEX_POINT('',#52789);
#11496=VERTEX_POINT('',#52791);
#11497=VERTEX_POINT('',#52795);
#11498=VERTEX_POINT('',#52797);
#11499=VERTEX_POINT('',#52803);
#11500=VERTEX_POINT('',#52809);
#11501=VERTEX_POINT('',#52810);
#11502=VERTEX_POINT('',#52812);
#11503=VERTEX_POINT('',#52816);
#11504=VERTEX_POINT('',#52818);
#11505=VERTEX_POINT('',#52824);
#11506=VERTEX_POINT('',#52830);
#11507=VERTEX_POINT('',#52831);
#11508=VERTEX_POINT('',#52833);
#11509=VERTEX_POINT('',#52837);
#11510=VERTEX_POINT('',#52839);
#11511=VERTEX_POINT('',#52845);
#11512=VERTEX_POINT('',#52851);
#11513=VERTEX_POINT('',#52852);
#11514=VERTEX_POINT('',#52854);
#11515=VERTEX_POINT('',#52858);
#11516=VERTEX_POINT('',#52860);
#11517=VERTEX_POINT('',#52866);
#11518=VERTEX_POINT('',#52872);
#11519=VERTEX_POINT('',#52873);
#11520=VERTEX_POINT('',#52875);
#11521=VERTEX_POINT('',#52879);
#11522=VERTEX_POINT('',#52881);
#11523=VERTEX_POINT('',#52887);
#11524=VERTEX_POINT('',#52893);
#11525=VERTEX_POINT('',#52894);
#11526=VERTEX_POINT('',#52896);
#11527=VERTEX_POINT('',#52900);
#11528=VERTEX_POINT('',#52902);
#11529=VERTEX_POINT('',#52908);
#11530=VERTEX_POINT('',#52914);
#11531=VERTEX_POINT('',#52915);
#11532=VERTEX_POINT('',#52917);
#11533=VERTEX_POINT('',#52921);
#11534=VERTEX_POINT('',#52923);
#11535=VERTEX_POINT('',#52929);
#11536=VERTEX_POINT('',#52935);
#11537=VERTEX_POINT('',#52936);
#11538=VERTEX_POINT('',#52938);
#11539=VERTEX_POINT('',#52942);
#11540=VERTEX_POINT('',#52944);
#11541=VERTEX_POINT('',#52950);
#11542=VERTEX_POINT('',#52956);
#11543=VERTEX_POINT('',#52957);
#11544=VERTEX_POINT('',#52959);
#11545=VERTEX_POINT('',#52963);
#11546=VERTEX_POINT('',#52965);
#11547=VERTEX_POINT('',#52971);
#11548=VERTEX_POINT('',#52977);
#11549=VERTEX_POINT('',#52978);
#11550=VERTEX_POINT('',#52980);
#11551=VERTEX_POINT('',#52984);
#11552=VERTEX_POINT('',#52986);
#11553=VERTEX_POINT('',#52992);
#11554=VERTEX_POINT('',#52998);
#11555=VERTEX_POINT('',#52999);
#11556=VERTEX_POINT('',#53001);
#11557=VERTEX_POINT('',#53005);
#11558=VERTEX_POINT('',#53007);
#11559=VERTEX_POINT('',#53013);
#11560=VERTEX_POINT('',#53019);
#11561=VERTEX_POINT('',#53020);
#11562=VERTEX_POINT('',#53022);
#11563=VERTEX_POINT('',#53026);
#11564=VERTEX_POINT('',#53028);
#11565=VERTEX_POINT('',#53034);
#11566=VERTEX_POINT('',#53040);
#11567=VERTEX_POINT('',#53041);
#11568=VERTEX_POINT('',#53043);
#11569=VERTEX_POINT('',#53047);
#11570=VERTEX_POINT('',#53049);
#11571=VERTEX_POINT('',#53055);
#11572=VERTEX_POINT('',#53061);
#11573=VERTEX_POINT('',#53062);
#11574=VERTEX_POINT('',#53064);
#11575=VERTEX_POINT('',#53068);
#11576=VERTEX_POINT('',#53070);
#11577=VERTEX_POINT('',#53076);
#11578=VERTEX_POINT('',#53082);
#11579=VERTEX_POINT('',#53083);
#11580=VERTEX_POINT('',#53085);
#11581=VERTEX_POINT('',#53087);
#11582=VERTEX_POINT('',#53091);
#11583=VERTEX_POINT('',#53093);
#11584=VERTEX_POINT('',#53099);
#11585=VERTEX_POINT('',#53105);
#11586=VERTEX_POINT('',#53106);
#11587=VERTEX_POINT('',#53108);
#11588=VERTEX_POINT('',#53112);
#11589=VERTEX_POINT('',#53114);
#11590=VERTEX_POINT('',#53120);
#11591=VERTEX_POINT('',#53126);
#11592=VERTEX_POINT('',#53127);
#11593=VERTEX_POINT('',#53129);
#11594=VERTEX_POINT('',#53133);
#11595=VERTEX_POINT('',#53135);
#11596=VERTEX_POINT('',#53141);
#11597=VERTEX_POINT('',#53147);
#11598=VERTEX_POINT('',#53148);
#11599=VERTEX_POINT('',#53150);
#11600=VERTEX_POINT('',#53154);
#11601=VERTEX_POINT('',#53156);
#11602=VERTEX_POINT('',#53162);
#11603=VERTEX_POINT('',#53168);
#11604=VERTEX_POINT('',#53169);
#11605=VERTEX_POINT('',#53171);
#11606=VERTEX_POINT('',#53175);
#11607=VERTEX_POINT('',#53177);
#11608=VERTEX_POINT('',#53183);
#11609=VERTEX_POINT('',#53189);
#11610=VERTEX_POINT('',#53190);
#11611=VERTEX_POINT('',#53192);
#11612=VERTEX_POINT('',#53196);
#11613=VERTEX_POINT('',#53198);
#11614=VERTEX_POINT('',#53204);
#11615=VERTEX_POINT('',#53210);
#11616=VERTEX_POINT('',#53211);
#11617=VERTEX_POINT('',#53213);
#11618=VERTEX_POINT('',#53217);
#11619=VERTEX_POINT('',#53219);
#11620=VERTEX_POINT('',#53225);
#11621=VERTEX_POINT('',#53231);
#11622=VERTEX_POINT('',#53232);
#11623=VERTEX_POINT('',#53234);
#11624=VERTEX_POINT('',#53238);
#11625=VERTEX_POINT('',#53240);
#11626=VERTEX_POINT('',#53246);
#11627=VERTEX_POINT('',#53252);
#11628=VERTEX_POINT('',#53253);
#11629=VERTEX_POINT('',#53255);
#11630=VERTEX_POINT('',#53259);
#11631=VERTEX_POINT('',#53261);
#11632=VERTEX_POINT('',#53267);
#11633=VERTEX_POINT('',#53273);
#11634=VERTEX_POINT('',#53274);
#11635=VERTEX_POINT('',#53276);
#11636=VERTEX_POINT('',#53280);
#11637=VERTEX_POINT('',#53282);
#11638=VERTEX_POINT('',#53288);
#11639=VERTEX_POINT('',#53294);
#11640=VERTEX_POINT('',#53295);
#11641=VERTEX_POINT('',#53297);
#11642=VERTEX_POINT('',#53301);
#11643=VERTEX_POINT('',#53303);
#11644=VERTEX_POINT('',#53309);
#11645=VERTEX_POINT('',#53315);
#11646=VERTEX_POINT('',#53316);
#11647=VERTEX_POINT('',#53318);
#11648=VERTEX_POINT('',#53322);
#11649=VERTEX_POINT('',#53324);
#11650=VERTEX_POINT('',#53330);
#11651=VERTEX_POINT('',#53336);
#11652=VERTEX_POINT('',#53337);
#11653=VERTEX_POINT('',#53339);
#11654=VERTEX_POINT('',#53343);
#11655=VERTEX_POINT('',#53345);
#11656=VERTEX_POINT('',#53351);
#11657=VERTEX_POINT('',#53357);
#11658=VERTEX_POINT('',#53358);
#11659=VERTEX_POINT('',#53360);
#11660=VERTEX_POINT('',#53364);
#11661=VERTEX_POINT('',#53366);
#11662=VERTEX_POINT('',#53372);
#11663=VERTEX_POINT('',#53378);
#11664=VERTEX_POINT('',#53379);
#11665=VERTEX_POINT('',#53381);
#11666=VERTEX_POINT('',#53385);
#11667=VERTEX_POINT('',#53387);
#11668=VERTEX_POINT('',#53393);
#11669=VERTEX_POINT('',#53399);
#11670=VERTEX_POINT('',#53400);
#11671=VERTEX_POINT('',#53402);
#11672=VERTEX_POINT('',#53406);
#11673=VERTEX_POINT('',#53408);
#11674=VERTEX_POINT('',#53414);
#11675=VERTEX_POINT('',#53420);
#11676=VERTEX_POINT('',#53421);
#11677=VERTEX_POINT('',#53423);
#11678=VERTEX_POINT('',#53427);
#11679=VERTEX_POINT('',#53429);
#11680=VERTEX_POINT('',#53435);
#11681=VERTEX_POINT('',#53441);
#11682=VERTEX_POINT('',#53442);
#11683=VERTEX_POINT('',#53444);
#11684=VERTEX_POINT('',#53448);
#11685=VERTEX_POINT('',#53450);
#11686=VERTEX_POINT('',#53456);
#11687=VERTEX_POINT('',#53479);
#11688=VERTEX_POINT('',#53499);
#11689=VERTEX_POINT('',#53501);
#11690=VERTEX_POINT('',#53503);
#11691=VERTEX_POINT('',#53505);
#11692=VERTEX_POINT('',#53509);
#11693=VERTEX_POINT('',#53511);
#11694=VERTEX_POINT('',#53523);
#11695=VERTEX_POINT('',#53527);
#11696=VERTEX_POINT('',#53528);
#11697=VERTEX_POINT('',#53532);
#11698=VERTEX_POINT('',#53533);
#11699=VERTEX_POINT('',#53535);
#11700=VERTEX_POINT('',#53537);
#11701=VERTEX_POINT('',#53541);
#11702=VERTEX_POINT('',#53543);
#11703=VERTEX_POINT('',#53547);
#11704=VERTEX_POINT('',#53549);
#11705=VERTEX_POINT('',#53553);
#11706=VERTEX_POINT('',#53555);
#11707=VERTEX_POINT('',#53559);
#11708=VERTEX_POINT('',#53561);
#11709=VERTEX_POINT('',#53569);
#11710=VERTEX_POINT('',#53576);
#14586=EDGE_CURVE('',#11391,#11392,#7456,.T.);
#14587=EDGE_CURVE('',#11391,#11393,#797,.T.);
#14588=EDGE_CURVE('',#11393,#11394,#5766,.T.);
#14589=EDGE_CURVE('',#11394,#11395,#7457,.T.);
#14590=EDGE_CURVE('',#11395,#11395,#5767,.T.);
#14591=EDGE_CURVE('',#11394,#11396,#5768,.T.);
#14592=EDGE_CURVE('',#11396,#11392,#798,.T.);
#14593=EDGE_CURVE('',#11397,#11398,#7458,.T.);
#14594=EDGE_CURVE('',#11397,#11391,#799,.T.);
#14595=EDGE_CURVE('',#11392,#11398,#800,.T.);
#14596=EDGE_CURVE('',#11399,#11400,#7459,.T.);
#14597=EDGE_CURVE('',#11399,#11397,#801,.T.);
#14598=EDGE_CURVE('',#11398,#11400,#802,.T.);
#14599=EDGE_CURVE('',#11401,#11402,#7460,.T.);
#14600=EDGE_CURVE('',#11401,#11399,#803,.T.);
#14601=EDGE_CURVE('',#11400,#11402,#804,.T.);
#14602=EDGE_CURVE('',#11403,#11404,#7461,.T.);
#14603=EDGE_CURVE('',#11403,#11401,#805,.T.);
#14604=EDGE_CURVE('',#11402,#11404,#806,.T.);
#14605=EDGE_CURVE('',#11405,#11406,#7462,.T.);
#14606=EDGE_CURVE('',#11405,#11403,#807,.T.);
#14607=EDGE_CURVE('',#11404,#11406,#808,.T.);
#14608=EDGE_CURVE('',#11407,#11408,#7463,.T.);
#14609=EDGE_CURVE('',#11407,#11405,#809,.T.);
#14610=EDGE_CURVE('',#11406,#11408,#810,.T.);
#14611=EDGE_CURVE('',#11409,#11410,#7464,.T.);
#14612=EDGE_CURVE('',#11409,#11407,#811,.T.);
#14613=EDGE_CURVE('',#11408,#11410,#812,.T.);
#14614=EDGE_CURVE('',#11411,#11412,#7465,.T.);
#14615=EDGE_CURVE('',#11411,#11409,#813,.T.);
#14616=EDGE_CURVE('',#11410,#11412,#814,.T.);
#14617=EDGE_CURVE('',#11413,#11414,#7466,.T.);
#14618=EDGE_CURVE('',#11413,#11411,#815,.T.);
#14619=EDGE_CURVE('',#11412,#11414,#816,.T.);
#14620=EDGE_CURVE('',#11415,#11416,#7467,.T.);
#14621=EDGE_CURVE('',#11415,#11413,#817,.T.);
#14622=EDGE_CURVE('',#11414,#11416,#818,.T.);
#14623=EDGE_CURVE('',#11417,#11418,#7468,.T.);
#14624=EDGE_CURVE('',#11417,#11415,#819,.T.);
#14625=EDGE_CURVE('',#11416,#11418,#820,.T.);
#14626=EDGE_CURVE('',#11419,#11420,#7469,.T.);
#14627=EDGE_CURVE('',#11419,#11417,#821,.T.);
#14628=EDGE_CURVE('',#11418,#11420,#822,.T.);
#14629=EDGE_CURVE('',#11421,#11422,#7470,.T.);
#14630=EDGE_CURVE('',#11421,#11419,#823,.T.);
#14631=EDGE_CURVE('',#11420,#11422,#824,.T.);
#14632=EDGE_CURVE('',#11423,#11424,#7471,.T.);
#14633=EDGE_CURVE('',#11423,#11421,#825,.T.);
#14634=EDGE_CURVE('',#11422,#11424,#826,.T.);
#14635=EDGE_CURVE('',#11425,#11426,#7472,.T.);
#14636=EDGE_CURVE('',#11425,#11423,#827,.T.);
#14637=EDGE_CURVE('',#11424,#11426,#828,.T.);
#14638=EDGE_CURVE('',#11427,#11428,#7473,.T.);
#14639=EDGE_CURVE('',#11427,#11425,#829,.T.);
#14640=EDGE_CURVE('',#11426,#11428,#830,.T.);
#14641=EDGE_CURVE('',#11429,#11430,#7474,.T.);
#14642=EDGE_CURVE('',#11429,#11427,#831,.T.);
#14643=EDGE_CURVE('',#11428,#11430,#832,.T.);
#14644=EDGE_CURVE('',#11431,#11432,#7475,.T.);
#14645=EDGE_CURVE('',#11431,#11433,#833,.T.);
#14646=EDGE_CURVE('',#11434,#11433,#5769,.T.);
#14647=EDGE_CURVE('',#11432,#11434,#834,.T.);
#14648=EDGE_CURVE('',#11435,#11436,#7476,.T.);
#14649=EDGE_CURVE('',#11435,#11431,#835,.T.);
#14650=EDGE_CURVE('',#11436,#11432,#836,.T.);
#14651=EDGE_CURVE('',#11437,#11438,#7477,.T.);
#14652=EDGE_CURVE('',#11437,#11435,#837,.T.);
#14653=EDGE_CURVE('',#11438,#11436,#838,.T.);
#14654=EDGE_CURVE('',#11439,#11440,#7478,.T.);
#14655=EDGE_CURVE('',#11439,#11437,#839,.T.);
#14656=EDGE_CURVE('',#11440,#11438,#840,.T.);
#14657=EDGE_CURVE('',#11441,#11442,#7479,.T.);
#14658=EDGE_CURVE('',#11441,#11439,#841,.T.);
#14659=EDGE_CURVE('',#11442,#11440,#842,.T.);
#14660=EDGE_CURVE('',#11443,#11444,#7480,.T.);
#14661=EDGE_CURVE('',#11443,#11441,#843,.T.);
#14662=EDGE_CURVE('',#11444,#11442,#844,.T.);
#14663=EDGE_CURVE('',#11445,#11446,#7481,.T.);
#14664=EDGE_CURVE('',#11445,#11443,#845,.T.);
#14665=EDGE_CURVE('',#11446,#11444,#846,.T.);
#14666=EDGE_CURVE('',#11447,#11448,#7482,.T.);
#14667=EDGE_CURVE('',#11447,#11445,#847,.T.);
#14668=EDGE_CURVE('',#11448,#11446,#848,.T.);
#14669=EDGE_CURVE('',#11449,#11450,#7483,.T.);
#14670=EDGE_CURVE('',#11449,#11447,#849,.T.);
#14671=EDGE_CURVE('',#11450,#11448,#850,.T.);
#14672=EDGE_CURVE('',#11451,#11452,#7484,.T.);
#14673=EDGE_CURVE('',#11451,#11449,#851,.T.);
#14674=EDGE_CURVE('',#11452,#11450,#852,.T.);
#14675=EDGE_CURVE('',#11453,#11454,#7485,.T.);
#14676=EDGE_CURVE('',#11453,#11451,#853,.T.);
#14677=EDGE_CURVE('',#11454,#11452,#854,.T.);
#14678=EDGE_CURVE('',#11455,#11456,#7486,.T.);
#14679=EDGE_CURVE('',#11455,#11453,#855,.T.);
#14680=EDGE_CURVE('',#11456,#11454,#856,.T.);
#14681=EDGE_CURVE('',#11457,#11458,#7487,.T.);
#14682=EDGE_CURVE('',#11457,#11455,#857,.T.);
#14683=EDGE_CURVE('',#11458,#11456,#858,.T.);
#14684=EDGE_CURVE('',#11459,#11460,#7488,.T.);
#14685=EDGE_CURVE('',#11459,#11457,#859,.T.);
#14686=EDGE_CURVE('',#11460,#11458,#860,.T.);
#14687=EDGE_CURVE('',#11461,#11462,#7489,.T.);
#14688=EDGE_CURVE('',#11461,#11459,#861,.T.);
#14689=EDGE_CURVE('',#11462,#11460,#862,.T.);
#14690=EDGE_CURVE('',#11463,#11464,#7490,.T.);
#14691=EDGE_CURVE('',#11463,#11461,#863,.T.);
#14692=EDGE_CURVE('',#11464,#11462,#864,.T.);
#14693=EDGE_CURVE('',#11465,#11466,#7491,.T.);
#14694=EDGE_CURVE('',#11465,#11463,#865,.T.);
#14695=EDGE_CURVE('',#11466,#11464,#866,.T.);
#14696=EDGE_CURVE('',#11467,#11468,#7492,.T.);
#14697=EDGE_CURVE('',#11467,#11465,#867,.T.);
#14698=EDGE_CURVE('',#11468,#11466,#868,.T.);
#14699=EDGE_CURVE('',#11469,#11470,#7493,.T.);
#14700=EDGE_CURVE('',#11469,#11467,#869,.T.);
#14701=EDGE_CURVE('',#11470,#11468,#870,.T.);
#14702=EDGE_CURVE('',#11433,#11471,#871,.T.);
#14703=EDGE_CURVE('',#11472,#11471,#5770,.T.);
#14704=EDGE_CURVE('',#11473,#11472,#5771,.T.);
#14705=EDGE_CURVE('',#11473,#11434,#872,.T.);
#14706=EDGE_CURVE('',#11430,#11473,#873,.T.);
#14707=EDGE_CURVE('',#11474,#11396,#874,.T.);
#14708=EDGE_CURVE('',#11474,#11470,#875,.T.);
#14709=EDGE_CURVE('',#11393,#11475,#876,.T.);
#14710=EDGE_CURVE('',#11475,#11474,#5772,.T.);
#14711=EDGE_CURVE('',#11475,#11469,#877,.T.);
#14712=EDGE_CURVE('',#11471,#11429,#878,.T.);
#14713=EDGE_CURVE('',#11476,#11477,#5773,.T.);
#14714=EDGE_CURVE('',#11476,#11478,#7494,.T.);
#14715=EDGE_CURVE('',#11478,#11477,#7495,.T.);
#14716=EDGE_CURVE('',#11477,#11479,#7496,.T.);
#14717=EDGE_CURVE('',#11478,#11480,#7497,.T.);
#14718=EDGE_CURVE('',#11479,#11480,#291,.T.);
#14719=EDGE_CURVE('',#11481,#11476,#7498,.T.);
#14720=EDGE_CURVE('',#11480,#11481,#292,.T.);
#14721=EDGE_CURVE('',#11482,#11483,#5774,.T.);
#14722=EDGE_CURVE('',#11482,#11484,#7499,.T.);
#14723=EDGE_CURVE('',#11484,#11483,#7500,.T.);
#14724=EDGE_CURVE('',#11483,#11485,#7501,.T.);
#14725=EDGE_CURVE('',#11484,#11486,#7502,.T.);
#14726=EDGE_CURVE('',#11485,#11486,#293,.T.);
#14727=EDGE_CURVE('',#11487,#11482,#7503,.T.);
#14728=EDGE_CURVE('',#11486,#11487,#294,.T.);
#14729=EDGE_CURVE('',#11488,#11489,#5775,.T.);
#14730=EDGE_CURVE('',#11488,#11490,#7504,.T.);
#14731=EDGE_CURVE('',#11490,#11489,#7505,.T.);
#14732=EDGE_CURVE('',#11489,#11491,#7506,.T.);
#14733=EDGE_CURVE('',#11490,#11492,#7507,.T.);
#14734=EDGE_CURVE('',#11491,#11492,#295,.T.);
#14735=EDGE_CURVE('',#11493,#11488,#7508,.T.);
#14736=EDGE_CURVE('',#11492,#11493,#296,.T.);
#14737=EDGE_CURVE('',#11494,#11495,#5776,.T.);
#14738=EDGE_CURVE('',#11494,#11496,#7509,.T.);
#14739=EDGE_CURVE('',#11496,#11495,#7510,.T.);
#14740=EDGE_CURVE('',#11495,#11497,#7511,.T.);
#14741=EDGE_CURVE('',#11496,#11498,#7512,.T.);
#14742=EDGE_CURVE('',#11497,#11498,#297,.T.);
#14743=EDGE_CURVE('',#11499,#11494,#7513,.T.);
#14744=EDGE_CURVE('',#11498,#11499,#298,.T.);
#14745=EDGE_CURVE('',#11500,#11501,#5777,.T.);
#14746=EDGE_CURVE('',#11500,#11502,#7514,.T.);
#14747=EDGE_CURVE('',#11502,#11501,#7515,.T.);
#14748=EDGE_CURVE('',#11501,#11503,#7516,.T.);
#14749=EDGE_CURVE('',#11502,#11504,#7517,.T.);
#14750=EDGE_CURVE('',#11503,#11504,#299,.T.);
#14751=EDGE_CURVE('',#11505,#11500,#7518,.T.);
#14752=EDGE_CURVE('',#11504,#11505,#300,.T.);
#14753=EDGE_CURVE('',#11506,#11507,#5778,.T.);
#14754=EDGE_CURVE('',#11506,#11508,#7519,.T.);
#14755=EDGE_CURVE('',#11508,#11507,#7520,.T.);
#14756=EDGE_CURVE('',#11507,#11509,#7521,.T.);
#14757=EDGE_CURVE('',#11508,#11510,#7522,.T.);
#14758=EDGE_CURVE('',#11509,#11510,#301,.T.);
#14759=EDGE_CURVE('',#11511,#11506,#7523,.T.);
#14760=EDGE_CURVE('',#11510,#11511,#302,.T.);
#14761=EDGE_CURVE('',#11512,#11513,#5779,.T.);
#14762=EDGE_CURVE('',#11512,#11514,#7524,.T.);
#14763=EDGE_CURVE('',#11514,#11513,#7525,.T.);
#14764=EDGE_CURVE('',#11513,#11515,#7526,.T.);
#14765=EDGE_CURVE('',#11514,#11516,#7527,.T.);
#14766=EDGE_CURVE('',#11515,#11516,#303,.T.);
#14767=EDGE_CURVE('',#11517,#11512,#7528,.T.);
#14768=EDGE_CURVE('',#11516,#11517,#304,.T.);
#14769=EDGE_CURVE('',#11518,#11519,#5780,.T.);
#14770=EDGE_CURVE('',#11518,#11520,#7529,.T.);
#14771=EDGE_CURVE('',#11520,#11519,#7530,.T.);
#14772=EDGE_CURVE('',#11519,#11521,#7531,.T.);
#14773=EDGE_CURVE('',#11520,#11522,#7532,.T.);
#14774=EDGE_CURVE('',#11521,#11522,#305,.T.);
#14775=EDGE_CURVE('',#11523,#11518,#7533,.T.);
#14776=EDGE_CURVE('',#11522,#11523,#306,.T.);
#14777=EDGE_CURVE('',#11524,#11525,#5781,.T.);
#14778=EDGE_CURVE('',#11524,#11526,#7534,.T.);
#14779=EDGE_CURVE('',#11526,#11525,#7535,.T.);
#14780=EDGE_CURVE('',#11525,#11527,#7536,.T.);
#14781=EDGE_CURVE('',#11526,#11528,#7537,.T.);
#14782=EDGE_CURVE('',#11527,#11528,#307,.T.);
#14783=EDGE_CURVE('',#11529,#11524,#7538,.T.);
#14784=EDGE_CURVE('',#11528,#11529,#308,.T.);
#14785=EDGE_CURVE('',#11530,#11531,#5782,.T.);
#14786=EDGE_CURVE('',#11530,#11532,#7539,.T.);
#14787=EDGE_CURVE('',#11532,#11531,#7540,.T.);
#14788=EDGE_CURVE('',#11531,#11533,#7541,.T.);
#14789=EDGE_CURVE('',#11532,#11534,#7542,.T.);
#14790=EDGE_CURVE('',#11533,#11534,#309,.T.);
#14791=EDGE_CURVE('',#11535,#11530,#7543,.T.);
#14792=EDGE_CURVE('',#11534,#11535,#310,.T.);
#14793=EDGE_CURVE('',#11536,#11537,#5783,.T.);
#14794=EDGE_CURVE('',#11536,#11538,#7544,.T.);
#14795=EDGE_CURVE('',#11538,#11537,#7545,.T.);
#14796=EDGE_CURVE('',#11537,#11539,#7546,.T.);
#14797=EDGE_CURVE('',#11538,#11540,#7547,.T.);
#14798=EDGE_CURVE('',#11539,#11540,#311,.T.);
#14799=EDGE_CURVE('',#11541,#11536,#7548,.T.);
#14800=EDGE_CURVE('',#11540,#11541,#312,.T.);
#14801=EDGE_CURVE('',#11542,#11543,#5784,.T.);
#14802=EDGE_CURVE('',#11542,#11544,#7549,.T.);
#14803=EDGE_CURVE('',#11544,#11543,#7550,.T.);
#14804=EDGE_CURVE('',#11543,#11545,#7551,.T.);
#14805=EDGE_CURVE('',#11544,#11546,#7552,.T.);
#14806=EDGE_CURVE('',#11545,#11546,#313,.T.);
#14807=EDGE_CURVE('',#11547,#11542,#7553,.T.);
#14808=EDGE_CURVE('',#11546,#11547,#314,.T.);
#14809=EDGE_CURVE('',#11548,#11549,#5785,.T.);
#14810=EDGE_CURVE('',#11548,#11550,#7554,.T.);
#14811=EDGE_CURVE('',#11550,#11549,#7555,.T.);
#14812=EDGE_CURVE('',#11549,#11551,#7556,.T.);
#14813=EDGE_CURVE('',#11550,#11552,#7557,.T.);
#14814=EDGE_CURVE('',#11551,#11552,#315,.T.);
#14815=EDGE_CURVE('',#11553,#11548,#7558,.T.);
#14816=EDGE_CURVE('',#11552,#11553,#316,.T.);
#14817=EDGE_CURVE('',#11554,#11555,#5786,.T.);
#14818=EDGE_CURVE('',#11554,#11556,#7559,.T.);
#14819=EDGE_CURVE('',#11556,#11555,#7560,.T.);
#14820=EDGE_CURVE('',#11555,#11557,#7561,.T.);
#14821=EDGE_CURVE('',#11556,#11558,#7562,.T.);
#14822=EDGE_CURVE('',#11557,#11558,#317,.T.);
#14823=EDGE_CURVE('',#11559,#11554,#7563,.T.);
#14824=EDGE_CURVE('',#11558,#11559,#318,.T.);
#14825=EDGE_CURVE('',#11560,#11561,#5787,.T.);
#14826=EDGE_CURVE('',#11560,#11562,#7564,.T.);
#14827=EDGE_CURVE('',#11562,#11561,#7565,.T.);
#14828=EDGE_CURVE('',#11561,#11563,#7566,.T.);
#14829=EDGE_CURVE('',#11562,#11564,#7567,.T.);
#14830=EDGE_CURVE('',#11563,#11564,#319,.T.);
#14831=EDGE_CURVE('',#11565,#11560,#7568,.T.);
#14832=EDGE_CURVE('',#11564,#11565,#320,.T.);
#14833=EDGE_CURVE('',#11566,#11567,#5788,.T.);
#14834=EDGE_CURVE('',#11566,#11568,#7569,.T.);
#14835=EDGE_CURVE('',#11568,#11567,#7570,.T.);
#14836=EDGE_CURVE('',#11567,#11569,#7571,.T.);
#14837=EDGE_CURVE('',#11568,#11570,#7572,.T.);
#14838=EDGE_CURVE('',#11569,#11570,#321,.T.);
#14839=EDGE_CURVE('',#11571,#11566,#7573,.T.);
#14840=EDGE_CURVE('',#11570,#11571,#322,.T.);
#14841=EDGE_CURVE('',#11572,#11573,#5789,.T.);
#14842=EDGE_CURVE('',#11572,#11574,#7574,.T.);
#14843=EDGE_CURVE('',#11574,#11573,#7575,.T.);
#14844=EDGE_CURVE('',#11573,#11575,#7576,.T.);
#14845=EDGE_CURVE('',#11574,#11576,#7577,.T.);
#14846=EDGE_CURVE('',#11575,#11576,#323,.T.);
#14847=EDGE_CURVE('',#11577,#11572,#7578,.T.);
#14848=EDGE_CURVE('',#11576,#11577,#324,.T.);
#14849=EDGE_CURVE('',#11578,#11579,#5790,.T.);
#14850=EDGE_CURVE('',#11578,#11580,#7579,.T.);
#14851=EDGE_CURVE('',#11580,#11581,#7580,.T.);
#14852=EDGE_CURVE('',#11579,#11581,#5791,.T.);
#14853=EDGE_CURVE('',#11581,#11582,#7581,.T.);
#14854=EDGE_CURVE('',#11580,#11583,#7582,.T.);
#14855=EDGE_CURVE('',#11582,#11583,#325,.T.);
#14856=EDGE_CURVE('',#11584,#11578,#7583,.T.);
#14857=EDGE_CURVE('',#11583,#11584,#326,.T.);
#14858=EDGE_CURVE('',#11585,#11586,#5792,.T.);
#14859=EDGE_CURVE('',#11585,#11587,#7584,.T.);
#14860=EDGE_CURVE('',#11587,#11586,#7585,.T.);
#14861=EDGE_CURVE('',#11586,#11588,#7586,.T.);
#14862=EDGE_CURVE('',#11587,#11589,#7587,.T.);
#14863=EDGE_CURVE('',#11588,#11589,#327,.T.);
#14864=EDGE_CURVE('',#11590,#11585,#7588,.T.);
#14865=EDGE_CURVE('',#11589,#11590,#328,.T.);
#14866=EDGE_CURVE('',#11591,#11592,#5793,.T.);
#14867=EDGE_CURVE('',#11591,#11593,#7589,.T.);
#14868=EDGE_CURVE('',#11593,#11592,#7590,.T.);
#14869=EDGE_CURVE('',#11592,#11594,#7591,.T.);
#14870=EDGE_CURVE('',#11593,#11595,#7592,.T.);
#14871=EDGE_CURVE('',#11594,#11595,#329,.T.);
#14872=EDGE_CURVE('',#11596,#11591,#7593,.T.);
#14873=EDGE_CURVE('',#11595,#11596,#330,.T.);
#14874=EDGE_CURVE('',#11597,#11598,#5794,.T.);
#14875=EDGE_CURVE('',#11597,#11599,#7594,.T.);
#14876=EDGE_CURVE('',#11599,#11598,#7595,.T.);
#14877=EDGE_CURVE('',#11598,#11600,#7596,.T.);
#14878=EDGE_CURVE('',#11599,#11601,#7597,.T.);
#14879=EDGE_CURVE('',#11600,#11601,#331,.T.);
#14880=EDGE_CURVE('',#11602,#11597,#7598,.T.);
#14881=EDGE_CURVE('',#11601,#11602,#332,.T.);
#14882=EDGE_CURVE('',#11603,#11604,#5795,.T.);
#14883=EDGE_CURVE('',#11603,#11605,#7599,.T.);
#14884=EDGE_CURVE('',#11605,#11604,#7600,.T.);
#14885=EDGE_CURVE('',#11604,#11606,#7601,.T.);
#14886=EDGE_CURVE('',#11605,#11607,#7602,.T.);
#14887=EDGE_CURVE('',#11606,#11607,#333,.T.);
#14888=EDGE_CURVE('',#11608,#11603,#7603,.T.);
#14889=EDGE_CURVE('',#11607,#11608,#334,.T.);
#14890=EDGE_CURVE('',#11609,#11610,#5796,.T.);
#14891=EDGE_CURVE('',#11609,#11611,#7604,.T.);
#14892=EDGE_CURVE('',#11611,#11610,#7605,.T.);
#14893=EDGE_CURVE('',#11610,#11612,#7606,.T.);
#14894=EDGE_CURVE('',#11611,#11613,#7607,.T.);
#14895=EDGE_CURVE('',#11612,#11613,#335,.T.);
#14896=EDGE_CURVE('',#11614,#11609,#7608,.T.);
#14897=EDGE_CURVE('',#11613,#11614,#336,.T.);
#14898=EDGE_CURVE('',#11615,#11616,#5797,.T.);
#14899=EDGE_CURVE('',#11615,#11617,#7609,.T.);
#14900=EDGE_CURVE('',#11617,#11616,#7610,.T.);
#14901=EDGE_CURVE('',#11616,#11618,#7611,.T.);
#14902=EDGE_CURVE('',#11617,#11619,#7612,.T.);
#14903=EDGE_CURVE('',#11618,#11619,#337,.T.);
#14904=EDGE_CURVE('',#11620,#11615,#7613,.T.);
#14905=EDGE_CURVE('',#11619,#11620,#338,.T.);
#14906=EDGE_CURVE('',#11621,#11622,#5798,.T.);
#14907=EDGE_CURVE('',#11621,#11623,#7614,.T.);
#14908=EDGE_CURVE('',#11623,#11622,#7615,.T.);
#14909=EDGE_CURVE('',#11622,#11624,#7616,.T.);
#14910=EDGE_CURVE('',#11623,#11625,#7617,.T.);
#14911=EDGE_CURVE('',#11624,#11625,#339,.T.);
#14912=EDGE_CURVE('',#11626,#11621,#7618,.T.);
#14913=EDGE_CURVE('',#11625,#11626,#340,.T.);
#14914=EDGE_CURVE('',#11627,#11628,#5799,.T.);
#14915=EDGE_CURVE('',#11627,#11629,#7619,.T.);
#14916=EDGE_CURVE('',#11629,#11628,#7620,.T.);
#14917=EDGE_CURVE('',#11628,#11630,#7621,.T.);
#14918=EDGE_CURVE('',#11629,#11631,#7622,.T.);
#14919=EDGE_CURVE('',#11630,#11631,#341,.T.);
#14920=EDGE_CURVE('',#11632,#11627,#7623,.T.);
#14921=EDGE_CURVE('',#11631,#11632,#342,.T.);
#14922=EDGE_CURVE('',#11633,#11634,#5800,.T.);
#14923=EDGE_CURVE('',#11633,#11635,#7624,.T.);
#14924=EDGE_CURVE('',#11635,#11634,#7625,.T.);
#14925=EDGE_CURVE('',#11634,#11636,#7626,.T.);
#14926=EDGE_CURVE('',#11635,#11637,#7627,.T.);
#14927=EDGE_CURVE('',#11636,#11637,#343,.T.);
#14928=EDGE_CURVE('',#11638,#11633,#7628,.T.);
#14929=EDGE_CURVE('',#11637,#11638,#344,.T.);
#14930=EDGE_CURVE('',#11639,#11640,#5801,.T.);
#14931=EDGE_CURVE('',#11639,#11641,#7629,.T.);
#14932=EDGE_CURVE('',#11641,#11640,#7630,.T.);
#14933=EDGE_CURVE('',#11640,#11642,#7631,.T.);
#14934=EDGE_CURVE('',#11641,#11643,#7632,.T.);
#14935=EDGE_CURVE('',#11642,#11643,#345,.T.);
#14936=EDGE_CURVE('',#11644,#11639,#7633,.T.);
#14937=EDGE_CURVE('',#11643,#11644,#346,.T.);
#14938=EDGE_CURVE('',#11645,#11646,#5802,.T.);
#14939=EDGE_CURVE('',#11645,#11647,#7634,.T.);
#14940=EDGE_CURVE('',#11647,#11646,#7635,.T.);
#14941=EDGE_CURVE('',#11646,#11648,#7636,.T.);
#14942=EDGE_CURVE('',#11647,#11649,#7637,.T.);
#14943=EDGE_CURVE('',#11648,#11649,#347,.T.);
#14944=EDGE_CURVE('',#11650,#11645,#7638,.T.);
#14945=EDGE_CURVE('',#11649,#11650,#348,.T.);
#14946=EDGE_CURVE('',#11651,#11652,#5803,.T.);
#14947=EDGE_CURVE('',#11651,#11653,#7639,.T.);
#14948=EDGE_CURVE('',#11653,#11652,#7640,.T.);
#14949=EDGE_CURVE('',#11652,#11654,#7641,.T.);
#14950=EDGE_CURVE('',#11653,#11655,#7642,.T.);
#14951=EDGE_CURVE('',#11654,#11655,#349,.T.);
#14952=EDGE_CURVE('',#11656,#11651,#7643,.T.);
#14953=EDGE_CURVE('',#11655,#11656,#350,.T.);
#14954=EDGE_CURVE('',#11657,#11658,#5804,.T.);
#14955=EDGE_CURVE('',#11657,#11659,#7644,.T.);
#14956=EDGE_CURVE('',#11659,#11658,#7645,.T.);
#14957=EDGE_CURVE('',#11658,#11660,#7646,.T.);
#14958=EDGE_CURVE('',#11659,#11661,#7647,.T.);
#14959=EDGE_CURVE('',#11660,#11661,#351,.T.);
#14960=EDGE_CURVE('',#11662,#11657,#7648,.T.);
#14961=EDGE_CURVE('',#11661,#11662,#352,.T.);
#14962=EDGE_CURVE('',#11663,#11664,#5805,.T.);
#14963=EDGE_CURVE('',#11663,#11665,#7649,.T.);
#14964=EDGE_CURVE('',#11665,#11664,#7650,.T.);
#14965=EDGE_CURVE('',#11664,#11666,#7651,.T.);
#14966=EDGE_CURVE('',#11665,#11667,#7652,.T.);
#14967=EDGE_CURVE('',#11666,#11667,#353,.T.);
#14968=EDGE_CURVE('',#11668,#11663,#7653,.T.);
#14969=EDGE_CURVE('',#11667,#11668,#354,.T.);
#14970=EDGE_CURVE('',#11669,#11670,#5806,.T.);
#14971=EDGE_CURVE('',#11669,#11671,#7654,.T.);
#14972=EDGE_CURVE('',#11671,#11670,#7655,.T.);
#14973=EDGE_CURVE('',#11670,#11672,#7656,.T.);
#14974=EDGE_CURVE('',#11671,#11673,#7657,.T.);
#14975=EDGE_CURVE('',#11672,#11673,#355,.T.);
#14976=EDGE_CURVE('',#11674,#11669,#7658,.T.);
#14977=EDGE_CURVE('',#11673,#11674,#356,.T.);
#14978=EDGE_CURVE('',#11675,#11676,#5807,.T.);
#14979=EDGE_CURVE('',#11675,#11677,#7659,.T.);
#14980=EDGE_CURVE('',#11677,#11676,#7660,.T.);
#14981=EDGE_CURVE('',#11676,#11678,#7661,.T.);
#14982=EDGE_CURVE('',#11677,#11679,#7662,.T.);
#14983=EDGE_CURVE('',#11678,#11679,#357,.T.);
#14984=EDGE_CURVE('',#11680,#11675,#7663,.T.);
#14985=EDGE_CURVE('',#11679,#11680,#358,.T.);
#14986=EDGE_CURVE('',#11681,#11682,#5808,.T.);
#14987=EDGE_CURVE('',#11681,#11683,#7664,.T.);
#14988=EDGE_CURVE('',#11683,#11682,#7665,.T.);
#14989=EDGE_CURVE('',#11682,#11684,#7666,.T.);
#14990=EDGE_CURVE('',#11683,#11685,#7667,.T.);
#14991=EDGE_CURVE('',#11684,#11685,#359,.T.);
#14992=EDGE_CURVE('',#11686,#11681,#7668,.T.);
#14993=EDGE_CURVE('',#11685,#11686,#360,.T.);
#14994=EDGE_CURVE('',#11487,#11479,#5809,.T.);
#14995=EDGE_CURVE('',#11493,#11485,#5810,.T.);
#14996=EDGE_CURVE('',#11499,#11491,#5811,.T.);
#14997=EDGE_CURVE('',#11505,#11497,#5812,.T.);
#14998=EDGE_CURVE('',#11511,#11503,#5813,.T.);
#14999=EDGE_CURVE('',#11517,#11509,#5814,.T.);
#15000=EDGE_CURVE('',#11523,#11515,#5815,.T.);
#15001=EDGE_CURVE('',#11529,#11521,#5816,.T.);
#15002=EDGE_CURVE('',#11535,#11527,#5817,.T.);
#15003=EDGE_CURVE('',#11541,#11533,#5818,.T.);
#15004=EDGE_CURVE('',#11547,#11539,#5819,.T.);
#15005=EDGE_CURVE('',#11553,#11545,#5820,.T.);
#15006=EDGE_CURVE('',#11559,#11551,#5821,.T.);
#15007=EDGE_CURVE('',#11565,#11557,#5822,.T.);
#15008=EDGE_CURVE('',#11571,#11563,#5823,.T.);
#15009=EDGE_CURVE('',#11577,#11569,#5824,.T.);
#15010=EDGE_CURVE('',#11584,#11575,#5825,.T.);
#15011=EDGE_CURVE('',#11579,#11687,#7669,.T.);
#15012=EDGE_CURVE('',#11687,#11687,#5826,.T.);
#15013=EDGE_CURVE('',#11590,#11582,#5827,.T.);
#15014=EDGE_CURVE('',#11596,#11588,#5828,.T.);
#15015=EDGE_CURVE('',#11602,#11594,#5829,.T.);
#15016=EDGE_CURVE('',#11608,#11600,#5830,.T.);
#15017=EDGE_CURVE('',#11614,#11606,#5831,.T.);
#15018=EDGE_CURVE('',#11620,#11612,#5832,.T.);
#15019=EDGE_CURVE('',#11626,#11618,#5833,.T.);
#15020=EDGE_CURVE('',#11632,#11624,#5834,.T.);
#15021=EDGE_CURVE('',#11638,#11630,#5835,.T.);
#15022=EDGE_CURVE('',#11644,#11636,#5836,.T.);
#15023=EDGE_CURVE('',#11650,#11642,#5837,.T.);
#15024=EDGE_CURVE('',#11656,#11648,#5838,.T.);
#15025=EDGE_CURVE('',#11662,#11654,#5839,.T.);
#15026=EDGE_CURVE('',#11668,#11660,#5840,.T.);
#15027=EDGE_CURVE('',#11674,#11666,#5841,.T.);
#15028=EDGE_CURVE('',#11680,#11672,#5842,.T.);
#15029=EDGE_CURVE('',#11686,#11678,#5843,.T.);
#15030=EDGE_CURVE('',#11688,#11684,#5844,.T.);
#15031=EDGE_CURVE('',#11688,#11689,#7670,.T.);
#15032=EDGE_CURVE('',#11689,#11690,#5845,.T.);
#15033=EDGE_CURVE('',#11690,#11691,#7671,.T.);
#15034=EDGE_CURVE('',#11481,#11691,#5846,.T.);
#15035=EDGE_CURVE('',#11692,#11690,#7672,.T.);
#15036=EDGE_CURVE('',#11692,#11693,#7673,.T.);
#15037=EDGE_CURVE('',#11691,#11693,#361,.T.);
#15038=EDGE_CURVE('',#11693,#11688,#362,.T.);
#15039=EDGE_CURVE('',#11689,#11692,#7674,.T.);
#15040=EDGE_CURVE('',#11694,#11694,#5847,.T.);
#15041=EDGE_CURVE('',#11694,#11583,#7675,.T.);
#15042=EDGE_CURVE('',#11695,#11696,#7676,.T.);
#15043=EDGE_CURVE('',#11696,#11696,#5848,.T.);
#15044=EDGE_CURVE('',#11697,#11698,#7677,.T.);
#15045=EDGE_CURVE('',#11697,#11699,#7678,.T.);
#15046=EDGE_CURVE('',#11699,#11700,#7679,.T.);
#15047=EDGE_CURVE('',#11698,#11700,#7680,.T.);
#15048=EDGE_CURVE('',#11701,#11697,#7681,.T.);
#15049=EDGE_CURVE('',#11701,#11702,#7682,.T.);
#15050=EDGE_CURVE('',#11702,#11699,#7683,.T.);
#15051=EDGE_CURVE('',#11703,#11701,#7684,.T.);
#15052=EDGE_CURVE('',#11703,#11704,#7685,.T.);
#15053=EDGE_CURVE('',#11704,#11702,#7686,.T.);
#15054=EDGE_CURVE('',#11705,#11703,#7687,.T.);
#15055=EDGE_CURVE('',#11705,#11706,#7688,.T.);
#15056=EDGE_CURVE('',#11706,#11704,#7689,.T.);
#15057=EDGE_CURVE('',#11707,#11705,#7690,.T.);
#15058=EDGE_CURVE('',#11707,#11708,#7691,.T.);
#15059=EDGE_CURVE('',#11708,#11706,#7692,.T.);
#15060=EDGE_CURVE('',#11698,#11707,#7693,.T.);
#15061=EDGE_CURVE('',#11700,#11708,#7694,.T.);
#15062=EDGE_CURVE('',#11709,#11709,#5849,.T.);
#15063=EDGE_CURVE('',#11395,#11709,#7695,.T.);
#15064=EDGE_CURVE('',#11471,#11473,#5850,.T.);
#15065=EDGE_CURVE('',#11710,#11710,#5851,.T.);
#15066=EDGE_CURVE('',#11710,#11472,#7696,.T.);
#20817=ORIENTED_EDGE('',*,*,#14586,.F.);
#20818=ORIENTED_EDGE('',*,*,#14587,.T.);
#20819=ORIENTED_EDGE('',*,*,#14588,.T.);
#20820=ORIENTED_EDGE('',*,*,#14589,.T.);
#20821=ORIENTED_EDGE('',*,*,#14590,.T.);
#20822=ORIENTED_EDGE('',*,*,#14589,.F.);
#20823=ORIENTED_EDGE('',*,*,#14591,.T.);
#20824=ORIENTED_EDGE('',*,*,#14592,.T.);
#20825=ORIENTED_EDGE('',*,*,#14593,.F.);
#20826=ORIENTED_EDGE('',*,*,#14594,.T.);
#20827=ORIENTED_EDGE('',*,*,#14586,.T.);
#20828=ORIENTED_EDGE('',*,*,#14595,.T.);
#20829=ORIENTED_EDGE('',*,*,#14596,.F.);
#20830=ORIENTED_EDGE('',*,*,#14597,.T.);
#20831=ORIENTED_EDGE('',*,*,#14593,.T.);
#20832=ORIENTED_EDGE('',*,*,#14598,.T.);
#20833=ORIENTED_EDGE('',*,*,#14599,.F.);
#20834=ORIENTED_EDGE('',*,*,#14600,.T.);
#20835=ORIENTED_EDGE('',*,*,#14596,.T.);
#20836=ORIENTED_EDGE('',*,*,#14601,.T.);
#20837=ORIENTED_EDGE('',*,*,#14602,.F.);
#20838=ORIENTED_EDGE('',*,*,#14603,.T.);
#20839=ORIENTED_EDGE('',*,*,#14599,.T.);
#20840=ORIENTED_EDGE('',*,*,#14604,.T.);
#20841=ORIENTED_EDGE('',*,*,#14605,.F.);
#20842=ORIENTED_EDGE('',*,*,#14606,.T.);
#20843=ORIENTED_EDGE('',*,*,#14602,.T.);
#20844=ORIENTED_EDGE('',*,*,#14607,.T.);
#20845=ORIENTED_EDGE('',*,*,#14608,.F.);
#20846=ORIENTED_EDGE('',*,*,#14609,.T.);
#20847=ORIENTED_EDGE('',*,*,#14605,.T.);
#20848=ORIENTED_EDGE('',*,*,#14610,.T.);
#20849=ORIENTED_EDGE('',*,*,#14611,.F.);
#20850=ORIENTED_EDGE('',*,*,#14612,.T.);
#20851=ORIENTED_EDGE('',*,*,#14608,.T.);
#20852=ORIENTED_EDGE('',*,*,#14613,.T.);
#20853=ORIENTED_EDGE('',*,*,#14614,.F.);
#20854=ORIENTED_EDGE('',*,*,#14615,.T.);
#20855=ORIENTED_EDGE('',*,*,#14611,.T.);
#20856=ORIENTED_EDGE('',*,*,#14616,.T.);
#20857=ORIENTED_EDGE('',*,*,#14617,.F.);
#20858=ORIENTED_EDGE('',*,*,#14618,.T.);
#20859=ORIENTED_EDGE('',*,*,#14614,.T.);
#20860=ORIENTED_EDGE('',*,*,#14619,.T.);
#20861=ORIENTED_EDGE('',*,*,#14620,.F.);
#20862=ORIENTED_EDGE('',*,*,#14621,.T.);
#20863=ORIENTED_EDGE('',*,*,#14617,.T.);
#20864=ORIENTED_EDGE('',*,*,#14622,.T.);
#20865=ORIENTED_EDGE('',*,*,#14623,.F.);
#20866=ORIENTED_EDGE('',*,*,#14624,.T.);
#20867=ORIENTED_EDGE('',*,*,#14620,.T.);
#20868=ORIENTED_EDGE('',*,*,#14625,.T.);
#20869=ORIENTED_EDGE('',*,*,#14626,.F.);
#20870=ORIENTED_EDGE('',*,*,#14627,.T.);
#20871=ORIENTED_EDGE('',*,*,#14623,.T.);
#20872=ORIENTED_EDGE('',*,*,#14628,.T.);
#20873=ORIENTED_EDGE('',*,*,#14629,.F.);
#20874=ORIENTED_EDGE('',*,*,#14630,.T.);
#20875=ORIENTED_EDGE('',*,*,#14626,.T.);
#20876=ORIENTED_EDGE('',*,*,#14631,.T.);
#20877=ORIENTED_EDGE('',*,*,#14632,.F.);
#20878=ORIENTED_EDGE('',*,*,#14633,.T.);
#20879=ORIENTED_EDGE('',*,*,#14629,.T.);
#20880=ORIENTED_EDGE('',*,*,#14634,.T.);
#20881=ORIENTED_EDGE('',*,*,#14635,.F.);
#20882=ORIENTED_EDGE('',*,*,#14636,.T.);
#20883=ORIENTED_EDGE('',*,*,#14632,.T.);
#20884=ORIENTED_EDGE('',*,*,#14637,.T.);
#20885=ORIENTED_EDGE('',*,*,#14638,.F.);
#20886=ORIENTED_EDGE('',*,*,#14639,.T.);
#20887=ORIENTED_EDGE('',*,*,#14635,.T.);
#20888=ORIENTED_EDGE('',*,*,#14640,.T.);
#20889=ORIENTED_EDGE('',*,*,#14641,.F.);
#20890=ORIENTED_EDGE('',*,*,#14642,.T.);
#20891=ORIENTED_EDGE('',*,*,#14638,.T.);
#20892=ORIENTED_EDGE('',*,*,#14643,.T.);
#20893=ORIENTED_EDGE('',*,*,#14644,.F.);
#20894=ORIENTED_EDGE('',*,*,#14645,.T.);
#20895=ORIENTED_EDGE('',*,*,#14646,.F.);
#20896=ORIENTED_EDGE('',*,*,#14647,.F.);
#20897=ORIENTED_EDGE('',*,*,#14648,.F.);
#20898=ORIENTED_EDGE('',*,*,#14649,.T.);
#20899=ORIENTED_EDGE('',*,*,#14644,.T.);
#20900=ORIENTED_EDGE('',*,*,#14650,.F.);
#20901=ORIENTED_EDGE('',*,*,#14651,.F.);
#20902=ORIENTED_EDGE('',*,*,#14652,.T.);
#20903=ORIENTED_EDGE('',*,*,#14648,.T.);
#20904=ORIENTED_EDGE('',*,*,#14653,.F.);
#20905=ORIENTED_EDGE('',*,*,#14654,.F.);
#20906=ORIENTED_EDGE('',*,*,#14655,.T.);
#20907=ORIENTED_EDGE('',*,*,#14651,.T.);
#20908=ORIENTED_EDGE('',*,*,#14656,.F.);
#20909=ORIENTED_EDGE('',*,*,#14657,.F.);
#20910=ORIENTED_EDGE('',*,*,#14658,.T.);
#20911=ORIENTED_EDGE('',*,*,#14654,.T.);
#20912=ORIENTED_EDGE('',*,*,#14659,.F.);
#20913=ORIENTED_EDGE('',*,*,#14660,.F.);
#20914=ORIENTED_EDGE('',*,*,#14661,.T.);
#20915=ORIENTED_EDGE('',*,*,#14657,.T.);
#20916=ORIENTED_EDGE('',*,*,#14662,.F.);
#20917=ORIENTED_EDGE('',*,*,#14663,.F.);
#20918=ORIENTED_EDGE('',*,*,#14664,.T.);
#20919=ORIENTED_EDGE('',*,*,#14660,.T.);
#20920=ORIENTED_EDGE('',*,*,#14665,.F.);
#20921=ORIENTED_EDGE('',*,*,#14666,.F.);
#20922=ORIENTED_EDGE('',*,*,#14667,.T.);
#20923=ORIENTED_EDGE('',*,*,#14663,.T.);
#20924=ORIENTED_EDGE('',*,*,#14668,.F.);
#20925=ORIENTED_EDGE('',*,*,#14669,.F.);
#20926=ORIENTED_EDGE('',*,*,#14670,.T.);
#20927=ORIENTED_EDGE('',*,*,#14666,.T.);
#20928=ORIENTED_EDGE('',*,*,#14671,.F.);
#20929=ORIENTED_EDGE('',*,*,#14672,.F.);
#20930=ORIENTED_EDGE('',*,*,#14673,.T.);
#20931=ORIENTED_EDGE('',*,*,#14669,.T.);
#20932=ORIENTED_EDGE('',*,*,#14674,.F.);
#20933=ORIENTED_EDGE('',*,*,#14675,.F.);
#20934=ORIENTED_EDGE('',*,*,#14676,.T.);
#20935=ORIENTED_EDGE('',*,*,#14672,.T.);
#20936=ORIENTED_EDGE('',*,*,#14677,.F.);
#20937=ORIENTED_EDGE('',*,*,#14678,.F.);
#20938=ORIENTED_EDGE('',*,*,#14679,.T.);
#20939=ORIENTED_EDGE('',*,*,#14675,.T.);
#20940=ORIENTED_EDGE('',*,*,#14680,.F.);
#20941=ORIENTED_EDGE('',*,*,#14681,.F.);
#20942=ORIENTED_EDGE('',*,*,#14682,.T.);
#20943=ORIENTED_EDGE('',*,*,#14678,.T.);
#20944=ORIENTED_EDGE('',*,*,#14683,.F.);
#20945=ORIENTED_EDGE('',*,*,#14684,.F.);
#20946=ORIENTED_EDGE('',*,*,#14685,.T.);
#20947=ORIENTED_EDGE('',*,*,#14681,.T.);
#20948=ORIENTED_EDGE('',*,*,#14686,.F.);
#20949=ORIENTED_EDGE('',*,*,#14687,.F.);
#20950=ORIENTED_EDGE('',*,*,#14688,.T.);
#20951=ORIENTED_EDGE('',*,*,#14684,.T.);
#20952=ORIENTED_EDGE('',*,*,#14689,.F.);
#20953=ORIENTED_EDGE('',*,*,#14690,.F.);
#20954=ORIENTED_EDGE('',*,*,#14691,.T.);
#20955=ORIENTED_EDGE('',*,*,#14687,.T.);
#20956=ORIENTED_EDGE('',*,*,#14692,.F.);
#20957=ORIENTED_EDGE('',*,*,#14693,.F.);
#20958=ORIENTED_EDGE('',*,*,#14694,.T.);
#20959=ORIENTED_EDGE('',*,*,#14690,.T.);
#20960=ORIENTED_EDGE('',*,*,#14695,.F.);
#20961=ORIENTED_EDGE('',*,*,#14696,.F.);
#20962=ORIENTED_EDGE('',*,*,#14697,.T.);
#20963=ORIENTED_EDGE('',*,*,#14693,.T.);
#20964=ORIENTED_EDGE('',*,*,#14698,.F.);
#20965=ORIENTED_EDGE('',*,*,#14699,.F.);
#20966=ORIENTED_EDGE('',*,*,#14700,.T.);
#20967=ORIENTED_EDGE('',*,*,#14696,.T.);
#20968=ORIENTED_EDGE('',*,*,#14701,.F.);
#20969=ORIENTED_EDGE('',*,*,#14646,.T.);
#20970=ORIENTED_EDGE('',*,*,#14702,.T.);
#20971=ORIENTED_EDGE('',*,*,#14703,.F.);
#20972=ORIENTED_EDGE('',*,*,#14704,.F.);
#20973=ORIENTED_EDGE('',*,*,#14705,.T.);
#20974=ORIENTED_EDGE('',*,*,#14705,.F.);
#20975=ORIENTED_EDGE('',*,*,#14706,.F.);
#20976=ORIENTED_EDGE('',*,*,#14643,.F.);
#20977=ORIENTED_EDGE('',*,*,#14640,.F.);
#20978=ORIENTED_EDGE('',*,*,#14637,.F.);
#20979=ORIENTED_EDGE('',*,*,#14634,.F.);
#20980=ORIENTED_EDGE('',*,*,#14631,.F.);
#20981=ORIENTED_EDGE('',*,*,#14628,.F.);
#20982=ORIENTED_EDGE('',*,*,#14625,.F.);
#20983=ORIENTED_EDGE('',*,*,#14622,.F.);
#20984=ORIENTED_EDGE('',*,*,#14619,.F.);
#20985=ORIENTED_EDGE('',*,*,#14616,.F.);
#20986=ORIENTED_EDGE('',*,*,#14613,.F.);
#20987=ORIENTED_EDGE('',*,*,#14610,.F.);
#20988=ORIENTED_EDGE('',*,*,#14607,.F.);
#20989=ORIENTED_EDGE('',*,*,#14604,.F.);
#20990=ORIENTED_EDGE('',*,*,#14601,.F.);
#20991=ORIENTED_EDGE('',*,*,#14598,.F.);
#20992=ORIENTED_EDGE('',*,*,#14595,.F.);
#20993=ORIENTED_EDGE('',*,*,#14592,.F.);
#20994=ORIENTED_EDGE('',*,*,#14707,.F.);
#20995=ORIENTED_EDGE('',*,*,#14708,.T.);
#20996=ORIENTED_EDGE('',*,*,#14701,.T.);
#20997=ORIENTED_EDGE('',*,*,#14698,.T.);
#20998=ORIENTED_EDGE('',*,*,#14695,.T.);
#20999=ORIENTED_EDGE('',*,*,#14692,.T.);
#21000=ORIENTED_EDGE('',*,*,#14689,.T.);
#21001=ORIENTED_EDGE('',*,*,#14686,.T.);
#21002=ORIENTED_EDGE('',*,*,#14683,.T.);
#21003=ORIENTED_EDGE('',*,*,#14680,.T.);
#21004=ORIENTED_EDGE('',*,*,#14677,.T.);
#21005=ORIENTED_EDGE('',*,*,#14674,.T.);
#21006=ORIENTED_EDGE('',*,*,#14671,.T.);
#21007=ORIENTED_EDGE('',*,*,#14668,.T.);
#21008=ORIENTED_EDGE('',*,*,#14665,.T.);
#21009=ORIENTED_EDGE('',*,*,#14662,.T.);
#21010=ORIENTED_EDGE('',*,*,#14659,.T.);
#21011=ORIENTED_EDGE('',*,*,#14656,.T.);
#21012=ORIENTED_EDGE('',*,*,#14653,.T.);
#21013=ORIENTED_EDGE('',*,*,#14650,.T.);
#21014=ORIENTED_EDGE('',*,*,#14647,.T.);
#21015=ORIENTED_EDGE('',*,*,#14588,.F.);
#21016=ORIENTED_EDGE('',*,*,#14709,.T.);
#21017=ORIENTED_EDGE('',*,*,#14710,.T.);
#21018=ORIENTED_EDGE('',*,*,#14707,.T.);
#21019=ORIENTED_EDGE('',*,*,#14591,.F.);
#21020=ORIENTED_EDGE('',*,*,#14699,.T.);
#21021=ORIENTED_EDGE('',*,*,#14708,.F.);
#21022=ORIENTED_EDGE('',*,*,#14710,.F.);
#21023=ORIENTED_EDGE('',*,*,#14711,.T.);
#21024=ORIENTED_EDGE('',*,*,#14702,.F.);
#21025=ORIENTED_EDGE('',*,*,#14645,.F.);
#21026=ORIENTED_EDGE('',*,*,#14649,.F.);
#21027=ORIENTED_EDGE('',*,*,#14652,.F.);
#21028=ORIENTED_EDGE('',*,*,#14655,.F.);
#21029=ORIENTED_EDGE('',*,*,#14658,.F.);
#21030=ORIENTED_EDGE('',*,*,#14661,.F.);
#21031=ORIENTED_EDGE('',*,*,#14664,.F.);
#21032=ORIENTED_EDGE('',*,*,#14667,.F.);
#21033=ORIENTED_EDGE('',*,*,#14670,.F.);
#21034=ORIENTED_EDGE('',*,*,#14673,.F.);
#21035=ORIENTED_EDGE('',*,*,#14676,.F.);
#21036=ORIENTED_EDGE('',*,*,#14679,.F.);
#21037=ORIENTED_EDGE('',*,*,#14682,.F.);
#21038=ORIENTED_EDGE('',*,*,#14685,.F.);
#21039=ORIENTED_EDGE('',*,*,#14688,.F.);
#21040=ORIENTED_EDGE('',*,*,#14691,.F.);
#21041=ORIENTED_EDGE('',*,*,#14694,.F.);
#21042=ORIENTED_EDGE('',*,*,#14697,.F.);
#21043=ORIENTED_EDGE('',*,*,#14700,.F.);
#21044=ORIENTED_EDGE('',*,*,#14711,.F.);
#21045=ORIENTED_EDGE('',*,*,#14709,.F.);
#21046=ORIENTED_EDGE('',*,*,#14587,.F.);
#21047=ORIENTED_EDGE('',*,*,#14594,.F.);
#21048=ORIENTED_EDGE('',*,*,#14597,.F.);
#21049=ORIENTED_EDGE('',*,*,#14600,.F.);
#21050=ORIENTED_EDGE('',*,*,#14603,.F.);
#21051=ORIENTED_EDGE('',*,*,#14606,.F.);
#21052=ORIENTED_EDGE('',*,*,#14609,.F.);
#21053=ORIENTED_EDGE('',*,*,#14612,.F.);
#21054=ORIENTED_EDGE('',*,*,#14615,.F.);
#21055=ORIENTED_EDGE('',*,*,#14618,.F.);
#21056=ORIENTED_EDGE('',*,*,#14621,.F.);
#21057=ORIENTED_EDGE('',*,*,#14624,.F.);
#21058=ORIENTED_EDGE('',*,*,#14627,.F.);
#21059=ORIENTED_EDGE('',*,*,#14630,.F.);
#21060=ORIENTED_EDGE('',*,*,#14633,.F.);
#21061=ORIENTED_EDGE('',*,*,#14636,.F.);
#21062=ORIENTED_EDGE('',*,*,#14639,.F.);
#21063=ORIENTED_EDGE('',*,*,#14642,.F.);
#21064=ORIENTED_EDGE('',*,*,#14712,.F.);
#21065=ORIENTED_EDGE('',*,*,#14713,.F.);
#21066=ORIENTED_EDGE('',*,*,#14714,.T.);
#21067=ORIENTED_EDGE('',*,*,#14715,.T.);
#21068=ORIENTED_EDGE('',*,*,#14716,.F.);
#21069=ORIENTED_EDGE('',*,*,#14715,.F.);
#21070=ORIENTED_EDGE('',*,*,#14717,.T.);
#21071=ORIENTED_EDGE('',*,*,#14718,.F.);
#21072=ORIENTED_EDGE('',*,*,#14719,.F.);
#21073=ORIENTED_EDGE('',*,*,#14720,.F.);
#21074=ORIENTED_EDGE('',*,*,#14717,.F.);
#21075=ORIENTED_EDGE('',*,*,#14714,.F.);
#21076=ORIENTED_EDGE('',*,*,#14721,.F.);
#21077=ORIENTED_EDGE('',*,*,#14722,.T.);
#21078=ORIENTED_EDGE('',*,*,#14723,.T.);
#21079=ORIENTED_EDGE('',*,*,#14724,.F.);
#21080=ORIENTED_EDGE('',*,*,#14723,.F.);
#21081=ORIENTED_EDGE('',*,*,#14725,.T.);
#21082=ORIENTED_EDGE('',*,*,#14726,.F.);
#21083=ORIENTED_EDGE('',*,*,#14727,.F.);
#21084=ORIENTED_EDGE('',*,*,#14728,.F.);
#21085=ORIENTED_EDGE('',*,*,#14725,.F.);
#21086=ORIENTED_EDGE('',*,*,#14722,.F.);
#21087=ORIENTED_EDGE('',*,*,#14729,.F.);
#21088=ORIENTED_EDGE('',*,*,#14730,.T.);
#21089=ORIENTED_EDGE('',*,*,#14731,.T.);
#21090=ORIENTED_EDGE('',*,*,#14732,.F.);
#21091=ORIENTED_EDGE('',*,*,#14731,.F.);
#21092=ORIENTED_EDGE('',*,*,#14733,.T.);
#21093=ORIENTED_EDGE('',*,*,#14734,.F.);
#21094=ORIENTED_EDGE('',*,*,#14735,.F.);
#21095=ORIENTED_EDGE('',*,*,#14736,.F.);
#21096=ORIENTED_EDGE('',*,*,#14733,.F.);
#21097=ORIENTED_EDGE('',*,*,#14730,.F.);
#21098=ORIENTED_EDGE('',*,*,#14737,.F.);
#21099=ORIENTED_EDGE('',*,*,#14738,.T.);
#21100=ORIENTED_EDGE('',*,*,#14739,.T.);
#21101=ORIENTED_EDGE('',*,*,#14740,.F.);
#21102=ORIENTED_EDGE('',*,*,#14739,.F.);
#21103=ORIENTED_EDGE('',*,*,#14741,.T.);
#21104=ORIENTED_EDGE('',*,*,#14742,.F.);
#21105=ORIENTED_EDGE('',*,*,#14743,.F.);
#21106=ORIENTED_EDGE('',*,*,#14744,.F.);
#21107=ORIENTED_EDGE('',*,*,#14741,.F.);
#21108=ORIENTED_EDGE('',*,*,#14738,.F.);
#21109=ORIENTED_EDGE('',*,*,#14745,.F.);
#21110=ORIENTED_EDGE('',*,*,#14746,.T.);
#21111=ORIENTED_EDGE('',*,*,#14747,.T.);
#21112=ORIENTED_EDGE('',*,*,#14748,.F.);
#21113=ORIENTED_EDGE('',*,*,#14747,.F.);
#21114=ORIENTED_EDGE('',*,*,#14749,.T.);
#21115=ORIENTED_EDGE('',*,*,#14750,.F.);
#21116=ORIENTED_EDGE('',*,*,#14751,.F.);
#21117=ORIENTED_EDGE('',*,*,#14752,.F.);
#21118=ORIENTED_EDGE('',*,*,#14749,.F.);
#21119=ORIENTED_EDGE('',*,*,#14746,.F.);
#21120=ORIENTED_EDGE('',*,*,#14753,.F.);
#21121=ORIENTED_EDGE('',*,*,#14754,.T.);
#21122=ORIENTED_EDGE('',*,*,#14755,.T.);
#21123=ORIENTED_EDGE('',*,*,#14756,.F.);
#21124=ORIENTED_EDGE('',*,*,#14755,.F.);
#21125=ORIENTED_EDGE('',*,*,#14757,.T.);
#21126=ORIENTED_EDGE('',*,*,#14758,.F.);
#21127=ORIENTED_EDGE('',*,*,#14759,.F.);
#21128=ORIENTED_EDGE('',*,*,#14760,.F.);
#21129=ORIENTED_EDGE('',*,*,#14757,.F.);
#21130=ORIENTED_EDGE('',*,*,#14754,.F.);
#21131=ORIENTED_EDGE('',*,*,#14761,.F.);
#21132=ORIENTED_EDGE('',*,*,#14762,.T.);
#21133=ORIENTED_EDGE('',*,*,#14763,.T.);
#21134=ORIENTED_EDGE('',*,*,#14764,.F.);
#21135=ORIENTED_EDGE('',*,*,#14763,.F.);
#21136=ORIENTED_EDGE('',*,*,#14765,.T.);
#21137=ORIENTED_EDGE('',*,*,#14766,.F.);
#21138=ORIENTED_EDGE('',*,*,#14767,.F.);
#21139=ORIENTED_EDGE('',*,*,#14768,.F.);
#21140=ORIENTED_EDGE('',*,*,#14765,.F.);
#21141=ORIENTED_EDGE('',*,*,#14762,.F.);
#21142=ORIENTED_EDGE('',*,*,#14769,.F.);
#21143=ORIENTED_EDGE('',*,*,#14770,.T.);
#21144=ORIENTED_EDGE('',*,*,#14771,.T.);
#21145=ORIENTED_EDGE('',*,*,#14772,.F.);
#21146=ORIENTED_EDGE('',*,*,#14771,.F.);
#21147=ORIENTED_EDGE('',*,*,#14773,.T.);
#21148=ORIENTED_EDGE('',*,*,#14774,.F.);
#21149=ORIENTED_EDGE('',*,*,#14775,.F.);
#21150=ORIENTED_EDGE('',*,*,#14776,.F.);
#21151=ORIENTED_EDGE('',*,*,#14773,.F.);
#21152=ORIENTED_EDGE('',*,*,#14770,.F.);
#21153=ORIENTED_EDGE('',*,*,#14777,.F.);
#21154=ORIENTED_EDGE('',*,*,#14778,.T.);
#21155=ORIENTED_EDGE('',*,*,#14779,.T.);
#21156=ORIENTED_EDGE('',*,*,#14780,.F.);
#21157=ORIENTED_EDGE('',*,*,#14779,.F.);
#21158=ORIENTED_EDGE('',*,*,#14781,.T.);
#21159=ORIENTED_EDGE('',*,*,#14782,.F.);
#21160=ORIENTED_EDGE('',*,*,#14783,.F.);
#21161=ORIENTED_EDGE('',*,*,#14784,.F.);
#21162=ORIENTED_EDGE('',*,*,#14781,.F.);
#21163=ORIENTED_EDGE('',*,*,#14778,.F.);
#21164=ORIENTED_EDGE('',*,*,#14785,.F.);
#21165=ORIENTED_EDGE('',*,*,#14786,.T.);
#21166=ORIENTED_EDGE('',*,*,#14787,.T.);
#21167=ORIENTED_EDGE('',*,*,#14788,.F.);
#21168=ORIENTED_EDGE('',*,*,#14787,.F.);
#21169=ORIENTED_EDGE('',*,*,#14789,.T.);
#21170=ORIENTED_EDGE('',*,*,#14790,.F.);
#21171=ORIENTED_EDGE('',*,*,#14791,.F.);
#21172=ORIENTED_EDGE('',*,*,#14792,.F.);
#21173=ORIENTED_EDGE('',*,*,#14789,.F.);
#21174=ORIENTED_EDGE('',*,*,#14786,.F.);
#21175=ORIENTED_EDGE('',*,*,#14793,.F.);
#21176=ORIENTED_EDGE('',*,*,#14794,.T.);
#21177=ORIENTED_EDGE('',*,*,#14795,.T.);
#21178=ORIENTED_EDGE('',*,*,#14796,.F.);
#21179=ORIENTED_EDGE('',*,*,#14795,.F.);
#21180=ORIENTED_EDGE('',*,*,#14797,.T.);
#21181=ORIENTED_EDGE('',*,*,#14798,.F.);
#21182=ORIENTED_EDGE('',*,*,#14799,.F.);
#21183=ORIENTED_EDGE('',*,*,#14800,.F.);
#21184=ORIENTED_EDGE('',*,*,#14797,.F.);
#21185=ORIENTED_EDGE('',*,*,#14794,.F.);
#21186=ORIENTED_EDGE('',*,*,#14801,.F.);
#21187=ORIENTED_EDGE('',*,*,#14802,.T.);
#21188=ORIENTED_EDGE('',*,*,#14803,.T.);
#21189=ORIENTED_EDGE('',*,*,#14804,.F.);
#21190=ORIENTED_EDGE('',*,*,#14803,.F.);
#21191=ORIENTED_EDGE('',*,*,#14805,.T.);
#21192=ORIENTED_EDGE('',*,*,#14806,.F.);
#21193=ORIENTED_EDGE('',*,*,#14807,.F.);
#21194=ORIENTED_EDGE('',*,*,#14808,.F.);
#21195=ORIENTED_EDGE('',*,*,#14805,.F.);
#21196=ORIENTED_EDGE('',*,*,#14802,.F.);
#21197=ORIENTED_EDGE('',*,*,#14809,.F.);
#21198=ORIENTED_EDGE('',*,*,#14810,.T.);
#21199=ORIENTED_EDGE('',*,*,#14811,.T.);
#21200=ORIENTED_EDGE('',*,*,#14812,.F.);
#21201=ORIENTED_EDGE('',*,*,#14811,.F.);
#21202=ORIENTED_EDGE('',*,*,#14813,.T.);
#21203=ORIENTED_EDGE('',*,*,#14814,.F.);
#21204=ORIENTED_EDGE('',*,*,#14815,.F.);
#21205=ORIENTED_EDGE('',*,*,#14816,.F.);
#21206=ORIENTED_EDGE('',*,*,#14813,.F.);
#21207=ORIENTED_EDGE('',*,*,#14810,.F.);
#21208=ORIENTED_EDGE('',*,*,#14817,.F.);
#21209=ORIENTED_EDGE('',*,*,#14818,.T.);
#21210=ORIENTED_EDGE('',*,*,#14819,.T.);
#21211=ORIENTED_EDGE('',*,*,#14820,.F.);
#21212=ORIENTED_EDGE('',*,*,#14819,.F.);
#21213=ORIENTED_EDGE('',*,*,#14821,.T.);
#21214=ORIENTED_EDGE('',*,*,#14822,.F.);
#21215=ORIENTED_EDGE('',*,*,#14823,.F.);
#21216=ORIENTED_EDGE('',*,*,#14824,.F.);
#21217=ORIENTED_EDGE('',*,*,#14821,.F.);
#21218=ORIENTED_EDGE('',*,*,#14818,.F.);
#21219=ORIENTED_EDGE('',*,*,#14825,.F.);
#21220=ORIENTED_EDGE('',*,*,#14826,.T.);
#21221=ORIENTED_EDGE('',*,*,#14827,.T.);
#21222=ORIENTED_EDGE('',*,*,#14828,.F.);
#21223=ORIENTED_EDGE('',*,*,#14827,.F.);
#21224=ORIENTED_EDGE('',*,*,#14829,.T.);
#21225=ORIENTED_EDGE('',*,*,#14830,.F.);
#21226=ORIENTED_EDGE('',*,*,#14831,.F.);
#21227=ORIENTED_EDGE('',*,*,#14832,.F.);
#21228=ORIENTED_EDGE('',*,*,#14829,.F.);
#21229=ORIENTED_EDGE('',*,*,#14826,.F.);
#21230=ORIENTED_EDGE('',*,*,#14833,.F.);
#21231=ORIENTED_EDGE('',*,*,#14834,.T.);
#21232=ORIENTED_EDGE('',*,*,#14835,.T.);
#21233=ORIENTED_EDGE('',*,*,#14836,.F.);
#21234=ORIENTED_EDGE('',*,*,#14835,.F.);
#21235=ORIENTED_EDGE('',*,*,#14837,.T.);
#21236=ORIENTED_EDGE('',*,*,#14838,.F.);
#21237=ORIENTED_EDGE('',*,*,#14839,.F.);
#21238=ORIENTED_EDGE('',*,*,#14840,.F.);
#21239=ORIENTED_EDGE('',*,*,#14837,.F.);
#21240=ORIENTED_EDGE('',*,*,#14834,.F.);
#21241=ORIENTED_EDGE('',*,*,#14841,.F.);
#21242=ORIENTED_EDGE('',*,*,#14842,.T.);
#21243=ORIENTED_EDGE('',*,*,#14843,.T.);
#21244=ORIENTED_EDGE('',*,*,#14844,.F.);
#21245=ORIENTED_EDGE('',*,*,#14843,.F.);
#21246=ORIENTED_EDGE('',*,*,#14845,.T.);
#21247=ORIENTED_EDGE('',*,*,#14846,.F.);
#21248=ORIENTED_EDGE('',*,*,#14847,.F.);
#21249=ORIENTED_EDGE('',*,*,#14848,.F.);
#21250=ORIENTED_EDGE('',*,*,#14845,.F.);
#21251=ORIENTED_EDGE('',*,*,#14842,.F.);
#21252=ORIENTED_EDGE('',*,*,#14849,.F.);
#21253=ORIENTED_EDGE('',*,*,#14850,.T.);
#21254=ORIENTED_EDGE('',*,*,#14851,.T.);
#21255=ORIENTED_EDGE('',*,*,#14852,.F.);
#21256=ORIENTED_EDGE('',*,*,#14853,.F.);
#21257=ORIENTED_EDGE('',*,*,#14851,.F.);
#21258=ORIENTED_EDGE('',*,*,#14854,.T.);
#21259=ORIENTED_EDGE('',*,*,#14855,.F.);
#21260=ORIENTED_EDGE('',*,*,#14856,.F.);
#21261=ORIENTED_EDGE('',*,*,#14857,.F.);
#21262=ORIENTED_EDGE('',*,*,#14854,.F.);
#21263=ORIENTED_EDGE('',*,*,#14850,.F.);
#21264=ORIENTED_EDGE('',*,*,#14858,.F.);
#21265=ORIENTED_EDGE('',*,*,#14859,.T.);
#21266=ORIENTED_EDGE('',*,*,#14860,.T.);
#21267=ORIENTED_EDGE('',*,*,#14861,.F.);
#21268=ORIENTED_EDGE('',*,*,#14860,.F.);
#21269=ORIENTED_EDGE('',*,*,#14862,.T.);
#21270=ORIENTED_EDGE('',*,*,#14863,.F.);
#21271=ORIENTED_EDGE('',*,*,#14864,.F.);
#21272=ORIENTED_EDGE('',*,*,#14865,.F.);
#21273=ORIENTED_EDGE('',*,*,#14862,.F.);
#21274=ORIENTED_EDGE('',*,*,#14859,.F.);
#21275=ORIENTED_EDGE('',*,*,#14866,.F.);
#21276=ORIENTED_EDGE('',*,*,#14867,.T.);
#21277=ORIENTED_EDGE('',*,*,#14868,.T.);
#21278=ORIENTED_EDGE('',*,*,#14869,.F.);
#21279=ORIENTED_EDGE('',*,*,#14868,.F.);
#21280=ORIENTED_EDGE('',*,*,#14870,.T.);
#21281=ORIENTED_EDGE('',*,*,#14871,.F.);
#21282=ORIENTED_EDGE('',*,*,#14872,.F.);
#21283=ORIENTED_EDGE('',*,*,#14873,.F.);
#21284=ORIENTED_EDGE('',*,*,#14870,.F.);
#21285=ORIENTED_EDGE('',*,*,#14867,.F.);
#21286=ORIENTED_EDGE('',*,*,#14874,.F.);
#21287=ORIENTED_EDGE('',*,*,#14875,.T.);
#21288=ORIENTED_EDGE('',*,*,#14876,.T.);
#21289=ORIENTED_EDGE('',*,*,#14877,.F.);
#21290=ORIENTED_EDGE('',*,*,#14876,.F.);
#21291=ORIENTED_EDGE('',*,*,#14878,.T.);
#21292=ORIENTED_EDGE('',*,*,#14879,.F.);
#21293=ORIENTED_EDGE('',*,*,#14880,.F.);
#21294=ORIENTED_EDGE('',*,*,#14881,.F.);
#21295=ORIENTED_EDGE('',*,*,#14878,.F.);
#21296=ORIENTED_EDGE('',*,*,#14875,.F.);
#21297=ORIENTED_EDGE('',*,*,#14882,.F.);
#21298=ORIENTED_EDGE('',*,*,#14883,.T.);
#21299=ORIENTED_EDGE('',*,*,#14884,.T.);
#21300=ORIENTED_EDGE('',*,*,#14885,.F.);
#21301=ORIENTED_EDGE('',*,*,#14884,.F.);
#21302=ORIENTED_EDGE('',*,*,#14886,.T.);
#21303=ORIENTED_EDGE('',*,*,#14887,.F.);
#21304=ORIENTED_EDGE('',*,*,#14888,.F.);
#21305=ORIENTED_EDGE('',*,*,#14889,.F.);
#21306=ORIENTED_EDGE('',*,*,#14886,.F.);
#21307=ORIENTED_EDGE('',*,*,#14883,.F.);
#21308=ORIENTED_EDGE('',*,*,#14890,.F.);
#21309=ORIENTED_EDGE('',*,*,#14891,.T.);
#21310=ORIENTED_EDGE('',*,*,#14892,.T.);
#21311=ORIENTED_EDGE('',*,*,#14893,.F.);
#21312=ORIENTED_EDGE('',*,*,#14892,.F.);
#21313=ORIENTED_EDGE('',*,*,#14894,.T.);
#21314=ORIENTED_EDGE('',*,*,#14895,.F.);
#21315=ORIENTED_EDGE('',*,*,#14896,.F.);
#21316=ORIENTED_EDGE('',*,*,#14897,.F.);
#21317=ORIENTED_EDGE('',*,*,#14894,.F.);
#21318=ORIENTED_EDGE('',*,*,#14891,.F.);
#21319=ORIENTED_EDGE('',*,*,#14898,.F.);
#21320=ORIENTED_EDGE('',*,*,#14899,.T.);
#21321=ORIENTED_EDGE('',*,*,#14900,.T.);
#21322=ORIENTED_EDGE('',*,*,#14901,.F.);
#21323=ORIENTED_EDGE('',*,*,#14900,.F.);
#21324=ORIENTED_EDGE('',*,*,#14902,.T.);
#21325=ORIENTED_EDGE('',*,*,#14903,.F.);
#21326=ORIENTED_EDGE('',*,*,#14904,.F.);
#21327=ORIENTED_EDGE('',*,*,#14905,.F.);
#21328=ORIENTED_EDGE('',*,*,#14902,.F.);
#21329=ORIENTED_EDGE('',*,*,#14899,.F.);
#21330=ORIENTED_EDGE('',*,*,#14906,.F.);
#21331=ORIENTED_EDGE('',*,*,#14907,.T.);
#21332=ORIENTED_EDGE('',*,*,#14908,.T.);
#21333=ORIENTED_EDGE('',*,*,#14909,.F.);
#21334=ORIENTED_EDGE('',*,*,#14908,.F.);
#21335=ORIENTED_EDGE('',*,*,#14910,.T.);
#21336=ORIENTED_EDGE('',*,*,#14911,.F.);
#21337=ORIENTED_EDGE('',*,*,#14912,.F.);
#21338=ORIENTED_EDGE('',*,*,#14913,.F.);
#21339=ORIENTED_EDGE('',*,*,#14910,.F.);
#21340=ORIENTED_EDGE('',*,*,#14907,.F.);
#21341=ORIENTED_EDGE('',*,*,#14914,.F.);
#21342=ORIENTED_EDGE('',*,*,#14915,.T.);
#21343=ORIENTED_EDGE('',*,*,#14916,.T.);
#21344=ORIENTED_EDGE('',*,*,#14917,.F.);
#21345=ORIENTED_EDGE('',*,*,#14916,.F.);
#21346=ORIENTED_EDGE('',*,*,#14918,.T.);
#21347=ORIENTED_EDGE('',*,*,#14919,.F.);
#21348=ORIENTED_EDGE('',*,*,#14920,.F.);
#21349=ORIENTED_EDGE('',*,*,#14921,.F.);
#21350=ORIENTED_EDGE('',*,*,#14918,.F.);
#21351=ORIENTED_EDGE('',*,*,#14915,.F.);
#21352=ORIENTED_EDGE('',*,*,#14922,.F.);
#21353=ORIENTED_EDGE('',*,*,#14923,.T.);
#21354=ORIENTED_EDGE('',*,*,#14924,.T.);
#21355=ORIENTED_EDGE('',*,*,#14925,.F.);
#21356=ORIENTED_EDGE('',*,*,#14924,.F.);
#21357=ORIENTED_EDGE('',*,*,#14926,.T.);
#21358=ORIENTED_EDGE('',*,*,#14927,.F.);
#21359=ORIENTED_EDGE('',*,*,#14928,.F.);
#21360=ORIENTED_EDGE('',*,*,#14929,.F.);
#21361=ORIENTED_EDGE('',*,*,#14926,.F.);
#21362=ORIENTED_EDGE('',*,*,#14923,.F.);
#21363=ORIENTED_EDGE('',*,*,#14930,.F.);
#21364=ORIENTED_EDGE('',*,*,#14931,.T.);
#21365=ORIENTED_EDGE('',*,*,#14932,.T.);
#21366=ORIENTED_EDGE('',*,*,#14933,.F.);
#21367=ORIENTED_EDGE('',*,*,#14932,.F.);
#21368=ORIENTED_EDGE('',*,*,#14934,.T.);
#21369=ORIENTED_EDGE('',*,*,#14935,.F.);
#21370=ORIENTED_EDGE('',*,*,#14936,.F.);
#21371=ORIENTED_EDGE('',*,*,#14937,.F.);
#21372=ORIENTED_EDGE('',*,*,#14934,.F.);
#21373=ORIENTED_EDGE('',*,*,#14931,.F.);
#21374=ORIENTED_EDGE('',*,*,#14938,.F.);
#21375=ORIENTED_EDGE('',*,*,#14939,.T.);
#21376=ORIENTED_EDGE('',*,*,#14940,.T.);
#21377=ORIENTED_EDGE('',*,*,#14941,.F.);
#21378=ORIENTED_EDGE('',*,*,#14940,.F.);
#21379=ORIENTED_EDGE('',*,*,#14942,.T.);
#21380=ORIENTED_EDGE('',*,*,#14943,.F.);
#21381=ORIENTED_EDGE('',*,*,#14944,.F.);
#21382=ORIENTED_EDGE('',*,*,#14945,.F.);
#21383=ORIENTED_EDGE('',*,*,#14942,.F.);
#21384=ORIENTED_EDGE('',*,*,#14939,.F.);
#21385=ORIENTED_EDGE('',*,*,#14946,.F.);
#21386=ORIENTED_EDGE('',*,*,#14947,.T.);
#21387=ORIENTED_EDGE('',*,*,#14948,.T.);
#21388=ORIENTED_EDGE('',*,*,#14949,.F.);
#21389=ORIENTED_EDGE('',*,*,#14948,.F.);
#21390=ORIENTED_EDGE('',*,*,#14950,.T.);
#21391=ORIENTED_EDGE('',*,*,#14951,.F.);
#21392=ORIENTED_EDGE('',*,*,#14952,.F.);
#21393=ORIENTED_EDGE('',*,*,#14953,.F.);
#21394=ORIENTED_EDGE('',*,*,#14950,.F.);
#21395=ORIENTED_EDGE('',*,*,#14947,.F.);
#21396=ORIENTED_EDGE('',*,*,#14954,.F.);
#21397=ORIENTED_EDGE('',*,*,#14955,.T.);
#21398=ORIENTED_EDGE('',*,*,#14956,.T.);
#21399=ORIENTED_EDGE('',*,*,#14957,.F.);
#21400=ORIENTED_EDGE('',*,*,#14956,.F.);
#21401=ORIENTED_EDGE('',*,*,#14958,.T.);
#21402=ORIENTED_EDGE('',*,*,#14959,.F.);
#21403=ORIENTED_EDGE('',*,*,#14960,.F.);
#21404=ORIENTED_EDGE('',*,*,#14961,.F.);
#21405=ORIENTED_EDGE('',*,*,#14958,.F.);
#21406=ORIENTED_EDGE('',*,*,#14955,.F.);
#21407=ORIENTED_EDGE('',*,*,#14962,.F.);
#21408=ORIENTED_EDGE('',*,*,#14963,.T.);
#21409=ORIENTED_EDGE('',*,*,#14964,.T.);
#21410=ORIENTED_EDGE('',*,*,#14965,.F.);
#21411=ORIENTED_EDGE('',*,*,#14964,.F.);
#21412=ORIENTED_EDGE('',*,*,#14966,.T.);
#21413=ORIENTED_EDGE('',*,*,#14967,.F.);
#21414=ORIENTED_EDGE('',*,*,#14968,.F.);
#21415=ORIENTED_EDGE('',*,*,#14969,.F.);
#21416=ORIENTED_EDGE('',*,*,#14966,.F.);
#21417=ORIENTED_EDGE('',*,*,#14963,.F.);
#21418=ORIENTED_EDGE('',*,*,#14970,.F.);
#21419=ORIENTED_EDGE('',*,*,#14971,.T.);
#21420=ORIENTED_EDGE('',*,*,#14972,.T.);
#21421=ORIENTED_EDGE('',*,*,#14973,.F.);
#21422=ORIENTED_EDGE('',*,*,#14972,.F.);
#21423=ORIENTED_EDGE('',*,*,#14974,.T.);
#21424=ORIENTED_EDGE('',*,*,#14975,.F.);
#21425=ORIENTED_EDGE('',*,*,#14976,.F.);
#21426=ORIENTED_EDGE('',*,*,#14977,.F.);
#21427=ORIENTED_EDGE('',*,*,#14974,.F.);
#21428=ORIENTED_EDGE('',*,*,#14971,.F.);
#21429=ORIENTED_EDGE('',*,*,#14978,.F.);
#21430=ORIENTED_EDGE('',*,*,#14979,.T.);
#21431=ORIENTED_EDGE('',*,*,#14980,.T.);
#21432=ORIENTED_EDGE('',*,*,#14981,.F.);
#21433=ORIENTED_EDGE('',*,*,#14980,.F.);
#21434=ORIENTED_EDGE('',*,*,#14982,.T.);
#21435=ORIENTED_EDGE('',*,*,#14983,.F.);
#21436=ORIENTED_EDGE('',*,*,#14984,.F.);
#21437=ORIENTED_EDGE('',*,*,#14985,.F.);
#21438=ORIENTED_EDGE('',*,*,#14982,.F.);
#21439=ORIENTED_EDGE('',*,*,#14979,.F.);
#21440=ORIENTED_EDGE('',*,*,#14986,.F.);
#21441=ORIENTED_EDGE('',*,*,#14987,.T.);
#21442=ORIENTED_EDGE('',*,*,#14988,.T.);
#21443=ORIENTED_EDGE('',*,*,#14989,.F.);
#21444=ORIENTED_EDGE('',*,*,#14988,.F.);
#21445=ORIENTED_EDGE('',*,*,#14990,.T.);
#21446=ORIENTED_EDGE('',*,*,#14991,.F.);
#21447=ORIENTED_EDGE('',*,*,#14992,.F.);
#21448=ORIENTED_EDGE('',*,*,#14993,.F.);
#21449=ORIENTED_EDGE('',*,*,#14990,.F.);
#21450=ORIENTED_EDGE('',*,*,#14987,.F.);
#21451=ORIENTED_EDGE('',*,*,#14719,.T.);
#21452=ORIENTED_EDGE('',*,*,#14713,.T.);
#21453=ORIENTED_EDGE('',*,*,#14716,.T.);
#21454=ORIENTED_EDGE('',*,*,#14994,.F.);
#21455=ORIENTED_EDGE('',*,*,#14727,.T.);
#21456=ORIENTED_EDGE('',*,*,#14721,.T.);
#21457=ORIENTED_EDGE('',*,*,#14724,.T.);
#21458=ORIENTED_EDGE('',*,*,#14995,.F.);
#21459=ORIENTED_EDGE('',*,*,#14735,.T.);
#21460=ORIENTED_EDGE('',*,*,#14729,.T.);
#21461=ORIENTED_EDGE('',*,*,#14732,.T.);
#21462=ORIENTED_EDGE('',*,*,#14996,.F.);
#21463=ORIENTED_EDGE('',*,*,#14743,.T.);
#21464=ORIENTED_EDGE('',*,*,#14737,.T.);
#21465=ORIENTED_EDGE('',*,*,#14740,.T.);
#21466=ORIENTED_EDGE('',*,*,#14997,.F.);
#21467=ORIENTED_EDGE('',*,*,#14751,.T.);
#21468=ORIENTED_EDGE('',*,*,#14745,.T.);
#21469=ORIENTED_EDGE('',*,*,#14748,.T.);
#21470=ORIENTED_EDGE('',*,*,#14998,.F.);
#21471=ORIENTED_EDGE('',*,*,#14759,.T.);
#21472=ORIENTED_EDGE('',*,*,#14753,.T.);
#21473=ORIENTED_EDGE('',*,*,#14756,.T.);
#21474=ORIENTED_EDGE('',*,*,#14999,.F.);
#21475=ORIENTED_EDGE('',*,*,#14767,.T.);
#21476=ORIENTED_EDGE('',*,*,#14761,.T.);
#21477=ORIENTED_EDGE('',*,*,#14764,.T.);
#21478=ORIENTED_EDGE('',*,*,#15000,.F.);
#21479=ORIENTED_EDGE('',*,*,#14775,.T.);
#21480=ORIENTED_EDGE('',*,*,#14769,.T.);
#21481=ORIENTED_EDGE('',*,*,#14772,.T.);
#21482=ORIENTED_EDGE('',*,*,#15001,.F.);
#21483=ORIENTED_EDGE('',*,*,#14783,.T.);
#21484=ORIENTED_EDGE('',*,*,#14777,.T.);
#21485=ORIENTED_EDGE('',*,*,#14780,.T.);
#21486=ORIENTED_EDGE('',*,*,#15002,.F.);
#21487=ORIENTED_EDGE('',*,*,#14791,.T.);
#21488=ORIENTED_EDGE('',*,*,#14785,.T.);
#21489=ORIENTED_EDGE('',*,*,#14788,.T.);
#21490=ORIENTED_EDGE('',*,*,#15003,.F.);
#21491=ORIENTED_EDGE('',*,*,#14799,.T.);
#21492=ORIENTED_EDGE('',*,*,#14793,.T.);
#21493=ORIENTED_EDGE('',*,*,#14796,.T.);
#21494=ORIENTED_EDGE('',*,*,#15004,.F.);
#21495=ORIENTED_EDGE('',*,*,#14807,.T.);
#21496=ORIENTED_EDGE('',*,*,#14801,.T.);
#21497=ORIENTED_EDGE('',*,*,#14804,.T.);
#21498=ORIENTED_EDGE('',*,*,#15005,.F.);
#21499=ORIENTED_EDGE('',*,*,#14815,.T.);
#21500=ORIENTED_EDGE('',*,*,#14809,.T.);
#21501=ORIENTED_EDGE('',*,*,#14812,.T.);
#21502=ORIENTED_EDGE('',*,*,#15006,.F.);
#21503=ORIENTED_EDGE('',*,*,#14823,.T.);
#21504=ORIENTED_EDGE('',*,*,#14817,.T.);
#21505=ORIENTED_EDGE('',*,*,#14820,.T.);
#21506=ORIENTED_EDGE('',*,*,#15007,.F.);
#21507=ORIENTED_EDGE('',*,*,#14831,.T.);
#21508=ORIENTED_EDGE('',*,*,#14825,.T.);
#21509=ORIENTED_EDGE('',*,*,#14828,.T.);
#21510=ORIENTED_EDGE('',*,*,#15008,.F.);
#21511=ORIENTED_EDGE('',*,*,#14839,.T.);
#21512=ORIENTED_EDGE('',*,*,#14833,.T.);
#21513=ORIENTED_EDGE('',*,*,#14836,.T.);
#21514=ORIENTED_EDGE('',*,*,#15009,.F.);
#21515=ORIENTED_EDGE('',*,*,#14847,.T.);
#21516=ORIENTED_EDGE('',*,*,#14841,.T.);
#21517=ORIENTED_EDGE('',*,*,#14844,.T.);
#21518=ORIENTED_EDGE('',*,*,#15010,.F.);
#21519=ORIENTED_EDGE('',*,*,#14856,.T.);
#21520=ORIENTED_EDGE('',*,*,#14849,.T.);
#21521=ORIENTED_EDGE('',*,*,#15011,.T.);
#21522=ORIENTED_EDGE('',*,*,#15012,.T.);
#21523=ORIENTED_EDGE('',*,*,#15011,.F.);
#21524=ORIENTED_EDGE('',*,*,#14852,.T.);
#21525=ORIENTED_EDGE('',*,*,#14853,.T.);
#21526=ORIENTED_EDGE('',*,*,#15013,.F.);
#21527=ORIENTED_EDGE('',*,*,#14864,.T.);
#21528=ORIENTED_EDGE('',*,*,#14858,.T.);
#21529=ORIENTED_EDGE('',*,*,#14861,.T.);
#21530=ORIENTED_EDGE('',*,*,#15014,.F.);
#21531=ORIENTED_EDGE('',*,*,#14872,.T.);
#21532=ORIENTED_EDGE('',*,*,#14866,.T.);
#21533=ORIENTED_EDGE('',*,*,#14869,.T.);
#21534=ORIENTED_EDGE('',*,*,#15015,.F.);
#21535=ORIENTED_EDGE('',*,*,#14880,.T.);
#21536=ORIENTED_EDGE('',*,*,#14874,.T.);
#21537=ORIENTED_EDGE('',*,*,#14877,.T.);
#21538=ORIENTED_EDGE('',*,*,#15016,.F.);
#21539=ORIENTED_EDGE('',*,*,#14888,.T.);
#21540=ORIENTED_EDGE('',*,*,#14882,.T.);
#21541=ORIENTED_EDGE('',*,*,#14885,.T.);
#21542=ORIENTED_EDGE('',*,*,#15017,.F.);
#21543=ORIENTED_EDGE('',*,*,#14896,.T.);
#21544=ORIENTED_EDGE('',*,*,#14890,.T.);
#21545=ORIENTED_EDGE('',*,*,#14893,.T.);
#21546=ORIENTED_EDGE('',*,*,#15018,.F.);
#21547=ORIENTED_EDGE('',*,*,#14904,.T.);
#21548=ORIENTED_EDGE('',*,*,#14898,.T.);
#21549=ORIENTED_EDGE('',*,*,#14901,.T.);
#21550=ORIENTED_EDGE('',*,*,#15019,.F.);
#21551=ORIENTED_EDGE('',*,*,#14912,.T.);
#21552=ORIENTED_EDGE('',*,*,#14906,.T.);
#21553=ORIENTED_EDGE('',*,*,#14909,.T.);
#21554=ORIENTED_EDGE('',*,*,#15020,.F.);
#21555=ORIENTED_EDGE('',*,*,#14920,.T.);
#21556=ORIENTED_EDGE('',*,*,#14914,.T.);
#21557=ORIENTED_EDGE('',*,*,#14917,.T.);
#21558=ORIENTED_EDGE('',*,*,#15021,.F.);
#21559=ORIENTED_EDGE('',*,*,#14928,.T.);
#21560=ORIENTED_EDGE('',*,*,#14922,.T.);
#21561=ORIENTED_EDGE('',*,*,#14925,.T.);
#21562=ORIENTED_EDGE('',*,*,#15022,.F.);
#21563=ORIENTED_EDGE('',*,*,#14936,.T.);
#21564=ORIENTED_EDGE('',*,*,#14930,.T.);
#21565=ORIENTED_EDGE('',*,*,#14933,.T.);
#21566=ORIENTED_EDGE('',*,*,#15023,.F.);
#21567=ORIENTED_EDGE('',*,*,#14944,.T.);
#21568=ORIENTED_EDGE('',*,*,#14938,.T.);
#21569=ORIENTED_EDGE('',*,*,#14941,.T.);
#21570=ORIENTED_EDGE('',*,*,#15024,.F.);
#21571=ORIENTED_EDGE('',*,*,#14952,.T.);
#21572=ORIENTED_EDGE('',*,*,#14946,.T.);
#21573=ORIENTED_EDGE('',*,*,#14949,.T.);
#21574=ORIENTED_EDGE('',*,*,#15025,.F.);
#21575=ORIENTED_EDGE('',*,*,#14960,.T.);
#21576=ORIENTED_EDGE('',*,*,#14954,.T.);
#21577=ORIENTED_EDGE('',*,*,#14957,.T.);
#21578=ORIENTED_EDGE('',*,*,#15026,.F.);
#21579=ORIENTED_EDGE('',*,*,#14968,.T.);
#21580=ORIENTED_EDGE('',*,*,#14962,.T.);
#21581=ORIENTED_EDGE('',*,*,#14965,.T.);
#21582=ORIENTED_EDGE('',*,*,#15027,.F.);
#21583=ORIENTED_EDGE('',*,*,#14976,.T.);
#21584=ORIENTED_EDGE('',*,*,#14970,.T.);
#21585=ORIENTED_EDGE('',*,*,#14973,.T.);
#21586=ORIENTED_EDGE('',*,*,#15028,.F.);
#21587=ORIENTED_EDGE('',*,*,#14984,.T.);
#21588=ORIENTED_EDGE('',*,*,#14978,.T.);
#21589=ORIENTED_EDGE('',*,*,#14981,.T.);
#21590=ORIENTED_EDGE('',*,*,#15029,.F.);
#21591=ORIENTED_EDGE('',*,*,#14992,.T.);
#21592=ORIENTED_EDGE('',*,*,#14986,.T.);
#21593=ORIENTED_EDGE('',*,*,#14989,.T.);
#21594=ORIENTED_EDGE('',*,*,#15030,.F.);
#21595=ORIENTED_EDGE('',*,*,#15031,.T.);
#21596=ORIENTED_EDGE('',*,*,#15032,.T.);
#21597=ORIENTED_EDGE('',*,*,#15033,.T.);
#21598=ORIENTED_EDGE('',*,*,#15034,.F.);
#21599=ORIENTED_EDGE('',*,*,#15033,.F.);
#21600=ORIENTED_EDGE('',*,*,#15035,.F.);
#21601=ORIENTED_EDGE('',*,*,#15036,.T.);
#21602=ORIENTED_EDGE('',*,*,#15037,.F.);
#21603=ORIENTED_EDGE('',*,*,#15038,.F.);
#21604=ORIENTED_EDGE('',*,*,#15036,.F.);
#21605=ORIENTED_EDGE('',*,*,#15039,.F.);
#21606=ORIENTED_EDGE('',*,*,#15031,.F.);
#21607=ORIENTED_EDGE('',*,*,#15032,.F.);
#21608=ORIENTED_EDGE('',*,*,#15039,.T.);
#21609=ORIENTED_EDGE('',*,*,#15035,.T.);
#21610=ORIENTED_EDGE('',*,*,#15040,.F.);
#21611=ORIENTED_EDGE('',*,*,#15041,.T.);
#21612=ORIENTED_EDGE('',*,*,#14857,.T.);
#21613=ORIENTED_EDGE('',*,*,#15010,.T.);
#21614=ORIENTED_EDGE('',*,*,#14846,.T.);
#21615=ORIENTED_EDGE('',*,*,#14848,.T.);
#21616=ORIENTED_EDGE('',*,*,#15009,.T.);
#21617=ORIENTED_EDGE('',*,*,#14838,.T.);
#21618=ORIENTED_EDGE('',*,*,#14840,.T.);
#21619=ORIENTED_EDGE('',*,*,#15008,.T.);
#21620=ORIENTED_EDGE('',*,*,#14830,.T.);
#21621=ORIENTED_EDGE('',*,*,#14832,.T.);
#21622=ORIENTED_EDGE('',*,*,#15007,.T.);
#21623=ORIENTED_EDGE('',*,*,#14822,.T.);
#21624=ORIENTED_EDGE('',*,*,#14824,.T.);
#21625=ORIENTED_EDGE('',*,*,#15006,.T.);
#21626=ORIENTED_EDGE('',*,*,#14814,.T.);
#21627=ORIENTED_EDGE('',*,*,#14816,.T.);
#21628=ORIENTED_EDGE('',*,*,#15005,.T.);
#21629=ORIENTED_EDGE('',*,*,#14806,.T.);
#21630=ORIENTED_EDGE('',*,*,#14808,.T.);
#21631=ORIENTED_EDGE('',*,*,#15004,.T.);
#21632=ORIENTED_EDGE('',*,*,#14798,.T.);
#21633=ORIENTED_EDGE('',*,*,#14800,.T.);
#21634=ORIENTED_EDGE('',*,*,#15003,.T.);
#21635=ORIENTED_EDGE('',*,*,#14790,.T.);
#21636=ORIENTED_EDGE('',*,*,#14792,.T.);
#21637=ORIENTED_EDGE('',*,*,#15002,.T.);
#21638=ORIENTED_EDGE('',*,*,#14782,.T.);
#21639=ORIENTED_EDGE('',*,*,#14784,.T.);
#21640=ORIENTED_EDGE('',*,*,#15001,.T.);
#21641=ORIENTED_EDGE('',*,*,#14774,.T.);
#21642=ORIENTED_EDGE('',*,*,#14776,.T.);
#21643=ORIENTED_EDGE('',*,*,#15000,.T.);
#21644=ORIENTED_EDGE('',*,*,#14766,.T.);
#21645=ORIENTED_EDGE('',*,*,#14768,.T.);
#21646=ORIENTED_EDGE('',*,*,#14999,.T.);
#21647=ORIENTED_EDGE('',*,*,#14758,.T.);
#21648=ORIENTED_EDGE('',*,*,#14760,.T.);
#21649=ORIENTED_EDGE('',*,*,#14998,.T.);
#21650=ORIENTED_EDGE('',*,*,#14750,.T.);
#21651=ORIENTED_EDGE('',*,*,#14752,.T.);
#21652=ORIENTED_EDGE('',*,*,#14997,.T.);
#21653=ORIENTED_EDGE('',*,*,#14742,.T.);
#21654=ORIENTED_EDGE('',*,*,#14744,.T.);
#21655=ORIENTED_EDGE('',*,*,#14996,.T.);
#21656=ORIENTED_EDGE('',*,*,#14734,.T.);
#21657=ORIENTED_EDGE('',*,*,#14736,.T.);
#21658=ORIENTED_EDGE('',*,*,#14995,.T.);
#21659=ORIENTED_EDGE('',*,*,#14726,.T.);
#21660=ORIENTED_EDGE('',*,*,#14728,.T.);
#21661=ORIENTED_EDGE('',*,*,#14994,.T.);
#21662=ORIENTED_EDGE('',*,*,#14718,.T.);
#21663=ORIENTED_EDGE('',*,*,#14720,.T.);
#21664=ORIENTED_EDGE('',*,*,#15034,.T.);
#21665=ORIENTED_EDGE('',*,*,#15037,.T.);
#21666=ORIENTED_EDGE('',*,*,#15038,.T.);
#21667=ORIENTED_EDGE('',*,*,#15030,.T.);
#21668=ORIENTED_EDGE('',*,*,#14991,.T.);
#21669=ORIENTED_EDGE('',*,*,#14993,.T.);
#21670=ORIENTED_EDGE('',*,*,#15029,.T.);
#21671=ORIENTED_EDGE('',*,*,#14983,.T.);
#21672=ORIENTED_EDGE('',*,*,#14985,.T.);
#21673=ORIENTED_EDGE('',*,*,#15028,.T.);
#21674=ORIENTED_EDGE('',*,*,#14975,.T.);
#21675=ORIENTED_EDGE('',*,*,#14977,.T.);
#21676=ORIENTED_EDGE('',*,*,#15027,.T.);
#21677=ORIENTED_EDGE('',*,*,#14967,.T.);
#21678=ORIENTED_EDGE('',*,*,#14969,.T.);
#21679=ORIENTED_EDGE('',*,*,#15026,.T.);
#21680=ORIENTED_EDGE('',*,*,#14959,.T.);
#21681=ORIENTED_EDGE('',*,*,#14961,.T.);
#21682=ORIENTED_EDGE('',*,*,#15025,.T.);
#21683=ORIENTED_EDGE('',*,*,#14951,.T.);
#21684=ORIENTED_EDGE('',*,*,#14953,.T.);
#21685=ORIENTED_EDGE('',*,*,#15024,.T.);
#21686=ORIENTED_EDGE('',*,*,#14943,.T.);
#21687=ORIENTED_EDGE('',*,*,#14945,.T.);
#21688=ORIENTED_EDGE('',*,*,#15023,.T.);
#21689=ORIENTED_EDGE('',*,*,#14935,.T.);
#21690=ORIENTED_EDGE('',*,*,#14937,.T.);
#21691=ORIENTED_EDGE('',*,*,#15022,.T.);
#21692=ORIENTED_EDGE('',*,*,#14927,.T.);
#21693=ORIENTED_EDGE('',*,*,#14929,.T.);
#21694=ORIENTED_EDGE('',*,*,#15021,.T.);
#21695=ORIENTED_EDGE('',*,*,#14919,.T.);
#21696=ORIENTED_EDGE('',*,*,#14921,.T.);
#21697=ORIENTED_EDGE('',*,*,#15020,.T.);
#21698=ORIENTED_EDGE('',*,*,#14911,.T.);
#21699=ORIENTED_EDGE('',*,*,#14913,.T.);
#21700=ORIENTED_EDGE('',*,*,#15019,.T.);
#21701=ORIENTED_EDGE('',*,*,#14903,.T.);
#21702=ORIENTED_EDGE('',*,*,#14905,.T.);
#21703=ORIENTED_EDGE('',*,*,#15018,.T.);
#21704=ORIENTED_EDGE('',*,*,#14895,.T.);
#21705=ORIENTED_EDGE('',*,*,#14897,.T.);
#21706=ORIENTED_EDGE('',*,*,#15017,.T.);
#21707=ORIENTED_EDGE('',*,*,#14887,.T.);
#21708=ORIENTED_EDGE('',*,*,#14889,.T.);
#21709=ORIENTED_EDGE('',*,*,#15016,.T.);
#21710=ORIENTED_EDGE('',*,*,#14879,.T.);
#21711=ORIENTED_EDGE('',*,*,#14881,.T.);
#21712=ORIENTED_EDGE('',*,*,#15015,.T.);
#21713=ORIENTED_EDGE('',*,*,#14871,.T.);
#21714=ORIENTED_EDGE('',*,*,#14873,.T.);
#21715=ORIENTED_EDGE('',*,*,#15014,.T.);
#21716=ORIENTED_EDGE('',*,*,#14863,.T.);
#21717=ORIENTED_EDGE('',*,*,#14865,.T.);
#21718=ORIENTED_EDGE('',*,*,#15013,.T.);
#21719=ORIENTED_EDGE('',*,*,#14855,.T.);
#21720=ORIENTED_EDGE('',*,*,#15041,.F.);
#21721=ORIENTED_EDGE('',*,*,#15042,.T.);
#21722=ORIENTED_EDGE('',*,*,#15043,.F.);
#21723=ORIENTED_EDGE('',*,*,#15042,.F.);
#21724=ORIENTED_EDGE('',*,*,#15044,.F.);
#21725=ORIENTED_EDGE('',*,*,#15045,.T.);
#21726=ORIENTED_EDGE('',*,*,#15046,.T.);
#21727=ORIENTED_EDGE('',*,*,#15047,.F.);
#21728=ORIENTED_EDGE('',*,*,#15048,.F.);
#21729=ORIENTED_EDGE('',*,*,#15049,.T.);
#21730=ORIENTED_EDGE('',*,*,#15050,.T.);
#21731=ORIENTED_EDGE('',*,*,#15045,.F.);
#21732=ORIENTED_EDGE('',*,*,#15051,.F.);
#21733=ORIENTED_EDGE('',*,*,#15052,.T.);
#21734=ORIENTED_EDGE('',*,*,#15053,.T.);
#21735=ORIENTED_EDGE('',*,*,#15049,.F.);
#21736=ORIENTED_EDGE('',*,*,#15054,.F.);
#21737=ORIENTED_EDGE('',*,*,#15055,.T.);
#21738=ORIENTED_EDGE('',*,*,#15056,.T.);
#21739=ORIENTED_EDGE('',*,*,#15052,.F.);
#21740=ORIENTED_EDGE('',*,*,#15057,.F.);
#21741=ORIENTED_EDGE('',*,*,#15058,.T.);
#21742=ORIENTED_EDGE('',*,*,#15059,.T.);
#21743=ORIENTED_EDGE('',*,*,#15055,.F.);
#21744=ORIENTED_EDGE('',*,*,#15060,.F.);
#21745=ORIENTED_EDGE('',*,*,#15047,.T.);
#21746=ORIENTED_EDGE('',*,*,#15061,.T.);
#21747=ORIENTED_EDGE('',*,*,#15058,.F.);
#21748=ORIENTED_EDGE('',*,*,#15061,.F.);
#21749=ORIENTED_EDGE('',*,*,#15046,.F.);
#21750=ORIENTED_EDGE('',*,*,#15050,.F.);
#21751=ORIENTED_EDGE('',*,*,#15053,.F.);
#21752=ORIENTED_EDGE('',*,*,#15056,.F.);
#21753=ORIENTED_EDGE('',*,*,#15059,.F.);
#21754=ORIENTED_EDGE('',*,*,#15043,.T.);
#21755=ORIENTED_EDGE('',*,*,#15062,.F.);
#21756=ORIENTED_EDGE('',*,*,#14590,.F.);
#21757=ORIENTED_EDGE('',*,*,#15063,.T.);
#21758=ORIENTED_EDGE('',*,*,#15062,.T.);
#21759=ORIENTED_EDGE('',*,*,#15063,.F.);
#21760=ORIENTED_EDGE('',*,*,#14641,.T.);
#21761=ORIENTED_EDGE('',*,*,#14706,.T.);
#21762=ORIENTED_EDGE('',*,*,#15064,.F.);
#21763=ORIENTED_EDGE('',*,*,#14712,.T.);
#21764=ORIENTED_EDGE('',*,*,#15065,.F.);
#21765=ORIENTED_EDGE('',*,*,#15066,.T.);
#21766=ORIENTED_EDGE('',*,*,#14703,.T.);
#21767=ORIENTED_EDGE('',*,*,#15064,.T.);
#21768=ORIENTED_EDGE('',*,*,#14704,.T.);
#21769=ORIENTED_EDGE('',*,*,#15066,.F.);
#21770=ORIENTED_EDGE('',*,*,#15012,.F.);
#21771=ORIENTED_EDGE('',*,*,#15065,.T.);
#21772=ORIENTED_EDGE('',*,*,#15040,.T.);
#21773=ORIENTED_EDGE('',*,*,#15044,.T.);
#21774=ORIENTED_EDGE('',*,*,#15060,.T.);
#21775=ORIENTED_EDGE('',*,*,#15057,.T.);
#21776=ORIENTED_EDGE('',*,*,#15054,.T.);
#21777=ORIENTED_EDGE('',*,*,#15051,.T.);
#21778=ORIENTED_EDGE('',*,*,#15048,.T.);
#21971=CONICAL_SURFACE('',#25600,0.4175,0.785398163397448);
#21972=CONICAL_SURFACE('',#25602,0.0923760430703401,1.00831422748172);
#21973=CONICAL_SURFACE('',#25613,0.22,0.785398163397448);
#21974=CONICAL_SURFACE('',#25616,0.255,0.785398163397449);
#23137=ADVANCED_FACE('',(#3398),#1237,.T.);
#23138=ADVANCED_FACE('',(#3399),#1238,.T.);
#23139=ADVANCED_FACE('',(#3400),#1239,.T.);
#23140=ADVANCED_FACE('',(#3401),#1240,.T.);
#23141=ADVANCED_FACE('',(#3402),#1241,.T.);
#23142=ADVANCED_FACE('',(#3403),#1242,.T.);
#23143=ADVANCED_FACE('',(#3404),#1243,.T.);
#23144=ADVANCED_FACE('',(#3405),#1244,.T.);
#23145=ADVANCED_FACE('',(#3406),#1245,.T.);
#23146=ADVANCED_FACE('',(#3407),#1246,.T.);
#23147=ADVANCED_FACE('',(#3408),#1247,.T.);
#23148=ADVANCED_FACE('',(#3409),#1248,.T.);
#23149=ADVANCED_FACE('',(#3410),#1249,.T.);
#23150=ADVANCED_FACE('',(#3411),#1250,.T.);
#23151=ADVANCED_FACE('',(#3412),#1251,.T.);
#23152=ADVANCED_FACE('',(#3413),#1252,.T.);
#23153=ADVANCED_FACE('',(#3414),#1253,.T.);
#23154=ADVANCED_FACE('',(#3415),#1254,.T.);
#23155=ADVANCED_FACE('',(#3416),#1255,.T.);
#23156=ADVANCED_FACE('',(#3417),#1256,.T.);
#23157=ADVANCED_FACE('',(#3418),#1257,.T.);
#23158=ADVANCED_FACE('',(#3419),#1258,.T.);
#23159=ADVANCED_FACE('',(#3420),#1259,.T.);
#23160=ADVANCED_FACE('',(#3421),#1260,.T.);
#23161=ADVANCED_FACE('',(#3422),#1261,.T.);
#23162=ADVANCED_FACE('',(#3423),#1262,.T.);
#23163=ADVANCED_FACE('',(#3424),#1263,.T.);
#23164=ADVANCED_FACE('',(#3425),#1264,.T.);
#23165=ADVANCED_FACE('',(#3426),#1265,.T.);
#23166=ADVANCED_FACE('',(#3427),#1266,.T.);
#23167=ADVANCED_FACE('',(#3428),#1267,.T.);
#23168=ADVANCED_FACE('',(#3429),#1268,.T.);
#23169=ADVANCED_FACE('',(#3430),#1269,.T.);
#23170=ADVANCED_FACE('',(#3431),#1270,.T.);
#23171=ADVANCED_FACE('',(#3432),#1271,.T.);
#23172=ADVANCED_FACE('',(#3433),#1272,.T.);
#23173=ADVANCED_FACE('',(#3434),#1273,.T.);
#23174=ADVANCED_FACE('',(#3435),#2116,.F.);
#23175=ADVANCED_FACE('',(#3436),#371,.F.);
#23176=ADVANCED_FACE('',(#3437),#2117,.T.);
#23177=ADVANCED_FACE('',(#3438),#1274,.T.);
#23178=ADVANCED_FACE('',(#3439),#372,.F.);
#23179=ADVANCED_FACE('',(#3440),#2118,.T.);
#23180=ADVANCED_FACE('',(#3441),#2119,.F.);
#23181=ADVANCED_FACE('',(#3442),#2120,.F.);
#23182=ADVANCED_FACE('',(#3443),#2121,.T.);
#23183=ADVANCED_FACE('',(#3444),#2122,.F.);
#23184=ADVANCED_FACE('',(#3445),#2123,.F.);
#23185=ADVANCED_FACE('',(#3446),#2124,.T.);
#23186=ADVANCED_FACE('',(#3447),#2125,.F.);
#23187=ADVANCED_FACE('',(#3448),#2126,.F.);
#23188=ADVANCED_FACE('',(#3449),#2127,.T.);
#23189=ADVANCED_FACE('',(#3450),#2128,.F.);
#23190=ADVANCED_FACE('',(#3451),#2129,.F.);
#23191=ADVANCED_FACE('',(#3452),#2130,.T.);
#23192=ADVANCED_FACE('',(#3453),#2131,.F.);
#23193=ADVANCED_FACE('',(#3454),#2132,.F.);
#23194=ADVANCED_FACE('',(#3455),#2133,.T.);
#23195=ADVANCED_FACE('',(#3456),#2134,.F.);
#23196=ADVANCED_FACE('',(#3457),#2135,.F.);
#23197=ADVANCED_FACE('',(#3458),#2136,.T.);
#23198=ADVANCED_FACE('',(#3459),#2137,.F.);
#23199=ADVANCED_FACE('',(#3460),#2138,.F.);
#23200=ADVANCED_FACE('',(#3461),#2139,.T.);
#23201=ADVANCED_FACE('',(#3462),#2140,.F.);
#23202=ADVANCED_FACE('',(#3463),#2141,.F.);
#23203=ADVANCED_FACE('',(#3464),#2142,.T.);
#23204=ADVANCED_FACE('',(#3465),#2143,.F.);
#23205=ADVANCED_FACE('',(#3466),#2144,.F.);
#23206=ADVANCED_FACE('',(#3467),#2145,.T.);
#23207=ADVANCED_FACE('',(#3468),#2146,.F.);
#23208=ADVANCED_FACE('',(#3469),#2147,.F.);
#23209=ADVANCED_FACE('',(#3470),#2148,.T.);
#23210=ADVANCED_FACE('',(#3471),#2149,.F.);
#23211=ADVANCED_FACE('',(#3472),#2150,.F.);
#23212=ADVANCED_FACE('',(#3473),#2151,.T.);
#23213=ADVANCED_FACE('',(#3474),#2152,.F.);
#23214=ADVANCED_FACE('',(#3475),#2153,.F.);
#23215=ADVANCED_FACE('',(#3476),#2154,.T.);
#23216=ADVANCED_FACE('',(#3477),#2155,.F.);
#23217=ADVANCED_FACE('',(#3478),#2156,.F.);
#23218=ADVANCED_FACE('',(#3479),#2157,.T.);
#23219=ADVANCED_FACE('',(#3480),#2158,.F.);
#23220=ADVANCED_FACE('',(#3481),#2159,.F.);
#23221=ADVANCED_FACE('',(#3482),#2160,.T.);
#23222=ADVANCED_FACE('',(#3483),#2161,.F.);
#23223=ADVANCED_FACE('',(#3484),#2162,.F.);
#23224=ADVANCED_FACE('',(#3485),#2163,.T.);
#23225=ADVANCED_FACE('',(#3486),#2164,.F.);
#23226=ADVANCED_FACE('',(#3487),#2165,.F.);
#23227=ADVANCED_FACE('',(#3488),#2166,.T.);
#23228=ADVANCED_FACE('',(#3489),#2167,.F.);
#23229=ADVANCED_FACE('',(#3490),#2168,.F.);
#23230=ADVANCED_FACE('',(#3491),#2169,.T.);
#23231=ADVANCED_FACE('',(#3492),#2170,.F.);
#23232=ADVANCED_FACE('',(#3493),#2171,.F.);
#23233=ADVANCED_FACE('',(#3494),#2172,.T.);
#23234=ADVANCED_FACE('',(#3495),#2173,.F.);
#23235=ADVANCED_FACE('',(#3496),#2174,.F.);
#23236=ADVANCED_FACE('',(#3497),#2175,.T.);
#23237=ADVANCED_FACE('',(#3498),#2176,.F.);
#23238=ADVANCED_FACE('',(#3499),#2177,.F.);
#23239=ADVANCED_FACE('',(#3500),#2178,.T.);
#23240=ADVANCED_FACE('',(#3501),#2179,.F.);
#23241=ADVANCED_FACE('',(#3502),#2180,.F.);
#23242=ADVANCED_FACE('',(#3503),#2181,.T.);
#23243=ADVANCED_FACE('',(#3504),#2182,.F.);
#23244=ADVANCED_FACE('',(#3505),#2183,.F.);
#23245=ADVANCED_FACE('',(#3506),#2184,.T.);
#23246=ADVANCED_FACE('',(#3507),#2185,.F.);
#23247=ADVANCED_FACE('',(#3508),#2186,.F.);
#23248=ADVANCED_FACE('',(#3509),#2187,.T.);
#23249=ADVANCED_FACE('',(#3510),#2188,.F.);
#23250=ADVANCED_FACE('',(#3511),#2189,.F.);
#23251=ADVANCED_FACE('',(#3512),#2190,.T.);
#23252=ADVANCED_FACE('',(#3513),#2191,.F.);
#23253=ADVANCED_FACE('',(#3514),#2192,.F.);
#23254=ADVANCED_FACE('',(#3515),#2193,.T.);
#23255=ADVANCED_FACE('',(#3516),#2194,.F.);
#23256=ADVANCED_FACE('',(#3517),#2195,.F.);
#23257=ADVANCED_FACE('',(#3518),#2196,.T.);
#23258=ADVANCED_FACE('',(#3519),#2197,.F.);
#23259=ADVANCED_FACE('',(#3520),#2198,.F.);
#23260=ADVANCED_FACE('',(#3521),#2199,.T.);
#23261=ADVANCED_FACE('',(#3522),#2200,.F.);
#23262=ADVANCED_FACE('',(#3523),#2201,.F.);
#23263=ADVANCED_FACE('',(#3524),#2202,.T.);
#23264=ADVANCED_FACE('',(#3525),#2203,.F.);
#23265=ADVANCED_FACE('',(#3526),#2204,.F.);
#23266=ADVANCED_FACE('',(#3527),#2205,.T.);
#23267=ADVANCED_FACE('',(#3528),#2206,.F.);
#23268=ADVANCED_FACE('',(#3529),#2207,.F.);
#23269=ADVANCED_FACE('',(#3530),#2208,.T.);
#23270=ADVANCED_FACE('',(#3531),#2209,.F.);
#23271=ADVANCED_FACE('',(#3532),#2210,.F.);
#23272=ADVANCED_FACE('',(#3533),#2211,.T.);
#23273=ADVANCED_FACE('',(#3534),#2212,.F.);
#23274=ADVANCED_FACE('',(#3535),#2213,.F.);
#23275=ADVANCED_FACE('',(#3536),#2214,.T.);
#23276=ADVANCED_FACE('',(#3537),#2215,.F.);
#23277=ADVANCED_FACE('',(#3538),#2216,.F.);
#23278=ADVANCED_FACE('',(#3539),#2217,.T.);
#23279=ADVANCED_FACE('',(#3540),#2218,.F.);
#23280=ADVANCED_FACE('',(#3541),#2219,.F.);
#23281=ADVANCED_FACE('',(#3542),#2220,.T.);
#23282=ADVANCED_FACE('',(#3543),#2221,.F.);
#23283=ADVANCED_FACE('',(#3544),#2222,.F.);
#23284=ADVANCED_FACE('',(#3545),#1275,.T.);
#23285=ADVANCED_FACE('',(#3546),#2223,.F.);
#23286=ADVANCED_FACE('',(#3547),#2224,.F.);
#23287=ADVANCED_FACE('',(#3548),#2225,.T.);
#23288=ADVANCED_FACE('',(#3549),#21971,.T.);
#23289=ADVANCED_FACE('',(#3550),#21972,.F.);
#23290=ADVANCED_FACE('',(#3551),#2226,.F.);
#23291=ADVANCED_FACE('',(#3552),#2227,.F.);
#23292=ADVANCED_FACE('',(#3553),#2228,.F.);
#23293=ADVANCED_FACE('',(#3554),#2229,.F.);
#23294=ADVANCED_FACE('',(#3555),#2230,.F.);
#23295=ADVANCED_FACE('',(#3556),#2231,.F.);
#23296=ADVANCED_FACE('',(#3557,#1445),#2232,.F.);
#23297=ADVANCED_FACE('',(#3558),#2233,.T.);
#23298=ADVANCED_FACE('',(#3559),#21973,.T.);
#23299=ADVANCED_FACE('',(#3560),#1276,.T.);
#23300=ADVANCED_FACE('',(#3561),#21974,.T.);
#23301=ADVANCED_FACE('',(#3562,#1446),#2234,.T.);
#23302=ADVANCED_FACE('',(#3563,#1447),#2235,.T.);
#23318=CLOSED_SHELL('',(#23137,#23138,#23139,#23140,#23141,#23142,#23143,
#23144,#23145,#23146,#23147,#23148,#23149,#23150,#23151,#23152,#23153,#23154,
#23155,#23156,#23157,#23158,#23159,#23160,#23161,#23162,#23163,#23164,#23165,
#23166,#23167,#23168,#23169,#23170,#23171,#23172,#23173,#23174,#23175,#23176,
#23177,#23178,#23179,#23180,#23181,#23182,#23183,#23184,#23185,#23186,#23187,
#23188,#23189,#23190,#23191,#23192,#23193,#23194,#23195,#23196,#23197,#23198,
#23199,#23200,#23201,#23202,#23203,#23204,#23205,#23206,#23207,#23208,#23209,
#23210,#23211,#23212,#23213,#23214,#23215,#23216,#23217,#23218,#23219,#23220,
#23221,#23222,#23223,#23224,#23225,#23226,#23227,#23228,#23229,#23230,#23231,
#23232,#23233,#23234,#23235,#23236,#23237,#23238,#23239,#23240,#23241,#23242,
#23243,#23244,#23245,#23246,#23247,#23248,#23249,#23250,#23251,#23252,#23253,
#23254,#23255,#23256,#23257,#23258,#23259,#23260,#23261,#23262,#23263,#23264,
#23265,#23266,#23267,#23268,#23269,#23270,#23271,#23272,#23273,#23274,#23275,
#23276,#23277,#23278,#23279,#23280,#23281,#23282,#23283,#23284,#23285,#23286,
#23287,#23288,#23289,#23290,#23291,#23292,#23293,#23294,#23295,#23296,#23297,
#23298,#23299,#23300,#23301,#23302));
#25369=AXIS2_PLACEMENT_3D('',#50089,#31004,#31005);
#25370=AXIS2_PLACEMENT_3D('',#50090,#31006,#31007);
#25371=AXIS2_PLACEMENT_3D('',#50118,#31009,#31010);
#25372=AXIS2_PLACEMENT_3D('',#50121,#31012,#31013);
#25373=AXIS2_PLACEMENT_3D('',#50123,#31014,#31015);
#25374=AXIS2_PLACEMENT_3D('',#50143,#31016,#31017);
#25375=AXIS2_PLACEMENT_3D('',#50191,#31019,#31020);
#25376=AXIS2_PLACEMENT_3D('',#50239,#31022,#31023);
#25377=AXIS2_PLACEMENT_3D('',#50287,#31025,#31026);
#25378=AXIS2_PLACEMENT_3D('',#50341,#31028,#31029);
#25379=AXIS2_PLACEMENT_3D('',#50389,#31031,#31032);
#25380=AXIS2_PLACEMENT_3D('',#50437,#31034,#31035);
#25381=AXIS2_PLACEMENT_3D('',#50491,#31037,#31038);
#25382=AXIS2_PLACEMENT_3D('',#50539,#31040,#31041);
#25383=AXIS2_PLACEMENT_3D('',#50587,#31043,#31044);
#25384=AXIS2_PLACEMENT_3D('',#50635,#31046,#31047);
#25385=AXIS2_PLACEMENT_3D('',#50689,#31049,#31050);
#25386=AXIS2_PLACEMENT_3D('',#50737,#31052,#31053);
#25387=AXIS2_PLACEMENT_3D('',#50785,#31055,#31056);
#25388=AXIS2_PLACEMENT_3D('',#50839,#31058,#31059);
#25389=AXIS2_PLACEMENT_3D('',#50887,#31061,#31062);
#25390=AXIS2_PLACEMENT_3D('',#50935,#31064,#31065);
#25391=AXIS2_PLACEMENT_3D('',#50983,#31067,#31068);
#25392=AXIS2_PLACEMENT_3D('',#50996,#31070,#31071);
#25393=AXIS2_PLACEMENT_3D('',#51002,#31072,#31073);
#25394=AXIS2_PLACEMENT_3D('',#51027,#31075,#31076);
#25395=AXIS2_PLACEMENT_3D('',#51051,#31078,#31079);
#25396=AXIS2_PLACEMENT_3D('',#51075,#31081,#31082);
#25397=AXIS2_PLACEMENT_3D('',#51100,#31084,#31085);
#25398=AXIS2_PLACEMENT_3D('',#51125,#31087,#31088);
#25399=AXIS2_PLACEMENT_3D('',#51149,#31090,#31091);
#25400=AXIS2_PLACEMENT_3D('',#51174,#31093,#31094);
#25401=AXIS2_PLACEMENT_3D('',#51199,#31096,#31097);
#25402=AXIS2_PLACEMENT_3D('',#51223,#31099,#31100);
#25403=AXIS2_PLACEMENT_3D('',#51247,#31102,#31103);
#25404=AXIS2_PLACEMENT_3D('',#51272,#31105,#31106);
#25405=AXIS2_PLACEMENT_3D('',#51297,#31108,#31109);
#25406=AXIS2_PLACEMENT_3D('',#51321,#31111,#31112);
#25407=AXIS2_PLACEMENT_3D('',#51346,#31114,#31115);
#25408=AXIS2_PLACEMENT_3D('',#51371,#31117,#31118);
#25409=AXIS2_PLACEMENT_3D('',#51395,#31120,#31121);
#25410=AXIS2_PLACEMENT_3D('',#51419,#31123,#31124);
#25411=AXIS2_PLACEMENT_3D('',#51444,#31126,#31127);
#25412=AXIS2_PLACEMENT_3D('',#51505,#31128,#31129);
#25413=AXIS2_PLACEMENT_3D('',#51507,#31130,#31131);
#25414=AXIS2_PLACEMENT_3D('',#52146,#31132,#31133);
#25415=AXIS2_PLACEMENT_3D('',#52206,#31134,#31135);
#25416=AXIS2_PLACEMENT_3D('',#52207,#31136,#31137);
#25417=AXIS2_PLACEMENT_3D('',#52724,#31138,#31139);
#25418=AXIS2_PLACEMENT_3D('',#52727,#31140,#31141);
#25419=AXIS2_PLACEMENT_3D('',#52731,#31144,#31145);
#25420=AXIS2_PLACEMENT_3D('',#52739,#31148,#31149);
#25421=AXIS2_PLACEMENT_3D('',#52745,#31151,#31152);
#25422=AXIS2_PLACEMENT_3D('',#52748,#31153,#31154);
#25423=AXIS2_PLACEMENT_3D('',#52752,#31157,#31158);
#25424=AXIS2_PLACEMENT_3D('',#52760,#31161,#31162);
#25425=AXIS2_PLACEMENT_3D('',#52766,#31164,#31165);
#25426=AXIS2_PLACEMENT_3D('',#52769,#31166,#31167);
#25427=AXIS2_PLACEMENT_3D('',#52773,#31170,#31171);
#25428=AXIS2_PLACEMENT_3D('',#52781,#31174,#31175);
#25429=AXIS2_PLACEMENT_3D('',#52787,#31177,#31178);
#25430=AXIS2_PLACEMENT_3D('',#52790,#31179,#31180);
#25431=AXIS2_PLACEMENT_3D('',#52794,#31183,#31184);
#25432=AXIS2_PLACEMENT_3D('',#52802,#31187,#31188);
#25433=AXIS2_PLACEMENT_3D('',#52808,#31190,#31191);
#25434=AXIS2_PLACEMENT_3D('',#52811,#31192,#31193);
#25435=AXIS2_PLACEMENT_3D('',#52815,#31196,#31197);
#25436=AXIS2_PLACEMENT_3D('',#52823,#31200,#31201);
#25437=AXIS2_PLACEMENT_3D('',#52829,#31203,#31204);
#25438=AXIS2_PLACEMENT_3D('',#52832,#31205,#31206);
#25439=AXIS2_PLACEMENT_3D('',#52836,#31209,#31210);
#25440=AXIS2_PLACEMENT_3D('',#52844,#31213,#31214);
#25441=AXIS2_PLACEMENT_3D('',#52850,#31216,#31217);
#25442=AXIS2_PLACEMENT_3D('',#52853,#31218,#31219);
#25443=AXIS2_PLACEMENT_3D('',#52857,#31222,#31223);
#25444=AXIS2_PLACEMENT_3D('',#52865,#31226,#31227);
#25445=AXIS2_PLACEMENT_3D('',#52871,#31229,#31230);
#25446=AXIS2_PLACEMENT_3D('',#52874,#31231,#31232);
#25447=AXIS2_PLACEMENT_3D('',#52878,#31235,#31236);
#25448=AXIS2_PLACEMENT_3D('',#52886,#31239,#31240);
#25449=AXIS2_PLACEMENT_3D('',#52892,#31242,#31243);
#25450=AXIS2_PLACEMENT_3D('',#52895,#31244,#31245);
#25451=AXIS2_PLACEMENT_3D('',#52899,#31248,#31249);
#25452=AXIS2_PLACEMENT_3D('',#52907,#31252,#31253);
#25453=AXIS2_PLACEMENT_3D('',#52913,#31255,#31256);
#25454=AXIS2_PLACEMENT_3D('',#52916,#31257,#31258);
#25455=AXIS2_PLACEMENT_3D('',#52920,#31261,#31262);
#25456=AXIS2_PLACEMENT_3D('',#52928,#31265,#31266);
#25457=AXIS2_PLACEMENT_3D('',#52934,#31268,#31269);
#25458=AXIS2_PLACEMENT_3D('',#52937,#31270,#31271);
#25459=AXIS2_PLACEMENT_3D('',#52941,#31274,#31275);
#25460=AXIS2_PLACEMENT_3D('',#52949,#31278,#31279);
#25461=AXIS2_PLACEMENT_3D('',#52955,#31281,#31282);
#25462=AXIS2_PLACEMENT_3D('',#52958,#31283,#31284);
#25463=AXIS2_PLACEMENT_3D('',#52962,#31287,#31288);
#25464=AXIS2_PLACEMENT_3D('',#52970,#31291,#31292);
#25465=AXIS2_PLACEMENT_3D('',#52976,#31294,#31295);
#25466=AXIS2_PLACEMENT_3D('',#52979,#31296,#31297);
#25467=AXIS2_PLACEMENT_3D('',#52983,#31300,#31301);
#25468=AXIS2_PLACEMENT_3D('',#52991,#31304,#31305);
#25469=AXIS2_PLACEMENT_3D('',#52997,#31307,#31308);
#25470=AXIS2_PLACEMENT_3D('',#53000,#31309,#31310);
#25471=AXIS2_PLACEMENT_3D('',#53004,#31313,#31314);
#25472=AXIS2_PLACEMENT_3D('',#53012,#31317,#31318);
#25473=AXIS2_PLACEMENT_3D('',#53018,#31320,#31321);
#25474=AXIS2_PLACEMENT_3D('',#53021,#31322,#31323);
#25475=AXIS2_PLACEMENT_3D('',#53025,#31326,#31327);
#25476=AXIS2_PLACEMENT_3D('',#53033,#31330,#31331);
#25477=AXIS2_PLACEMENT_3D('',#53039,#31333,#31334);
#25478=AXIS2_PLACEMENT_3D('',#53042,#31335,#31336);
#25479=AXIS2_PLACEMENT_3D('',#53046,#31339,#31340);
#25480=AXIS2_PLACEMENT_3D('',#53054,#31343,#31344);
#25481=AXIS2_PLACEMENT_3D('',#53060,#31346,#31347);
#25482=AXIS2_PLACEMENT_3D('',#53063,#31348,#31349);
#25483=AXIS2_PLACEMENT_3D('',#53067,#31352,#31353);
#25484=AXIS2_PLACEMENT_3D('',#53075,#31356,#31357);
#25485=AXIS2_PLACEMENT_3D('',#53081,#31359,#31360);
#25486=AXIS2_PLACEMENT_3D('',#53084,#31361,#31362);
#25487=AXIS2_PLACEMENT_3D('',#53089,#31365,#31366);
#25488=AXIS2_PLACEMENT_3D('',#53090,#31367,#31368);
#25489=AXIS2_PLACEMENT_3D('',#53098,#31371,#31372);
#25490=AXIS2_PLACEMENT_3D('',#53104,#31374,#31375);
#25491=AXIS2_PLACEMENT_3D('',#53107,#31376,#31377);
#25492=AXIS2_PLACEMENT_3D('',#53111,#31380,#31381);
#25493=AXIS2_PLACEMENT_3D('',#53119,#31384,#31385);
#25494=AXIS2_PLACEMENT_3D('',#53125,#31387,#31388);
#25495=AXIS2_PLACEMENT_3D('',#53128,#31389,#31390);
#25496=AXIS2_PLACEMENT_3D('',#53132,#31393,#31394);
#25497=AXIS2_PLACEMENT_3D('',#53140,#31397,#31398);
#25498=AXIS2_PLACEMENT_3D('',#53146,#31400,#31401);
#25499=AXIS2_PLACEMENT_3D('',#53149,#31402,#31403);
#25500=AXIS2_PLACEMENT_3D('',#53153,#31406,#31407);
#25501=AXIS2_PLACEMENT_3D('',#53161,#31410,#31411);
#25502=AXIS2_PLACEMENT_3D('',#53167,#31413,#31414);
#25503=AXIS2_PLACEMENT_3D('',#53170,#31415,#31416);
#25504=AXIS2_PLACEMENT_3D('',#53174,#31419,#31420);
#25505=AXIS2_PLACEMENT_3D('',#53182,#31423,#31424);
#25506=AXIS2_PLACEMENT_3D('',#53188,#31426,#31427);
#25507=AXIS2_PLACEMENT_3D('',#53191,#31428,#31429);
#25508=AXIS2_PLACEMENT_3D('',#53195,#31432,#31433);
#25509=AXIS2_PLACEMENT_3D('',#53203,#31436,#31437);
#25510=AXIS2_PLACEMENT_3D('',#53209,#31439,#31440);
#25511=AXIS2_PLACEMENT_3D('',#53212,#31441,#31442);
#25512=AXIS2_PLACEMENT_3D('',#53216,#31445,#31446);
#25513=AXIS2_PLACEMENT_3D('',#53224,#31449,#31450);
#25514=AXIS2_PLACEMENT_3D('',#53230,#31452,#31453);
#25515=AXIS2_PLACEMENT_3D('',#53233,#31454,#31455);
#25516=AXIS2_PLACEMENT_3D('',#53237,#31458,#31459);
#25517=AXIS2_PLACEMENT_3D('',#53245,#31462,#31463);
#25518=AXIS2_PLACEMENT_3D('',#53251,#31465,#31466);
#25519=AXIS2_PLACEMENT_3D('',#53254,#31467,#31468);
#25520=AXIS2_PLACEMENT_3D('',#53258,#31471,#31472);
#25521=AXIS2_PLACEMENT_3D('',#53266,#31475,#31476);
#25522=AXIS2_PLACEMENT_3D('',#53272,#31478,#31479);
#25523=AXIS2_PLACEMENT_3D('',#53275,#31480,#31481);
#25524=AXIS2_PLACEMENT_3D('',#53279,#31484,#31485);
#25525=AXIS2_PLACEMENT_3D('',#53287,#31488,#31489);
#25526=AXIS2_PLACEMENT_3D('',#53293,#31491,#31492);
#25527=AXIS2_PLACEMENT_3D('',#53296,#31493,#31494);
#25528=AXIS2_PLACEMENT_3D('',#53300,#31497,#31498);
#25529=AXIS2_PLACEMENT_3D('',#53308,#31501,#31502);
#25530=AXIS2_PLACEMENT_3D('',#53314,#31504,#31505);
#25531=AXIS2_PLACEMENT_3D('',#53317,#31506,#31507);
#25532=AXIS2_PLACEMENT_3D('',#53321,#31510,#31511);
#25533=AXIS2_PLACEMENT_3D('',#53329,#31514,#31515);
#25534=AXIS2_PLACEMENT_3D('',#53335,#31517,#31518);
#25535=AXIS2_PLACEMENT_3D('',#53338,#31519,#31520);
#25536=AXIS2_PLACEMENT_3D('',#53342,#31523,#31524);
#25537=AXIS2_PLACEMENT_3D('',#53350,#31527,#31528);
#25538=AXIS2_PLACEMENT_3D('',#53356,#31530,#31531);
#25539=AXIS2_PLACEMENT_3D('',#53359,#31532,#31533);
#25540=AXIS2_PLACEMENT_3D('',#53363,#31536,#31537);
#25541=AXIS2_PLACEMENT_3D('',#53371,#31540,#31541);
#25542=AXIS2_PLACEMENT_3D('',#53377,#31543,#31544);
#25543=AXIS2_PLACEMENT_3D('',#53380,#31545,#31546);
#25544=AXIS2_PLACEMENT_3D('',#53384,#31549,#31550);
#25545=AXIS2_PLACEMENT_3D('',#53392,#31553,#31554);
#25546=AXIS2_PLACEMENT_3D('',#53398,#31556,#31557);
#25547=AXIS2_PLACEMENT_3D('',#53401,#31558,#31559);
#25548=AXIS2_PLACEMENT_3D('',#53405,#31562,#31563);
#25549=AXIS2_PLACEMENT_3D('',#53413,#31566,#31567);
#25550=AXIS2_PLACEMENT_3D('',#53419,#31569,#31570);
#25551=AXIS2_PLACEMENT_3D('',#53422,#31571,#31572);
#25552=AXIS2_PLACEMENT_3D('',#53426,#31575,#31576);
#25553=AXIS2_PLACEMENT_3D('',#53434,#31579,#31580);
#25554=AXIS2_PLACEMENT_3D('',#53440,#31582,#31583);
#25555=AXIS2_PLACEMENT_3D('',#53443,#31584,#31585);
#25556=AXIS2_PLACEMENT_3D('',#53447,#31588,#31589);
#25557=AXIS2_PLACEMENT_3D('',#53455,#31592,#31593);
#25558=AXIS2_PLACEMENT_3D('',#53461,#31595,#31596);
#25559=AXIS2_PLACEMENT_3D('',#53462,#31597,#31598);
#25560=AXIS2_PLACEMENT_3D('',#53463,#31599,#31600);
#25561=AXIS2_PLACEMENT_3D('',#53464,#31601,#31602);
#25562=AXIS2_PLACEMENT_3D('',#53465,#31603,#31604);
#25563=AXIS2_PLACEMENT_3D('',#53466,#31605,#31606);
#25564=AXIS2_PLACEMENT_3D('',#53467,#31607,#31608);
#25565=AXIS2_PLACEMENT_3D('',#53468,#31609,#31610);
#25566=AXIS2_PLACEMENT_3D('',#53469,#31611,#31612);
#25567=AXIS2_PLACEMENT_3D('',#53470,#31613,#31614);
#25568=AXIS2_PLACEMENT_3D('',#53471,#31615,#31616);
#25569=AXIS2_PLACEMENT_3D('',#53472,#31617,#31618);
#25570=AXIS2_PLACEMENT_3D('',#53473,#31619,#31620);
#25571=AXIS2_PLACEMENT_3D('',#53474,#31621,#31622);
#25572=AXIS2_PLACEMENT_3D('',#53475,#31623,#31624);
#25573=AXIS2_PLACEMENT_3D('',#53476,#31625,#31626);
#25574=AXIS2_PLACEMENT_3D('',#53477,#31627,#31628);
#25575=AXIS2_PLACEMENT_3D('',#53478,#31629,#31630);
#25576=AXIS2_PLACEMENT_3D('',#53481,#31632,#31633);
#25577=AXIS2_PLACEMENT_3D('',#53482,#31634,#31635);
#25578=AXIS2_PLACEMENT_3D('',#53483,#31636,#31637);
#25579=AXIS2_PLACEMENT_3D('',#53484,#31638,#31639);
#25580=AXIS2_PLACEMENT_3D('',#53485,#31640,#31641);
#25581=AXIS2_PLACEMENT_3D('',#53486,#31642,#31643);
#25582=AXIS2_PLACEMENT_3D('',#53487,#31644,#31645);
#25583=AXIS2_PLACEMENT_3D('',#53488,#31646,#31647);
#25584=AXIS2_PLACEMENT_3D('',#53489,#31648,#31649);
#25585=AXIS2_PLACEMENT_3D('',#53490,#31650,#31651);
#25586=AXIS2_PLACEMENT_3D('',#53491,#31652,#31653);
#25587=AXIS2_PLACEMENT_3D('',#53492,#31654,#31655);
#25588=AXIS2_PLACEMENT_3D('',#53493,#31656,#31657);
#25589=AXIS2_PLACEMENT_3D('',#53494,#31658,#31659);
#25590=AXIS2_PLACEMENT_3D('',#53495,#31660,#31661);
#25591=AXIS2_PLACEMENT_3D('',#53496,#31662,#31663);
#25592=AXIS2_PLACEMENT_3D('',#53497,#31664,#31665);
#25593=AXIS2_PLACEMENT_3D('',#53498,#31666,#31667);
#25594=AXIS2_PLACEMENT_3D('',#53500,#31668,#31669);
#25595=AXIS2_PLACEMENT_3D('',#53504,#31671,#31672);
#25596=AXIS2_PLACEMENT_3D('',#53507,#31674,#31675);
#25597=AXIS2_PLACEMENT_3D('',#53508,#31676,#31677);
#25598=AXIS2_PLACEMENT_3D('',#53516,#31680,#31681);
#25599=AXIS2_PLACEMENT_3D('',#53521,#31683,#31684);
#25600=AXIS2_PLACEMENT_3D('',#53522,#31685,#31686);
#25601=AXIS2_PLACEMENT_3D('',#53524,#31687,#31688);
#25602=AXIS2_PLACEMENT_3D('',#53526,#31690,#31691);
#25603=AXIS2_PLACEMENT_3D('',#53530,#31693,#31694);
#25604=AXIS2_PLACEMENT_3D('',#53531,#31695,#31696);
#25605=AXIS2_PLACEMENT_3D('',#53540,#31701,#31702);
#25606=AXIS2_PLACEMENT_3D('',#53546,#31706,#31707);
#25607=AXIS2_PLACEMENT_3D('',#53552,#31711,#31712);
#25608=AXIS2_PLACEMENT_3D('',#53558,#31716,#31717);
#25609=AXIS2_PLACEMENT_3D('',#53564,#31721,#31722);
#25610=AXIS2_PLACEMENT_3D('',#53567,#31725,#31726);
#25611=AXIS2_PLACEMENT_3D('',#53568,#31727,#31728);
#25612=AXIS2_PLACEMENT_3D('',#53570,#31729,#31730);
#25613=AXIS2_PLACEMENT_3D('',#53571,#31731,#31732);
#25614=AXIS2_PLACEMENT_3D('',#53573,#31734,#31735);
#25615=AXIS2_PLACEMENT_3D('',#53574,#31736,#31737);
#25616=AXIS2_PLACEMENT_3D('',#53575,#31738,#31739);
#25617=AXIS2_PLACEMENT_3D('',#53577,#31740,#31741);
#25618=AXIS2_PLACEMENT_3D('',#53579,#31743,#31744);
#25619=AXIS2_PLACEMENT_3D('',#53580,#31745,#31746);
#31004=DIRECTION('axis',(0.,0.,1.));
#31005=DIRECTION('refdir',(1.,0.,0.));
#31006=DIRECTION('center_axis',(0.,0.,1.));
#31007=DIRECTION('ref_axis',(1.,0.,0.));
#31008=DIRECTION('',(0.,0.,-1.));
#31009=DIRECTION('center_axis',(0.,0.,-1.));
#31010=DIRECTION('ref_axis',(1.,0.,0.));
#31011=DIRECTION('',(0.,0.,-1.));
#31012=DIRECTION('center_axis',(0.,0.,1.));
#31013=DIRECTION('ref_axis',(1.,0.,0.));
#31014=DIRECTION('center_axis',(0.,0.,-1.));
#31015=DIRECTION('ref_axis',(1.,0.,0.));
#31016=DIRECTION('center_axis',(0.,0.,1.));
#31017=DIRECTION('ref_axis',(1.,0.,0.));
#31018=DIRECTION('',(0.,0.,-1.));
#31019=DIRECTION('center_axis',(0.,0.,1.));
#31020=DIRECTION('ref_axis',(1.,0.,0.));
#31021=DIRECTION('',(0.,0.,-1.));
#31022=DIRECTION('center_axis',(0.,0.,1.));
#31023=DIRECTION('ref_axis',(1.,0.,0.));
#31024=DIRECTION('',(0.,0.,-1.));
#31025=DIRECTION('center_axis',(0.,0.,1.));
#31026=DIRECTION('ref_axis',(1.,0.,0.));
#31027=DIRECTION('',(0.,0.,-1.));
#31028=DIRECTION('center_axis',(0.,0.,1.));
#31029=DIRECTION('ref_axis',(1.,0.,0.));
#31030=DIRECTION('',(0.,0.,-1.));
#31031=DIRECTION('center_axis',(0.,0.,1.));
#31032=DIRECTION('ref_axis',(1.,0.,0.));
#31033=DIRECTION('',(0.,0.,-1.));
#31034=DIRECTION('center_axis',(0.,0.,1.));
#31035=DIRECTION('ref_axis',(1.,0.,0.));
#31036=DIRECTION('',(0.,0.,-1.));
#31037=DIRECTION('center_axis',(0.,0.,1.));
#31038=DIRECTION('ref_axis',(1.,0.,0.));
#31039=DIRECTION('',(0.,0.,-1.));
#31040=DIRECTION('center_axis',(0.,0.,1.));
#31041=DIRECTION('ref_axis',(1.,0.,0.));
#31042=DIRECTION('',(0.,0.,-1.));
#31043=DIRECTION('center_axis',(0.,0.,1.));
#31044=DIRECTION('ref_axis',(1.,0.,0.));
#31045=DIRECTION('',(0.,0.,-1.));
#31046=DIRECTION('center_axis',(0.,0.,1.));
#31047=DIRECTION('ref_axis',(1.,0.,0.));
#31048=DIRECTION('',(0.,0.,-1.));
#31049=DIRECTION('center_axis',(0.,0.,1.));
#31050=DIRECTION('ref_axis',(1.,0.,0.));
#31051=DIRECTION('',(0.,0.,-1.));
#31052=DIRECTION('center_axis',(0.,0.,1.));
#31053=DIRECTION('ref_axis',(1.,0.,0.));
#31054=DIRECTION('',(0.,0.,-1.));
#31055=DIRECTION('center_axis',(0.,0.,1.));
#31056=DIRECTION('ref_axis',(1.,0.,0.));
#31057=DIRECTION('',(0.,0.,-1.));
#31058=DIRECTION('center_axis',(0.,0.,1.));
#31059=DIRECTION('ref_axis',(1.,0.,0.));
#31060=DIRECTION('',(0.,0.,-1.));
#31061=DIRECTION('center_axis',(0.,0.,1.));
#31062=DIRECTION('ref_axis',(1.,0.,0.));
#31063=DIRECTION('',(0.,0.,-1.));
#31064=DIRECTION('center_axis',(0.,0.,1.));
#31065=DIRECTION('ref_axis',(1.,0.,0.));
#31066=DIRECTION('',(0.,0.,-1.));
#31067=DIRECTION('center_axis',(0.,0.,1.));
#31068=DIRECTION('ref_axis',(-0.082458823014217,-0.99659447244459,0.));
#31069=DIRECTION('',(0.,0.,1.));
#31070=DIRECTION('center_axis',(0.,0.,1.));
#31071=DIRECTION('ref_axis',(1.,1.20322412993372E-13,0.));
#31072=DIRECTION('center_axis',(0.,0.,1.));
#31073=DIRECTION('ref_axis',(1.,1.20322412993372E-13,0.));
#31074=DIRECTION('',(0.,0.,1.));
#31075=DIRECTION('center_axis',(0.,0.,1.));
#31076=DIRECTION('ref_axis',(1.,1.20322412993372E-13,0.));
#31077=DIRECTION('',(0.,0.,1.));
#31078=DIRECTION('center_axis',(0.,0.,1.));
#31079=DIRECTION('ref_axis',(1.,1.20322412993372E-13,0.));
#31080=DIRECTION('',(0.,0.,1.));
#31081=DIRECTION('center_axis',(0.,0.,1.));
#31082=DIRECTION('ref_axis',(1.,1.20322412993372E-13,0.));
#31083=DIRECTION('',(0.,0.,1.));
#31084=DIRECTION('center_axis',(0.,0.,1.));
#31085=DIRECTION('ref_axis',(1.,1.20322412993372E-13,0.));
#31086=DIRECTION('',(0.,0.,1.));
#31087=DIRECTION('center_axis',(0.,0.,1.));
#31088=DIRECTION('ref_axis',(1.,1.20322412993372E-13,0.));
#31089=DIRECTION('',(0.,0.,1.));
#31090=DIRECTION('center_axis',(0.,0.,1.));
#31091=DIRECTION('ref_axis',(1.,1.20322412993372E-13,0.));
#31092=DIRECTION('',(0.,0.,1.));
#31093=DIRECTION('center_axis',(0.,0.,1.));
#31094=DIRECTION('ref_axis',(1.,1.20322412993372E-13,0.));
#31095=DIRECTION('',(0.,0.,1.));
#31096=DIRECTION('center_axis',(0.,0.,1.));
#31097=DIRECTION('ref_axis',(1.,1.20322412993372E-13,0.));
#31098=DIRECTION('',(0.,0.,1.));
#31099=DIRECTION('center_axis',(0.,0.,1.));
#31100=DIRECTION('ref_axis',(1.,1.20322412993372E-13,0.));
#31101=DIRECTION('',(0.,0.,1.));
#31102=DIRECTION('center_axis',(0.,0.,1.));
#31103=DIRECTION('ref_axis',(1.,1.20322412993372E-13,0.));
#31104=DIRECTION('',(0.,0.,1.));
#31105=DIRECTION('center_axis',(0.,0.,1.));
#31106=DIRECTION('ref_axis',(1.,1.20322412993372E-13,0.));
#31107=DIRECTION('',(0.,0.,1.));
#31108=DIRECTION('center_axis',(0.,0.,1.));
#31109=DIRECTION('ref_axis',(1.,1.20322412993372E-13,0.));
#31110=DIRECTION('',(0.,0.,1.));
#31111=DIRECTION('center_axis',(0.,0.,1.));
#31112=DIRECTION('ref_axis',(1.,1.20322412993372E-13,0.));
#31113=DIRECTION('',(0.,0.,1.));
#31114=DIRECTION('center_axis',(0.,0.,1.));
#31115=DIRECTION('ref_axis',(1.,1.20322412993372E-13,0.));
#31116=DIRECTION('',(0.,0.,1.));
#31117=DIRECTION('center_axis',(0.,0.,1.));
#31118=DIRECTION('ref_axis',(1.,1.20322412993372E-13,0.));
#31119=DIRECTION('',(0.,0.,1.));
#31120=DIRECTION('center_axis',(0.,0.,1.));
#31121=DIRECTION('ref_axis',(1.,1.20322412993372E-13,0.));
#31122=DIRECTION('',(0.,0.,1.));
#31123=DIRECTION('center_axis',(0.,0.,1.));
#31124=DIRECTION('ref_axis',(1.,1.20322412993372E-13,0.));
#31125=DIRECTION('',(0.,0.,1.));
#31126=DIRECTION('center_axis',(0.,0.,1.));
#31127=DIRECTION('ref_axis',(1.,0.,0.));
#31128=DIRECTION('center_axis',(0.,0.,1.));
#31129=DIRECTION('ref_axis',(1.,0.,0.));
#31130=DIRECTION('center_axis',(0.,0.,1.));
#31131=DIRECTION('ref_axis',(1.,0.,0.));
#31132=DIRECTION('center_axis',(0.,0.,1.));
#31133=DIRECTION('ref_axis',(1.,0.,0.));
#31134=DIRECTION('center_axis',(0.,0.,-1.));
#31135=DIRECTION('ref_axis',(1.,1.20322412993372E-13,0.));
#31136=DIRECTION('center_axis',(0.,0.,1.));
#31137=DIRECTION('ref_axis',(-0.0824588795393025,0.996594467767669,0.));
#31138=DIRECTION('center_axis',(0.,0.,1.));
#31139=DIRECTION('ref_axis',(0.984807753012208,-0.17364817766693,0.));
#31140=DIRECTION('center_axis',(0.,0.,-1.));
#31141=DIRECTION('ref_axis',(1.,0.,0.));
#31142=DIRECTION('',(-0.996089805327885,-0.0883464754353937,0.));
#31143=DIRECTION('',(0.905801965515954,-0.423701309022564,0.));
#31144=DIRECTION('center_axis',(-0.423701309022564,-0.905801965515954,0.));
#31145=DIRECTION('ref_axis',(0.905801965515954,-0.423701309022564,0.));
#31146=DIRECTION('',(0.,0.,1.));
#31147=DIRECTION('',(0.,0.,1.));
#31148=DIRECTION('center_axis',(-0.0883464754353937,0.996089805327885,0.));
#31149=DIRECTION('ref_axis',(-0.996089805327885,-0.0883464754353937,0.));
#31150=DIRECTION('',(0.,0.,-1.));
#31151=DIRECTION('center_axis',(0.,0.,1.));
#31152=DIRECTION('ref_axis',(0.939692620785908,-0.342020143325669,0.));
#31153=DIRECTION('center_axis',(0.,0.,-1.));
#31154=DIRECTION('ref_axis',(1.,0.,0.));
#31155=DIRECTION('',(-0.996298167445974,0.0859648855277171,0.));
#31156=DIRECTION('',(0.818465838146947,-0.574555194725812,0.));
#31157=DIRECTION('center_axis',(-0.574555194725812,-0.818465838146947,0.));
#31158=DIRECTION('ref_axis',(0.818465838146947,-0.574555194725812,0.));
#31159=DIRECTION('',(0.,0.,1.));
#31160=DIRECTION('',(0.,0.,1.));
#31161=DIRECTION('center_axis',(0.0859648855277171,0.996298167445974,0.));
#31162=DIRECTION('ref_axis',(-0.996298167445974,0.0859648855277171,0.));
#31163=DIRECTION('',(0.,0.,-1.));
#31164=DIRECTION('center_axis',(0.,0.,1.));
#31165=DIRECTION('ref_axis',(0.866025403784438,-0.5,0.));
#31166=DIRECTION('center_axis',(0.,0.,-1.));
#31167=DIRECTION('ref_axis',(1.,0.,0.));
#31168=DIRECTION('',(-0.966234513897416,0.257664246944398,0.));
#31169=DIRECTION('',(0.706261040449543,-0.707951511576272,0.));
#31170=DIRECTION('center_axis',(-0.707951511576272,-0.706261040449543,0.));
#31171=DIRECTION('ref_axis',(0.706261040449543,-0.707951511576272,0.));
#31172=DIRECTION('',(0.,0.,1.));
#31173=DIRECTION('',(0.,0.,1.));
#31174=DIRECTION('center_axis',(0.257664246944398,0.966234513897416,0.));
#31175=DIRECTION('ref_axis',(-0.966234513897416,0.257664246944398,0.));
#31176=DIRECTION('',(0.,0.,-1.));
#31177=DIRECTION('center_axis',(0.,0.,1.));
#31178=DIRECTION('ref_axis',(0.766044443118978,-0.64278760968654,0.));
#31179=DIRECTION('center_axis',(0.,0.,-1.));
#31180=DIRECTION('ref_axis',(1.,0.,0.));
#31181=DIRECTION('',(-0.906812313582341,0.421534610602074,0.));
#31182=DIRECTION('',(0.57259685842341,-0.819837079988238,0.));
#31183=DIRECTION('center_axis',(-0.819837079988238,-0.57259685842341,0.));
#31184=DIRECTION('ref_axis',(0.57259685842341,-0.819837079988238,0.));
#31185=DIRECTION('',(0.,0.,1.));
#31186=DIRECTION('',(0.,0.,1.));
#31187=DIRECTION('center_axis',(0.421534610602074,0.906812313582341,0.));
#31188=DIRECTION('ref_axis',(-0.906812313582341,0.421534610602074,0.));
#31189=DIRECTION('',(0.,0.,-1.));
#31190=DIRECTION('center_axis',(0.,0.,1.));
#31191=DIRECTION('ref_axis',(0.642787609686539,-0.766044443118978,0.));
#31192=DIRECTION('center_axis',(0.,0.,-1.));
#31193=DIRECTION('ref_axis',(1.,0.,0.));
#31194=DIRECTION('',(-0.819837079988238,0.572596858423411,0.));
#31195=DIRECTION('',(0.421534610602073,-0.906812313582341,0.));
#31196=DIRECTION('center_axis',(-0.906812313582341,-0.421534610602073,0.));
#31197=DIRECTION('ref_axis',(0.421534610602073,-0.906812313582341,0.));
#31198=DIRECTION('',(0.,0.,1.));
#31199=DIRECTION('',(0.,0.,1.));
#31200=DIRECTION('center_axis',(0.572596858423411,0.819837079988238,0.));
#31201=DIRECTION('ref_axis',(-0.819837079988238,0.572596858423411,0.));
#31202=DIRECTION('',(0.,0.,-1.));
#31203=DIRECTION('center_axis',(0.,0.,1.));
#31204=DIRECTION('ref_axis',(0.5,-0.866025403784438,0.));
#31205=DIRECTION('center_axis',(0.,0.,-1.));
#31206=DIRECTION('ref_axis',(1.,0.,0.));
#31207=DIRECTION('',(-0.707951511576272,0.706261040449543,0.));
#31208=DIRECTION('',(0.257664246944398,-0.966234513897416,0.));
#31209=DIRECTION('center_axis',(-0.966234513897416,-0.257664246944398,0.));
#31210=DIRECTION('ref_axis',(0.257664246944398,-0.966234513897416,0.));
#31211=DIRECTION('',(0.,0.,1.));
#31212=DIRECTION('',(0.,0.,1.));
#31213=DIRECTION('center_axis',(0.706261040449543,0.707951511576272,0.));
#31214=DIRECTION('ref_axis',(-0.707951511576272,0.706261040449543,0.));
#31215=DIRECTION('',(0.,0.,-1.));
#31216=DIRECTION('center_axis',(0.,0.,1.));
#31217=DIRECTION('ref_axis',(0.342020143325668,-0.939692620785909,0.));
#31218=DIRECTION('center_axis',(0.,0.,-1.));
#31219=DIRECTION('ref_axis',(1.,0.,0.));
#31220=DIRECTION('',(-0.574555194725811,0.818465838146948,0.));
#31221=DIRECTION('',(0.0859648855277157,-0.996298167445974,0.));
#31222=DIRECTION('center_axis',(-0.996298167445974,-0.0859648855277157,
0.));
#31223=DIRECTION('ref_axis',(0.0859648855277157,-0.996298167445974,0.));
#31224=DIRECTION('',(0.,0.,1.));
#31225=DIRECTION('',(0.,0.,1.));
#31226=DIRECTION('center_axis',(0.818465838146948,0.574555194725811,0.));
#31227=DIRECTION('ref_axis',(-0.574555194725811,0.818465838146948,0.));
#31228=DIRECTION('',(0.,0.,-1.));
#31229=DIRECTION('center_axis',(0.,0.,1.));
#31230=DIRECTION('ref_axis',(0.17364817766693,-0.984807753012208,0.));
#31231=DIRECTION('center_axis',(0.,0.,-1.));
#31232=DIRECTION('ref_axis',(1.,0.,0.));
#31233=DIRECTION('',(-0.423701309022563,0.905801965515955,0.));
#31234=DIRECTION('',(-0.0883464754353941,-0.996089805327885,0.));
#31235=DIRECTION('center_axis',(-0.996089805327885,0.0883464754353941,0.));
#31236=DIRECTION('ref_axis',(-0.0883464754353941,-0.996089805327885,0.));
#31237=DIRECTION('',(0.,0.,1.));
#31238=DIRECTION('',(0.,0.,1.));
#31239=DIRECTION('center_axis',(0.905801965515955,0.423701309022563,0.));
#31240=DIRECTION('ref_axis',(-0.423701309022563,0.905801965515955,0.));
#31241=DIRECTION('',(0.,0.,-1.));
#31242=DIRECTION('center_axis',(0.,0.,1.));
#31243=DIRECTION('ref_axis',(-1.94289029309402E-16,-1.,0.));
#31244=DIRECTION('center_axis',(0.,0.,-1.));
#31245=DIRECTION('ref_axis',(1.,0.,0.));
#31246=DIRECTION('',(-0.259973473447873,0.96561575852067,0.));
#31247=DIRECTION('',(-0.259973473447873,-0.96561575852067,0.));
#31248=DIRECTION('center_axis',(-0.96561575852067,0.259973473447873,0.));
#31249=DIRECTION('ref_axis',(-0.259973473447873,-0.96561575852067,0.));
#31250=DIRECTION('',(0.,0.,1.));
#31251=DIRECTION('',(0.,0.,1.));
#31252=DIRECTION('center_axis',(0.96561575852067,0.259973473447873,0.));
#31253=DIRECTION('ref_axis',(-0.259973473447873,0.96561575852067,0.));
#31254=DIRECTION('',(0.,0.,-1.));
#31255=DIRECTION('center_axis',(0.,0.,1.));
#31256=DIRECTION('ref_axis',(-0.17364817766693,-0.984807753012208,0.));
#31257=DIRECTION('center_axis',(0.,0.,-1.));
#31258=DIRECTION('ref_axis',(1.,0.,0.));
#31259=DIRECTION('',(-0.0883464754353937,0.996089805327885,0.));
#31260=DIRECTION('',(-0.423701309022564,-0.905801965515954,0.));
#31261=DIRECTION('center_axis',(-0.905801965515954,0.423701309022564,0.));
#31262=DIRECTION('ref_axis',(-0.423701309022564,-0.905801965515954,0.));
#31263=DIRECTION('',(0.,0.,1.));
#31264=DIRECTION('',(0.,0.,1.));
#31265=DIRECTION('center_axis',(0.996089805327885,0.0883464754353937,0.));
#31266=DIRECTION('ref_axis',(-0.0883464754353937,0.996089805327885,0.));
#31267=DIRECTION('',(0.,0.,-1.));
#31268=DIRECTION('center_axis',(0.,0.,1.));
#31269=DIRECTION('ref_axis',(-0.342020143325669,-0.939692620785908,0.));
#31270=DIRECTION('center_axis',(0.,0.,-1.));
#31271=DIRECTION('ref_axis',(1.,0.,0.));
#31272=DIRECTION('',(0.0859648855277171,0.996298167445974,0.));
#31273=DIRECTION('',(-0.574555194725812,-0.818465838146947,0.));
#31274=DIRECTION('center_axis',(-0.818465838146947,0.574555194725812,0.));
#31275=DIRECTION('ref_axis',(-0.574555194725812,-0.818465838146947,0.));
#31276=DIRECTION('',(0.,0.,1.));
#31277=DIRECTION('',(0.,0.,1.));
#31278=DIRECTION('center_axis',(0.996298167445974,-0.0859648855277171,0.));
#31279=DIRECTION('ref_axis',(0.0859648855277171,0.996298167445974,0.));
#31280=DIRECTION('',(0.,0.,-1.));
#31281=DIRECTION('center_axis',(0.,0.,1.));
#31282=DIRECTION('ref_axis',(-0.5,-0.866025403784438,0.));
#31283=DIRECTION('center_axis',(0.,0.,-1.));
#31284=DIRECTION('ref_axis',(1.,0.,0.));
#31285=DIRECTION('',(0.257664246944398,0.966234513897416,0.));
#31286=DIRECTION('',(-0.707951511576272,-0.706261040449543,0.));
#31287=DIRECTION('center_axis',(-0.706261040449543,0.707951511576272,0.));
#31288=DIRECTION('ref_axis',(-0.707951511576272,-0.706261040449543,0.));
#31289=DIRECTION('',(0.,0.,1.));
#31290=DIRECTION('',(0.,0.,1.));
#31291=DIRECTION('center_axis',(0.966234513897416,-0.257664246944398,0.));
#31292=DIRECTION('ref_axis',(0.257664246944398,0.966234513897416,0.));
#31293=DIRECTION('',(0.,0.,-1.));
#31294=DIRECTION('center_axis',(0.,0.,1.));
#31295=DIRECTION('ref_axis',(-0.642787609686539,-0.766044443118978,0.));
#31296=DIRECTION('center_axis',(0.,0.,-1.));
#31297=DIRECTION('ref_axis',(1.,0.,0.));
#31298=DIRECTION('',(0.421534610602074,0.906812313582341,0.));
#31299=DIRECTION('',(-0.819837079988238,-0.57259685842341,0.));
#31300=DIRECTION('center_axis',(-0.572596858423411,0.819837079988238,0.));
#31301=DIRECTION('ref_axis',(-0.819837079988238,-0.57259685842341,0.));
#31302=DIRECTION('',(0.,0.,1.));
#31303=DIRECTION('',(0.,0.,1.));
#31304=DIRECTION('center_axis',(0.906812313582341,-0.421534610602074,0.));
#31305=DIRECTION('ref_axis',(0.421534610602074,0.906812313582341,0.));
#31306=DIRECTION('',(0.,0.,-1.));
#31307=DIRECTION('center_axis',(0.,0.,1.));
#31308=DIRECTION('ref_axis',(-0.766044443118978,-0.642787609686539,0.));
#31309=DIRECTION('center_axis',(0.,0.,-1.));
#31310=DIRECTION('ref_axis',(1.,0.,0.));
#31311=DIRECTION('',(0.572596858423411,0.819837079988238,0.));
#31312=DIRECTION('',(-0.906812313582341,-0.421534610602073,0.));
#31313=DIRECTION('center_axis',(-0.421534610602074,0.906812313582341,0.));
#31314=DIRECTION('ref_axis',(-0.906812313582341,-0.421534610602073,0.));
#31315=DIRECTION('',(0.,0.,1.));
#31316=DIRECTION('',(0.,0.,1.));
#31317=DIRECTION('center_axis',(0.819837079988238,-0.572596858423411,0.));
#31318=DIRECTION('ref_axis',(0.572596858423411,0.819837079988238,0.));
#31319=DIRECTION('',(0.,0.,-1.));
#31320=DIRECTION('center_axis',(0.,0.,1.));
#31321=DIRECTION('ref_axis',(-0.866025403784439,-0.5,0.));
#31322=DIRECTION('center_axis',(0.,0.,-1.));
#31323=DIRECTION('ref_axis',(1.,0.,0.));
#31324=DIRECTION('',(0.706261040449544,0.707951511576272,0.));
#31325=DIRECTION('',(-0.966234513897416,-0.257664246944397,0.));
#31326=DIRECTION('center_axis',(-0.257664246944397,0.966234513897416,0.));
#31327=DIRECTION('ref_axis',(-0.966234513897416,-0.257664246944397,0.));
#31328=DIRECTION('',(0.,0.,1.));
#31329=DIRECTION('',(0.,0.,1.));
#31330=DIRECTION('center_axis',(0.707951511576272,-0.706261040449544,0.));
#31331=DIRECTION('ref_axis',(0.706261040449544,0.707951511576272,0.));
#31332=DIRECTION('',(0.,0.,-1.));
#31333=DIRECTION('center_axis',(0.,0.,1.));
#31334=DIRECTION('ref_axis',(-0.939692620785909,-0.342020143325669,0.));
#31335=DIRECTION('center_axis',(0.,0.,-1.));
#31336=DIRECTION('ref_axis',(1.,0.,0.));
#31337=DIRECTION('',(0.818465838146947,0.574555194725811,0.));
#31338=DIRECTION('',(-0.996298167445974,-0.0859648855277162,0.));
#31339=DIRECTION('center_axis',(-0.0859648855277162,0.996298167445974,0.));
#31340=DIRECTION('ref_axis',(-0.996298167445974,-0.0859648855277162,0.));
#31341=DIRECTION('',(0.,0.,1.));
#31342=DIRECTION('',(0.,0.,1.));
#31343=DIRECTION('center_axis',(0.574555194725811,-0.818465838146948,0.));
#31344=DIRECTION('ref_axis',(0.818465838146947,0.574555194725811,0.));
#31345=DIRECTION('',(0.,0.,-1.));
#31346=DIRECTION('center_axis',(0.,0.,1.));
#31347=DIRECTION('ref_axis',(-0.984807753012208,-0.17364817766693,0.));
#31348=DIRECTION('center_axis',(0.,0.,-1.));
#31349=DIRECTION('ref_axis',(1.,0.,0.));
#31350=DIRECTION('',(0.905801965515954,0.423701309022563,0.));
#31351=DIRECTION('',(-0.996089805327885,0.0883464754353941,0.));
#31352=DIRECTION('center_axis',(0.0883464754353941,0.996089805327885,0.));
#31353=DIRECTION('ref_axis',(-0.996089805327885,0.0883464754353941,0.));
#31354=DIRECTION('',(0.,0.,1.));
#31355=DIRECTION('',(0.,0.,1.));
#31356=DIRECTION('center_axis',(0.423701309022563,-0.905801965515954,0.));
#31357=DIRECTION('ref_axis',(0.905801965515954,0.423701309022563,0.));
#31358=DIRECTION('',(0.,0.,-1.));
#31359=DIRECTION('center_axis',(0.,0.,1.));
#31360=DIRECTION('ref_axis',(-1.,1.11022302462516E-16,0.));
#31361=DIRECTION('center_axis',(0.,0.,-1.));
#31362=DIRECTION('ref_axis',(1.,0.,0.));
#31363=DIRECTION('',(0.96561575852067,0.259973473447873,0.));
#31364=DIRECTION('',(-0.96561575852067,0.259973473447873,0.));
#31365=DIRECTION('center_axis',(0.,0.,-1.));
#31366=DIRECTION('ref_axis',(1.,0.,0.));
#31367=DIRECTION('center_axis',(0.259973473447873,0.96561575852067,0.));
#31368=DIRECTION('ref_axis',(-0.96561575852067,0.259973473447873,0.));
#31369=DIRECTION('',(0.,0.,1.));
#31370=DIRECTION('',(0.,0.,1.));
#31371=DIRECTION('center_axis',(0.259973473447873,-0.96561575852067,0.));
#31372=DIRECTION('ref_axis',(0.96561575852067,0.259973473447873,0.));
#31373=DIRECTION('',(0.,0.,-1.));
#31374=DIRECTION('center_axis',(0.,0.,1.));
#31375=DIRECTION('ref_axis',(-0.984807753012208,0.173648177666931,0.));
#31376=DIRECTION('center_axis',(0.,0.,-1.));
#31377=DIRECTION('ref_axis',(1.,0.,0.));
#31378=DIRECTION('',(0.996089805327885,0.0883464754353933,0.));
#31379=DIRECTION('',(-0.905801965515954,0.423701309022564,0.));
#31380=DIRECTION('center_axis',(0.423701309022564,0.905801965515954,0.));
#31381=DIRECTION('ref_axis',(-0.905801965515954,0.423701309022564,0.));
#31382=DIRECTION('',(0.,0.,1.));
#31383=DIRECTION('',(0.,0.,1.));
#31384=DIRECTION('center_axis',(0.0883464754353933,-0.996089805327885,0.));
#31385=DIRECTION('ref_axis',(0.996089805327885,0.0883464754353933,0.));
#31386=DIRECTION('',(0.,0.,-1.));
#31387=DIRECTION('center_axis',(0.,0.,1.));
#31388=DIRECTION('ref_axis',(-0.939692620785908,0.342020143325669,0.));
#31389=DIRECTION('center_axis',(0.,0.,-1.));
#31390=DIRECTION('ref_axis',(1.,0.,0.));
#31391=DIRECTION('',(0.996298167445974,-0.0859648855277165,0.));
#31392=DIRECTION('',(-0.818465838146947,0.574555194725811,0.));
#31393=DIRECTION('center_axis',(0.574555194725811,0.818465838146947,0.));
#31394=DIRECTION('ref_axis',(-0.818465838146947,0.574555194725811,0.));
#31395=DIRECTION('',(0.,0.,1.));
#31396=DIRECTION('',(0.,0.,1.));
#31397=DIRECTION('center_axis',(-0.0859648855277165,-0.996298167445974,
0.));
#31398=DIRECTION('ref_axis',(0.996298167445974,-0.0859648855277165,0.));
#31399=DIRECTION('',(0.,0.,-1.));
#31400=DIRECTION('center_axis',(0.,0.,1.));
#31401=DIRECTION('ref_axis',(-0.866025403784439,0.5,0.));
#31402=DIRECTION('center_axis',(0.,0.,-1.));
#31403=DIRECTION('ref_axis',(1.,0.,0.));
#31404=DIRECTION('',(0.966234513897416,-0.257664246944398,0.));
#31405=DIRECTION('',(-0.706261040449544,0.707951511576272,0.));
#31406=DIRECTION('center_axis',(0.707951511576272,0.706261040449544,0.));
#31407=DIRECTION('ref_axis',(-0.706261040449544,0.707951511576272,0.));
#31408=DIRECTION('',(0.,0.,1.));
#31409=DIRECTION('',(0.,0.,1.));
#31410=DIRECTION('center_axis',(-0.257664246944398,-0.966234513897416,0.));
#31411=DIRECTION('ref_axis',(0.966234513897416,-0.257664246944398,0.));
#31412=DIRECTION('',(0.,0.,-1.));
#31413=DIRECTION('center_axis',(0.,0.,1.));
#31414=DIRECTION('ref_axis',(-0.766044443118978,0.642787609686539,0.));
#31415=DIRECTION('center_axis',(0.,0.,-1.));
#31416=DIRECTION('ref_axis',(1.,0.,0.));
#31417=DIRECTION('',(0.906812313582341,-0.421534610602074,0.));
#31418=DIRECTION('',(-0.57259685842341,0.819837079988238,0.));
#31419=DIRECTION('center_axis',(0.819837079988238,0.572596858423411,0.));
#31420=DIRECTION('ref_axis',(-0.57259685842341,0.819837079988238,0.));
#31421=DIRECTION('',(0.,0.,1.));
#31422=DIRECTION('',(0.,0.,1.));
#31423=DIRECTION('center_axis',(-0.421534610602074,-0.906812313582341,0.));
#31424=DIRECTION('ref_axis',(0.906812313582341,-0.421534610602074,0.));
#31425=DIRECTION('',(0.,0.,-1.));
#31426=DIRECTION('center_axis',(0.,0.,1.));
#31427=DIRECTION('ref_axis',(-0.642787609686539,0.766044443118978,0.));
#31428=DIRECTION('center_axis',(0.,0.,-1.));
#31429=DIRECTION('ref_axis',(1.,0.,0.));
#31430=DIRECTION('',(0.819837079988238,-0.572596858423411,0.));
#31431=DIRECTION('',(-0.421534610602074,0.906812313582341,0.));
#31432=DIRECTION('center_axis',(0.906812313582341,0.421534610602074,0.));
#31433=DIRECTION('ref_axis',(-0.421534610602074,0.906812313582341,0.));
#31434=DIRECTION('',(0.,0.,1.));
#31435=DIRECTION('',(0.,0.,1.));
#31436=DIRECTION('center_axis',(-0.572596858423411,-0.819837079988238,0.));
#31437=DIRECTION('ref_axis',(0.819837079988238,-0.572596858423411,0.));
#31438=DIRECTION('',(0.,0.,-1.));
#31439=DIRECTION('center_axis',(0.,0.,1.));
#31440=DIRECTION('ref_axis',(-0.5,0.866025403784439,0.));
#31441=DIRECTION('center_axis',(0.,0.,-1.));
#31442=DIRECTION('ref_axis',(1.,0.,0.));
#31443=DIRECTION('',(0.707951511576272,-0.706261040449544,0.));
#31444=DIRECTION('',(-0.257664246944397,0.966234513897416,0.));
#31445=DIRECTION('center_axis',(0.966234513897416,0.257664246944397,0.));
#31446=DIRECTION('ref_axis',(-0.257664246944397,0.966234513897416,0.));
#31447=DIRECTION('',(0.,0.,1.));
#31448=DIRECTION('',(0.,0.,1.));
#31449=DIRECTION('center_axis',(-0.706261040449544,-0.707951511576272,0.));
#31450=DIRECTION('ref_axis',(0.707951511576272,-0.706261040449544,0.));
#31451=DIRECTION('',(0.,0.,-1.));
#31452=DIRECTION('center_axis',(0.,0.,1.));
#31453=DIRECTION('ref_axis',(-0.342020143325669,0.939692620785909,0.));
#31454=DIRECTION('center_axis',(0.,0.,-1.));
#31455=DIRECTION('ref_axis',(1.,0.,0.));
#31456=DIRECTION('',(0.574555194725811,-0.818465838146947,0.));
#31457=DIRECTION('',(-0.0859648855277162,0.996298167445974,0.));
#31458=DIRECTION('center_axis',(0.996298167445974,0.0859648855277162,0.));
#31459=DIRECTION('ref_axis',(-0.0859648855277162,0.996298167445974,0.));
#31460=DIRECTION('',(0.,0.,1.));
#31461=DIRECTION('',(0.,0.,1.));
#31462=DIRECTION('center_axis',(-0.818465838146948,-0.574555194725811,0.));
#31463=DIRECTION('ref_axis',(0.574555194725811,-0.818465838146947,0.));
#31464=DIRECTION('',(0.,0.,-1.));
#31465=DIRECTION('center_axis',(0.,0.,1.));
#31466=DIRECTION('ref_axis',(-0.17364817766693,0.984807753012208,0.));
#31467=DIRECTION('center_axis',(0.,0.,-1.));
#31468=DIRECTION('ref_axis',(1.,0.,0.));
#31469=DIRECTION('',(0.423701309022564,-0.905801965515954,0.));
#31470=DIRECTION('',(0.0883464754353937,0.996089805327885,0.));
#31471=DIRECTION('center_axis',(0.996089805327885,-0.0883464754353937,0.));
#31472=DIRECTION('ref_axis',(0.0883464754353937,0.996089805327885,0.));
#31473=DIRECTION('',(0.,0.,1.));
#31474=DIRECTION('',(0.,0.,1.));
#31475=DIRECTION('center_axis',(-0.905801965515954,-0.423701309022564,0.));
#31476=DIRECTION('ref_axis',(0.423701309022564,-0.905801965515954,0.));
#31477=DIRECTION('',(0.,0.,-1.));
#31478=DIRECTION('center_axis',(0.,0.,1.));
#31479=DIRECTION('ref_axis',(5.55111512312578E-17,1.,0.));
#31480=DIRECTION('center_axis',(0.,0.,-1.));
#31481=DIRECTION('ref_axis',(1.,0.,0.));
#31482=DIRECTION('',(0.259973473447873,-0.96561575852067,0.));
#31483=DIRECTION('',(0.259973473447873,0.96561575852067,0.));
#31484=DIRECTION('center_axis',(0.96561575852067,-0.259973473447873,0.));
#31485=DIRECTION('ref_axis',(0.259973473447873,0.96561575852067,0.));
#31486=DIRECTION('',(0.,0.,1.));
#31487=DIRECTION('',(0.,0.,1.));
#31488=DIRECTION('center_axis',(-0.96561575852067,-0.259973473447873,0.));
#31489=DIRECTION('ref_axis',(0.259973473447873,-0.96561575852067,0.));
#31490=DIRECTION('',(0.,0.,-1.));
#31491=DIRECTION('center_axis',(0.,0.,1.));
#31492=DIRECTION('ref_axis',(0.17364817766693,0.984807753012208,0.));
#31493=DIRECTION('center_axis',(0.,0.,-1.));
#31494=DIRECTION('ref_axis',(1.,0.,0.));
#31495=DIRECTION('',(0.0883464754353936,-0.996089805327885,0.));
#31496=DIRECTION('',(0.423701309022564,0.905801965515954,0.));
#31497=DIRECTION('center_axis',(0.905801965515954,-0.423701309022564,0.));
#31498=DIRECTION('ref_axis',(0.423701309022564,0.905801965515954,0.));
#31499=DIRECTION('',(0.,0.,1.));
#31500=DIRECTION('',(0.,0.,1.));
#31501=DIRECTION('center_axis',(-0.996089805327885,-0.0883464754353936,
0.));
#31502=DIRECTION('ref_axis',(0.0883464754353936,-0.996089805327885,0.));
#31503=DIRECTION('',(0.,0.,-1.));
#31504=DIRECTION('center_axis',(0.,0.,1.));
#31505=DIRECTION('ref_axis',(0.342020143325669,0.939692620785908,0.));
#31506=DIRECTION('center_axis',(0.,0.,-1.));
#31507=DIRECTION('ref_axis',(1.,0.,0.));
#31508=DIRECTION('',(-0.0859648855277165,-0.996298167445974,0.));
#31509=DIRECTION('',(0.574555194725811,0.818465838146947,0.));
#31510=DIRECTION('center_axis',(0.818465838146947,-0.574555194725811,0.));
#31511=DIRECTION('ref_axis',(0.574555194725811,0.818465838146947,0.));
#31512=DIRECTION('',(0.,0.,1.));
#31513=DIRECTION('',(0.,0.,1.));
#31514=DIRECTION('center_axis',(-0.996298167445974,0.0859648855277165,0.));
#31515=DIRECTION('ref_axis',(-0.0859648855277165,-0.996298167445974,0.));
#31516=DIRECTION('',(0.,0.,-1.));
#31517=DIRECTION('center_axis',(0.,0.,1.));
#31518=DIRECTION('ref_axis',(0.5,0.866025403784439,0.));
#31519=DIRECTION('center_axis',(0.,0.,-1.));
#31520=DIRECTION('ref_axis',(1.,0.,0.));
#31521=DIRECTION('',(-0.257664246944398,-0.966234513897416,0.));
#31522=DIRECTION('',(0.707951511576272,0.706261040449543,0.));
#31523=DIRECTION('center_axis',(0.706261040449544,-0.707951511576272,0.));
#31524=DIRECTION('ref_axis',(0.707951511576272,0.706261040449543,0.));
#31525=DIRECTION('',(0.,0.,1.));
#31526=DIRECTION('',(0.,0.,1.));
#31527=DIRECTION('center_axis',(-0.966234513897416,0.257664246944398,0.));
#31528=DIRECTION('ref_axis',(-0.257664246944398,-0.966234513897416,0.));
#31529=DIRECTION('',(0.,0.,-1.));
#31530=DIRECTION('center_axis',(0.,0.,1.));
#31531=DIRECTION('ref_axis',(0.642787609686539,0.766044443118978,0.));
#31532=DIRECTION('center_axis',(0.,0.,-1.));
#31533=DIRECTION('ref_axis',(1.,0.,0.));
#31534=DIRECTION('',(-0.421534610602074,-0.906812313582341,0.));
#31535=DIRECTION('',(0.819837079988238,0.572596858423411,0.));
#31536=DIRECTION('center_axis',(0.572596858423411,-0.819837079988238,0.));
#31537=DIRECTION('ref_axis',(0.819837079988238,0.572596858423411,0.));
#31538=DIRECTION('',(0.,0.,1.));
#31539=DIRECTION('',(0.,0.,1.));
#31540=DIRECTION('center_axis',(-0.906812313582341,0.421534610602074,0.));
#31541=DIRECTION('ref_axis',(-0.421534610602074,-0.906812313582341,0.));
#31542=DIRECTION('',(0.,0.,-1.));
#31543=DIRECTION('center_axis',(0.,0.,1.));
#31544=DIRECTION('ref_axis',(0.766044443118978,0.642787609686539,0.));
#31545=DIRECTION('center_axis',(0.,0.,-1.));
#31546=DIRECTION('ref_axis',(1.,0.,0.));
#31547=DIRECTION('',(-0.572596858423411,-0.819837079988238,0.));
#31548=DIRECTION('',(0.906812313582341,0.421534610602073,0.));
#31549=DIRECTION('center_axis',(0.421534610602074,-0.906812313582341,0.));
#31550=DIRECTION('ref_axis',(0.906812313582341,0.421534610602073,0.));
#31551=DIRECTION('',(0.,0.,1.));
#31552=DIRECTION('',(0.,0.,1.));
#31553=DIRECTION('center_axis',(-0.819837079988238,0.572596858423411,0.));
#31554=DIRECTION('ref_axis',(-0.572596858423411,-0.819837079988238,0.));
#31555=DIRECTION('',(0.,0.,-1.));
#31556=DIRECTION('center_axis',(0.,0.,1.));
#31557=DIRECTION('ref_axis',(0.866025403784439,0.5,0.));
#31558=DIRECTION('center_axis',(0.,0.,-1.));
#31559=DIRECTION('ref_axis',(1.,0.,0.));
#31560=DIRECTION('',(-0.706261040449544,-0.707951511576272,0.));
#31561=DIRECTION('',(0.966234513897416,0.257664246944398,0.));
#31562=DIRECTION('center_axis',(0.257664246944398,-0.966234513897416,0.));
#31563=DIRECTION('ref_axis',(0.966234513897416,0.257664246944398,0.));
#31564=DIRECTION('',(0.,0.,1.));
#31565=DIRECTION('',(0.,0.,1.));
#31566=DIRECTION('center_axis',(-0.707951511576272,0.706261040449544,0.));
#31567=DIRECTION('ref_axis',(-0.706261040449544,-0.707951511576272,0.));
#31568=DIRECTION('',(0.,0.,-1.));
#31569=DIRECTION('center_axis',(0.,0.,1.));
#31570=DIRECTION('ref_axis',(0.939692620785909,0.342020143325669,0.));
#31571=DIRECTION('center_axis',(0.,0.,-1.));
#31572=DIRECTION('ref_axis',(1.,0.,0.));
#31573=DIRECTION('',(-0.818465838146947,-0.574555194725811,0.));
#31574=DIRECTION('',(0.996298167445974,0.0859648855277162,0.));
#31575=DIRECTION('center_axis',(0.0859648855277162,-0.996298167445974,0.));
#31576=DIRECTION('ref_axis',(0.996298167445974,0.0859648855277162,0.));
#31577=DIRECTION('',(0.,0.,1.));
#31578=DIRECTION('',(0.,0.,1.));
#31579=DIRECTION('center_axis',(-0.574555194725811,0.818465838146948,0.));
#31580=DIRECTION('ref_axis',(-0.818465838146947,-0.574555194725811,0.));
#31581=DIRECTION('',(0.,0.,-1.));
#31582=DIRECTION('center_axis',(0.,0.,1.));
#31583=DIRECTION('ref_axis',(0.984807753012208,0.17364817766693,0.));
#31584=DIRECTION('center_axis',(0.,0.,-1.));
#31585=DIRECTION('ref_axis',(1.,0.,0.));
#31586=DIRECTION('',(-0.905801965515954,-0.423701309022564,0.));
#31587=DIRECTION('',(0.996089805327885,-0.0883464754353937,0.));
#31588=DIRECTION('center_axis',(-0.0883464754353937,-0.996089805327885,
0.));
#31589=DIRECTION('ref_axis',(0.996089805327885,-0.0883464754353937,0.));
#31590=DIRECTION('',(0.,0.,1.));
#31591=DIRECTION('',(0.,0.,1.));
#31592=DIRECTION('center_axis',(-0.423701309022564,0.905801965515954,0.));
#31593=DIRECTION('ref_axis',(-0.905801965515954,-0.423701309022564,0.));
#31594=DIRECTION('',(0.,0.,-1.));
#31595=DIRECTION('center_axis',(0.,0.,1.));
#31596=DIRECTION('ref_axis',(1.,0.,0.));
#31597=DIRECTION('center_axis',(0.,0.,1.));
#31598=DIRECTION('ref_axis',(1.,0.,0.));
#31599=DIRECTION('center_axis',(0.,0.,1.));
#31600=DIRECTION('ref_axis',(1.,0.,0.));
#31601=DIRECTION('center_axis',(0.,0.,1.));
#31602=DIRECTION('ref_axis',(1.,0.,0.));
#31603=DIRECTION('center_axis',(0.,0.,1.));
#31604=DIRECTION('ref_axis',(1.,0.,0.));
#31605=DIRECTION('center_axis',(0.,0.,1.));
#31606=DIRECTION('ref_axis',(1.,0.,0.));
#31607=DIRECTION('center_axis',(0.,0.,1.));
#31608=DIRECTION('ref_axis',(1.,0.,0.));
#31609=DIRECTION('center_axis',(0.,0.,1.));
#31610=DIRECTION('ref_axis',(1.,0.,0.));
#31611=DIRECTION('center_axis',(0.,0.,1.));
#31612=DIRECTION('ref_axis',(1.,0.,0.));
#31613=DIRECTION('center_axis',(0.,0.,1.));
#31614=DIRECTION('ref_axis',(1.,0.,0.));
#31615=DIRECTION('center_axis',(0.,0.,1.));
#31616=DIRECTION('ref_axis',(1.,0.,0.));
#31617=DIRECTION('center_axis',(0.,0.,1.));
#31618=DIRECTION('ref_axis',(1.,0.,0.));
#31619=DIRECTION('center_axis',(0.,0.,1.));
#31620=DIRECTION('ref_axis',(1.,0.,0.));
#31621=DIRECTION('center_axis',(0.,0.,1.));
#31622=DIRECTION('ref_axis',(1.,0.,0.));
#31623=DIRECTION('center_axis',(0.,0.,1.));
#31624=DIRECTION('ref_axis',(1.,0.,0.));
#31625=DIRECTION('center_axis',(0.,0.,1.));
#31626=DIRECTION('ref_axis',(1.,0.,0.));
#31627=DIRECTION('center_axis',(0.,0.,1.));
#31628=DIRECTION('ref_axis',(1.,0.,0.));
#31629=DIRECTION('center_axis',(0.,0.,1.));
#31630=DIRECTION('ref_axis',(1.,0.,0.));
#31631=DIRECTION('',(0.,0.,-1.));
#31632=DIRECTION('center_axis',(0.,0.,1.));
#31633=DIRECTION('ref_axis',(1.,0.,0.));
#31634=DIRECTION('center_axis',(0.,0.,1.));
#31635=DIRECTION('ref_axis',(1.,0.,0.));
#31636=DIRECTION('center_axis',(0.,0.,1.));
#31637=DIRECTION('ref_axis',(1.,0.,0.));
#31638=DIRECTION('center_axis',(0.,0.,1.));
#31639=DIRECTION('ref_axis',(1.,0.,0.));
#31640=DIRECTION('center_axis',(0.,0.,1.));
#31641=DIRECTION('ref_axis',(1.,0.,0.));
#31642=DIRECTION('center_axis',(0.,0.,1.));
#31643=DIRECTION('ref_axis',(1.,0.,0.));
#31644=DIRECTION('center_axis',(0.,0.,1.));
#31645=DIRECTION('ref_axis',(1.,0.,0.));
#31646=DIRECTION('center_axis',(0.,0.,1.));
#31647=DIRECTION('ref_axis',(1.,0.,0.));
#31648=DIRECTION('center_axis',(0.,0.,1.));
#31649=DIRECTION('ref_axis',(1.,0.,0.));
#31650=DIRECTION('center_axis',(0.,0.,1.));
#31651=DIRECTION('ref_axis',(1.,0.,0.));
#31652=DIRECTION('center_axis',(0.,0.,1.));
#31653=DIRECTION('ref_axis',(1.,0.,0.));
#31654=DIRECTION('center_axis',(0.,0.,1.));
#31655=DIRECTION('ref_axis',(1.,0.,0.));
#31656=DIRECTION('center_axis',(0.,0.,1.));
#31657=DIRECTION('ref_axis',(1.,0.,0.));
#31658=DIRECTION('center_axis',(0.,0.,1.));
#31659=DIRECTION('ref_axis',(1.,0.,0.));
#31660=DIRECTION('center_axis',(0.,0.,1.));
#31661=DIRECTION('ref_axis',(1.,0.,0.));
#31662=DIRECTION('center_axis',(0.,0.,1.));
#31663=DIRECTION('ref_axis',(1.,0.,0.));
#31664=DIRECTION('center_axis',(0.,0.,1.));
#31665=DIRECTION('ref_axis',(1.,0.,0.));
#31666=DIRECTION('center_axis',(0.,0.,1.));
#31667=DIRECTION('ref_axis',(1.,0.,0.));
#31668=DIRECTION('center_axis',(0.,0.,1.));
#31669=DIRECTION('ref_axis',(1.,0.,0.));
#31670=DIRECTION('',(0.,0.,-1.));
#31671=DIRECTION('center_axis',(0.,0.,-1.));
#31672=DIRECTION('ref_axis',(1.,0.,0.));
#31673=DIRECTION('',(0.,0.,1.));
#31674=DIRECTION('center_axis',(0.,0.,1.));
#31675=DIRECTION('ref_axis',(1.,0.,0.));
#31676=DIRECTION('center_axis',(-0.259973473447873,-0.96561575852067,0.));
#31677=DIRECTION('ref_axis',(0.96561575852067,-0.259973473447873,0.));
#31678=DIRECTION('',(0.96561575852067,-0.259973473447873,0.));
#31679=DIRECTION('',(0.,0.,1.));
#31680=DIRECTION('center_axis',(-0.259973473447873,0.96561575852067,0.));
#31681=DIRECTION('ref_axis',(-0.96561575852067,-0.259973473447873,0.));
#31682=DIRECTION('',(-0.96561575852067,-0.259973473447873,0.));
#31683=DIRECTION('center_axis',(0.,0.,1.));
#31684=DIRECTION('ref_axis',(1.,0.,0.));
#31685=DIRECTION('center_axis',(0.,0.,-1.));
#31686=DIRECTION('ref_axis',(1.,0.,0.));
#31687=DIRECTION('center_axis',(0.,0.,1.));
#31688=DIRECTION('ref_axis',(1.,0.,0.));
#31689=DIRECTION('',(-0.707106781186548,-8.65956056235493E-17,-0.707106781186548));
#31690=DIRECTION('center_axis',(0.,0.,1.));
#31691=DIRECTION('ref_axis',(1.,0.,0.));
#31692=DIRECTION('',(-0.845934045579678,-1.03597042120892E-16,0.533287530821037));
#31693=DIRECTION('center_axis',(0.,0.,-1.));
#31694=DIRECTION('ref_axis',(1.,0.,0.));
#31695=DIRECTION('center_axis',(0.5,0.866025403784439,0.));
#31696=DIRECTION('ref_axis',(0.866025403784439,-0.5,0.));
#31697=DIRECTION('',(0.866025403784439,-0.5,0.));
#31698=DIRECTION('',(0.,0.,-1.));
#31699=DIRECTION('',(0.866025403784439,-0.5,0.));
#31700=DIRECTION('',(0.,0.,-1.));
#31701=DIRECTION('center_axis',(-0.5,0.866025403784439,0.));
#31702=DIRECTION('ref_axis',(0.866025403784439,0.5,0.));
#31703=DIRECTION('',(0.866025403784439,0.5,0.));
#31704=DIRECTION('',(0.,0.,-1.));
#31705=DIRECTION('',(0.866025403784439,0.5,0.));
#31706=DIRECTION('center_axis',(-1.,-1.20185167898973E-16,0.));
#31707=DIRECTION('ref_axis',(-1.20185167898973E-16,1.,0.));
#31708=DIRECTION('',(-1.20185167898973E-16,1.,0.));
#31709=DIRECTION('',(0.,0.,-1.));
#31710=DIRECTION('',(-1.20185167898973E-16,1.,0.));
#31711=DIRECTION('center_axis',(-0.5,-0.866025403784439,0.));
#31712=DIRECTION('ref_axis',(-0.866025403784439,0.5,0.));
#31713=DIRECTION('',(-0.866025403784439,0.5,0.));
#31714=DIRECTION('',(0.,0.,-1.));
#31715=DIRECTION('',(-0.866025403784439,0.5,0.));
#31716=DIRECTION('center_axis',(0.5,-0.866025403784439,0.));
#31717=DIRECTION('ref_axis',(-0.866025403784439,-0.5,0.));
#31718=DIRECTION('',(-0.866025403784439,-0.5,0.));
#31719=DIRECTION('',(0.,0.,-1.));
#31720=DIRECTION('',(-0.866025403784439,-0.5,0.));
#31721=DIRECTION('center_axis',(1.,-3.60555503696918E-16,0.));
#31722=DIRECTION('ref_axis',(-3.60555503696918E-16,-1.,0.));
#31723=DIRECTION('',(-3.60555503696918E-16,-1.,0.));
#31724=DIRECTION('',(-3.60555503696918E-16,-1.,0.));
#31725=DIRECTION('center_axis',(0.,0.,-1.));
#31726=DIRECTION('ref_axis',(-1.,0.,0.));
#31727=DIRECTION('center_axis',(0.,0.,-1.));
#31728=DIRECTION('ref_axis',(-1.,0.,0.));
#31729=DIRECTION('center_axis',(0.,0.,1.));
#31730=DIRECTION('ref_axis',(1.,0.,0.));
#31731=DIRECTION('center_axis',(0.,0.,1.));
#31732=DIRECTION('ref_axis',(1.,0.,0.));
#31733=DIRECTION('',(0.707106781186547,8.65956056235493E-17,-0.707106781186548));
#31734=DIRECTION('center_axis',(0.,0.,1.));
#31735=DIRECTION('ref_axis',(1.,0.,0.));
#31736=DIRECTION('center_axis',(0.,0.,1.));
#31737=DIRECTION('ref_axis',(1.,0.,0.));
#31738=DIRECTION('center_axis',(0.,0.,1.));
#31739=DIRECTION('ref_axis',(1.,0.,0.));
#31740=DIRECTION('center_axis',(0.,0.,1.));
#31741=DIRECTION('ref_axis',(1.,0.,0.));
#31742=DIRECTION('',(0.707106781186548,8.65956056235494E-17,-0.707106781186547));
#31743=DIRECTION('center_axis',(0.,0.,-1.));
#31744=DIRECTION('ref_axis',(-1.,0.,0.));
#31745=DIRECTION('center_axis',(0.,0.,1.));
#31746=DIRECTION('ref_axis',(1.,0.,0.));
#50089=CARTESIAN_POINT('',(0.,0.,0.));
#50090=CARTESIAN_POINT('Origin',(0.,0.,-0.775));
#50091=CARTESIAN_POINT('',(-0.245447138551752,4.00299569890614E-5,-1.43916725037879));
#50092=CARTESIAN_POINT('',(-0.245435809527805,6.93114097173611E-5,-1.45073274962121));
#50093=CARTESIAN_POINT('',(-0.24505,-3.00099698131059E-17,-0.775));
#50094=CARTESIAN_POINT('',(-0.232143106254475,-0.0797426101647723,-1.51495));
#50095=CARTESIAN_POINT('Ctrl Pts',(-0.245447138551752,4.00299569890614E-5,
-1.43916725037879));
#50096=CARTESIAN_POINT('Ctrl Pts',(-0.245452129536357,0.0022198044307001,
-1.43928101890267));
#50097=CARTESIAN_POINT('Ctrl Pts',(-0.245425591838023,0.00439945516314897,
-1.43939478742655));
#50098=CARTESIAN_POINT('Ctrl Pts',(-0.24536715191998,0.00657825184837683,
-1.43950855595043));
#50099=CARTESIAN_POINT('Ctrl Pts',(-0.243189299218486,0.0877744342843084,
-1.44374831355743));
#50100=CARTESIAN_POINT('Ctrl Pts',(-0.196705837434329,0.167784521123834,
-1.44798807116442));
#50101=CARTESIAN_POINT('Ctrl Pts',(-0.127250682360293,0.209893324947318,
-1.45222782877142));
#50102=CARTESIAN_POINT('Ctrl Pts',(-0.0577955272862565,0.252002128770801,
-1.45646758637841));
#50103=CARTESIAN_POINT('Ctrl Pts',(0.0346313210776596,0.25620964957824,
-1.46070734398541));
#50104=CARTESIAN_POINT('Ctrl Pts',(0.10763278442824,0.220593165770989,-1.4649471015924));
#50105=CARTESIAN_POINT('Ctrl Pts',(0.18063424777882,0.184976681963739,-1.4691868591994));
#50106=CARTESIAN_POINT('Ctrl Pts',(0.234210326116065,0.109536193541798,
-1.47342661680639));
#50107=CARTESIAN_POINT('Ctrl Pts',(0.243757317623978,0.0288712065516735,
-1.47766637441339));
#50108=CARTESIAN_POINT('Ctrl Pts',(0.253304309131892,-0.0517937804384507,
-1.48190613202038));
#50109=CARTESIAN_POINT('Ctrl Pts',(0.218822213810474,-0.137683265996759,
-1.48614588962738));
#50110=CARTESIAN_POINT('Ctrl Pts',(0.156173226820107,-0.189360044779689,
-1.49038564723437));
#50111=CARTESIAN_POINT('Ctrl Pts',(0.0935242398297384,-0.241036823562619,
-1.49462540484137));
#50112=CARTESIAN_POINT('Ctrl Pts',(0.00270836117041977,-0.258500895570172,
-1.49886516244836));
#50113=CARTESIAN_POINT('Ctrl Pts',(-0.074683455425355,-0.233793976655611,
-1.50310492005536));
#50114=CARTESIAN_POINT('Ctrl Pts',(-0.146756149166573,-0.210785158946641,
-1.50705328003691));
#50115=CARTESIAN_POINT('Ctrl Pts',(-0.20718663426269,-0.151202949907839,
-1.51100164001845));
#50116=CARTESIAN_POINT('Ctrl Pts',(-0.232146081401957,-0.0797429895224405,
-1.51495));
#50117=CARTESIAN_POINT('',(-0.24505,-3.00099698131059E-17,-1.51495));
#50118=CARTESIAN_POINT('Origin',(0.,0.,-1.51495));
#50119=CARTESIAN_POINT('',(-0.24505,-3.00099698131059E-17,-1.54495));
#50120=CARTESIAN_POINT('',(-0.24505,-3.00099698131059E-17,-0.775));
#50121=CARTESIAN_POINT('Origin',(0.,0.,-1.54495));
#50122=CARTESIAN_POINT('',(-0.0796899944392842,-0.231730462577251,-1.51495));
#50123=CARTESIAN_POINT('Origin',(0.,0.,-1.51495));
#50124=CARTESIAN_POINT('Ctrl Pts',(-0.079689994439284,-0.231730462577251,
-1.51495));
#50125=CARTESIAN_POINT('Ctrl Pts',(-0.00252611781080675,-0.258266416594893,
-1.510710242393));
#50126=CARTESIAN_POINT('Ctrl Pts',(0.0882646015602411,-0.242994367587768,
-1.50647048478601));
#50127=CARTESIAN_POINT('Ctrl Pts',(0.151921953058853,-0.192764344174053,
-1.50223072717901));
#50128=CARTESIAN_POINT('Ctrl Pts',(0.215579304557466,-0.142534320760337,
-1.49799096957202));
#50129=CARTESIAN_POINT('Ctrl Pts',(0.252103288183642,-0.0573463229400297,
-1.49375121196502));
#50130=CARTESIAN_POINT('Ctrl Pts',(0.24437106297374,0.0235286269972124,
-1.48951145435803));
#50131=CARTESIAN_POINT('Ctrl Pts',(0.236638837763837,0.104403576934455,
-1.48527169675103));
#50132=CARTESIAN_POINT('Ctrl Pts',(0.184650403717856,0.180965478988632,
-1.48103193914404));
#50133=CARTESIAN_POINT('Ctrl Pts',(0.112428881394831,0.218167306952772,
-1.47679218153704));
#50134=CARTESIAN_POINT('Ctrl Pts',(0.0402073590718059,0.255369134916912,
-1.47255242393005));
#50135=CARTESIAN_POINT('Ctrl Pts',(-0.052247251528263,0.253210888791013,
-1.46831266632305));
#50136=CARTESIAN_POINT('Ctrl Pts',(-0.122600130208318,0.212641738373403,
-1.46407290871606));
#50137=CARTESIAN_POINT('Ctrl Pts',(-0.192953008888373,0.172072587955792,
-1.45983315110906));
#50138=CARTESIAN_POINT('Ctrl Pts',(-0.241204155648414,0.0930925332464675,
-1.45559339350207));
#50139=CARTESIAN_POINT('Ctrl Pts',(-0.245169531263596,0.0119613979719827,
-1.45135363589507));
#50140=CARTESIAN_POINT('Ctrl Pts',(-0.245363099506438,0.00800101368085023,
-1.45114667380378));
#50141=CARTESIAN_POINT('Ctrl Pts',(-0.245451140707558,0.00403550365378323,
-1.45093971171249));
#50142=CARTESIAN_POINT('Ctrl Pts',(-0.245435809527805,6.93114097173611E-5,
-1.45073274962121));
#50143=CARTESIAN_POINT('Origin',(0.,0.,-0.775));
#50144=CARTESIAN_POINT('',(-0.244854737116733,0.000201854273987251,-1.35916725037879));
#50145=CARTESIAN_POINT('',(-0.244810640388203,0.000186482913498504,-1.37073274962121));
#50146=CARTESIAN_POINT('',(-0.24505,-3.00099698131059E-17,-0.775));
#50147=CARTESIAN_POINT('Ctrl Pts',(-0.244854737116733,0.000201854273987251,
-1.35916725037879));
#50148=CARTESIAN_POINT('Ctrl Pts',(-0.245054986723865,0.0260726681896089,
-1.36050913992737));
#50149=CARTESIAN_POINT('Ctrl Pts',(-0.241281085006606,0.0518865600215586,
-1.36185102947594));
#50150=CARTESIAN_POINT('Ctrl Pts',(-0.233287666986612,0.0763200425298408,
-1.36319291902451));
#50151=CARTESIAN_POINT('Ctrl Pts',(-0.20803211976799,0.153518678915402,
-1.36743267663151));
#50152=CARTESIAN_POINT('Ctrl Pts',(-0.140654359094768,0.216937087423053,
-1.3716724342385));
#50153=CARTESIAN_POINT('Ctrl Pts',(-0.0620694940034391,0.237476868429796,
-1.3759121918455));
#50154=CARTESIAN_POINT('Ctrl Pts',(0.0165153710878895,0.25801664943654,
-1.3801519494525));
#50155=CARTESIAN_POINT('Ctrl Pts',(0.106307340597324,0.235677802942377,
-1.38439170705949));
#50156=CARTESIAN_POINT('Ctrl Pts',(0.166107334095492,0.180710241059491,
-1.38863146466649));
#50157=CARTESIAN_POINT('Ctrl Pts',(0.225907327593661,0.125742679176606,
-1.39287122227348));
#50158=CARTESIAN_POINT('Ctrl Pts',(0.255715345080564,0.0381464019049985,
-1.39711097988048));
#50159=CARTESIAN_POINT('Ctrl Pts',(0.241854107162481,-0.0418870385864429,
-1.40135073748747));
#50160=CARTESIAN_POINT('Ctrl Pts',(0.227992869244398,-0.121920479077884,
-1.40559049509447));
#50161=CARTESIAN_POINT('Ctrl Pts',(0.170462375921329,-0.19439108278916,
-1.40983025270146));
#50162=CARTESIAN_POINT('Ctrl Pts',(0.0956602335168951,-0.226046518003429,
-1.41407001030846));
#50163=CARTESIAN_POINT('Ctrl Pts',(0.020858091112461,-0.257701953217699,
-1.41830976791545));
#50164=CARTESIAN_POINT('Ctrl Pts',(-0.0712157003733378,-0.248542219934963,
-1.42254952552245));
#50165=CARTESIAN_POINT('Ctrl Pts',(-0.138316474306822,-0.202771214277427,
-1.42678928312944));
#50166=CARTESIAN_POINT('Ctrl Pts',(-0.203616683984248,-0.158228415567734,
-1.43091527221256));
#50167=CARTESIAN_POINT('Ctrl Pts',(-0.245266132880854,-0.0790128167847663,
-1.43504126129568));
#50168=CARTESIAN_POINT('Ctrl Pts',(-0.245447138551752,4.00299569890614E-5,
-1.43916725037879));
#50169=CARTESIAN_POINT('Ctrl Pts',(-0.245435809527805,6.93114097173611E-5,
-1.45073274962121));
#50170=CARTESIAN_POINT('Ctrl Pts',(-0.245137071181209,-0.0772146114419689,
-1.4466999541055));
#50171=CARTESIAN_POINT('Ctrl Pts',(-0.205588725723683,-0.154757566241512,
-1.44266715858979));
#50172=CARTESIAN_POINT('Ctrl Pts',(-0.142732123706006,-0.199683987839884,
-1.43863436307408));
#50173=CARTESIAN_POINT('Ctrl Pts',(-0.0766497360629118,-0.24691602253762,
-1.43439460546709));
#50174=CARTESIAN_POINT('Ctrl Pts',(0.0151946436936002,-0.258097876093446,
-1.43015484786009));
#50175=CARTESIAN_POINT('Ctrl Pts',(0.0906723427971956,-0.228093108159075,
-1.4259150902531));
#50176=CARTESIAN_POINT('Ctrl Pts',(0.166150041900791,-0.198088340224704,
-1.4216753326461));
#50177=CARTESIAN_POINT('Ctrl Pts',(0.22526106035147,-0.126896950800135,
-1.41743557503911));
#50178=CARTESIAN_POINT('Ctrl Pts',(0.240876966702014,-0.0471868123444759,
-1.41319581743211));
#50179=CARTESIAN_POINT('Ctrl Pts',(0.256492873052558,0.0325233261111841,
-1.40895605982512));
#50180=CARTESIAN_POINT('Ctrl Pts',(0.228613667302968,0.120752213597935,
-1.40471630221812));
#50181=CARTESIAN_POINT('Ctrl Pts',(0.17003458597265,0.177019340192329,-1.40047654461113));
#50182=CARTESIAN_POINT('Ctrl Pts',(0.111455504642331,0.233286466786723,
-1.39623678700413));
#50183=CARTESIAN_POINT('Ctrl Pts',(0.0221765477312852,0.25759183248876,
-1.39199702939714));
#50184=CARTESIAN_POINT('Ctrl Pts',(-0.0568401410365609,0.238782541867253,
-1.38775727179014));
#50185=CARTESIAN_POINT('Ctrl Pts',(-0.135856829804407,0.219973251245746,
-1.38351751418315));
#50186=CARTESIAN_POINT('Ctrl Pts',(-0.204611250429054,0.158049304300695,
-1.37927775657615));
#50187=CARTESIAN_POINT('Ctrl Pts',(-0.231555826218807,0.0814237546635944,
-1.37503799896915));
#50188=CARTESIAN_POINT('Ctrl Pts',(-0.240676089537489,0.0554873585932992,
-1.37360291585317));
#50189=CARTESIAN_POINT('Ctrl Pts',(-0.245006186352852,0.0278665954788627,
-1.37216783273719));
#50190=CARTESIAN_POINT('Ctrl Pts',(-0.244810640388203,0.000186482913498504,
-1.37073274962121));
#50191=CARTESIAN_POINT('Origin',(0.,0.,-0.775));
#50192=CARTESIAN_POINT('',(-0.244719259061378,-0.000134367261369422,-1.27916725037879));
#50193=CARTESIAN_POINT('',(-0.244751695427407,-0.000157197744526027,-1.29073274962121));
#50194=CARTESIAN_POINT('',(-0.24505,-3.00099698131059E-17,-0.775));
#50195=CARTESIAN_POINT('Ctrl Pts',(-0.244719259061378,-0.000134367261369422,
-1.27916725037879));
#50196=CARTESIAN_POINT('Ctrl Pts',(-0.244472862950292,0.0494828240606653,
-1.28173726095206));
#50197=CARTESIAN_POINT('Ctrl Pts',(-0.229836346380894,0.0992336302732099,
-1.28430727152533));
#50198=CARTESIAN_POINT('Ctrl Pts',(-0.201810743245362,0.139715073160739,
-1.2868772820986));
#50199=CARTESIAN_POINT('Ctrl Pts',(-0.155576784007822,0.206497485346041,
-1.29111703970559));
#50200=CARTESIAN_POINT('Ctrl Pts',(-0.0729040986815001,0.248053098858462,
-1.29535679731259));
#50201=CARTESIAN_POINT('Ctrl Pts',(0.00827454241877256,0.245314919832351,
-1.29959655491958));
#50202=CARTESIAN_POINT('Ctrl Pts',(0.0894531835190455,0.24257674080624,
-1.30383631252658));
#50203=CARTESIAN_POINT('Ctrl Pts',(0.16913778039327,0.195544769241596,-1.30807607013357));
#50204=CARTESIAN_POINT('Ctrl Pts',(0.210766596934376,0.125798721930996,
-1.31231582774057));
#50205=CARTESIAN_POINT('Ctrl Pts',(0.252395413475482,0.0560526746203967,
-1.31655558534757));
#50206=CARTESIAN_POINT('Ctrl Pts',(0.255968449683472,-0.0364074484361572,
-1.32079534295456));
#50207=CARTESIAN_POINT('Ctrl Pts',(0.219846277492275,-0.109158108861869,
-1.32503510056156));
#50208=CARTESIAN_POINT('Ctrl Pts',(0.183724105301078,-0.181908769287581,
-1.32927485816855));
#50209=CARTESIAN_POINT('Ctrl Pts',(0.107906724710694,-0.234949967082449,
-1.33351461577555));
#50210=CARTESIAN_POINT('Ctrl Pts',(0.0271814967732379,-0.243944758897442,
-1.33775437338254));
#50211=CARTESIAN_POINT('Ctrl Pts',(-0.0535437311642181,-0.252939550712434,
-1.34199413098954));
#50212=CARTESIAN_POINT('Ctrl Pts',(-0.139176806448746,-0.21788793654755,
-1.34623388859653));
#50213=CARTESIAN_POINT('Ctrl Pts',(-0.190426677209,-0.154872697333372,-1.35047364620353));
#50214=CARTESIAN_POINT('Ctrl Pts',(-0.225455888131193,-0.111801874461019,
-1.35337151426195));
#50215=CARTESIAN_POINT('Ctrl Pts',(-0.244422289497751,-0.0556672784509742,
-1.35626938232037));
#50216=CARTESIAN_POINT('Ctrl Pts',(-0.244854737116733,0.000201854273987251,
-1.35916725037879));
#50217=CARTESIAN_POINT('Ctrl Pts',(-0.244810640388203,0.000186482913498504,
-1.37073274962121));
#50218=CARTESIAN_POINT('Ctrl Pts',(-0.244428472433774,-0.0539105270476947,
-1.36792807513019));
#50219=CARTESIAN_POINT('Ctrl Pts',(-0.226760440538336,-0.108234224483701,
-1.36512340063918));
#50220=CARTESIAN_POINT('Ctrl Pts',(-0.193781152536664,-0.150654232462379,
-1.36231872614817));
#50221=CARTESIAN_POINT('Ctrl Pts',(-0.143927172109908,-0.214779517622103,
-1.35807896854117));
#50222=CARTESIAN_POINT('Ctrl Pts',(-0.0590844803015342,-0.251702935612399,
-1.35383921093418));
#50223=CARTESIAN_POINT('Ctrl Pts',(0.0218187473288031,-0.244482765576226,
-1.34959945332718));
#50224=CARTESIAN_POINT('Ctrl Pts',(0.10272197495914,-0.237262595540053,
-1.34535969572019));
#50225=CARTESIAN_POINT('Ctrl Pts',(0.179685738411441,-0.185898837477412,
-1.34111993811319));
#50226=CARTESIAN_POINT('Ctrl Pts',(0.217396563364921,-0.11395882571878,
-1.3368801805062));
#50227=CARTESIAN_POINT('Ctrl Pts',(0.2551073883184,-0.0420188139601475,
-1.3326404228992));
#50228=CARTESIAN_POINT('Ctrl Pts',(0.253565274773058,0.0504974514944755,
-1.32840066529221));
#50229=CARTESIAN_POINT('Ctrl Pts',(0.213477862795548,0.121140699626764,
-1.32416090768521));
#50230=CARTESIAN_POINT('Ctrl Pts',(0.173390450818038,0.191783947759052,
-1.31992115007821));
#50231=CARTESIAN_POINT('Ctrl Pts',(0.0947577404083598,0.240554178569004,
-1.31568139247122));
#50232=CARTESIAN_POINT('Ctrl Pts',(0.0136587974671215,0.245074094240732,
-1.31144163486423));
#50233=CARTESIAN_POINT('Ctrl Pts',(-0.0674401454741175,0.24959400991246,
-1.30720187725723));
#50234=CARTESIAN_POINT('Ctrl Pts',(-0.151005320946917,0.209863610445962,
-1.30296211965023));
#50235=CARTESIAN_POINT('Ctrl Pts',(-0.198694439746781,0.144112432926045,
-1.29872236204324));
#50236=CARTESIAN_POINT('Ctrl Pts',(-0.22865036421838,0.102810824566048,
-1.29605915790256));
#50237=CARTESIAN_POINT('Ctrl Pts',(-0.244450581848228,0.0512421316912588,
-1.29339595376188));
#50238=CARTESIAN_POINT('Ctrl Pts',(-0.244751695427407,-0.000157197744526027,
-1.29073274962121));
#50239=CARTESIAN_POINT('Origin',(0.,0.,-0.775));
#50240=CARTESIAN_POINT('',(-0.245346864912507,-0.000144723283361653,-1.1991672503788));
#50241=CARTESIAN_POINT('',(-0.245384515459765,-0.000118217032388335,-1.21073274962121));
#50242=CARTESIAN_POINT('',(-0.24505,-3.00099698131059E-17,-0.775));
#50243=CARTESIAN_POINT('Ctrl Pts',(-0.245346864912507,-0.000144723283361653,
-1.1991672503788));
#50244=CARTESIAN_POINT('Ctrl Pts',(-0.24483734676681,0.0727041776369625,
-1.20296538197676));
#50245=CARTESIAN_POINT('Ctrl Pts',(-0.210320245808661,0.145972253025746,
-1.20676351357472));
#50246=CARTESIAN_POINT('Ctrl Pts',(-0.153552896413428,0.191492521208896,
-1.21056164517268));
#50247=CARTESIAN_POINT('Ctrl Pts',(-0.0901849495111878,0.242305637691093,
-1.21480140277968));
#50248=CARTESIAN_POINT('Ctrl Pts',(0.000908338903704564,0.258543075920582,
-1.21904116038667));
#50249=CARTESIAN_POINT('Ctrl Pts',(0.0779305696397273,0.23275460038141,
-1.22328091799367));
#50250=CARTESIAN_POINT('Ctrl Pts',(0.15495280037575,0.206966124842239,-1.22752067560066));
#50251=CARTESIAN_POINT('Ctrl Pts',(0.217903973432903,0.139151735534406,
-1.23176043320766));
#50252=CARTESIAN_POINT('Ctrl Pts',(0.237900156835131,0.0604267576219127,
-1.23600019081465));
#50253=CARTESIAN_POINT('Ctrl Pts',(0.25789634023736,-0.0182982202905806,
-1.24023994842165));
#50254=CARTESIAN_POINT('Ctrl Pts',(0.234937533984665,-0.107933786807734,
-1.24447970602864));
#50255=CARTESIAN_POINT('Ctrl Pts',(0.179557943493476,-0.167352390514998,
-1.24871946363564));
#50256=CARTESIAN_POINT('Ctrl Pts',(0.124178353002287,-0.226770994222261,
-1.25295922124264));
#50257=CARTESIAN_POINT('Ctrl Pts',(0.0363779782726041,-0.255972635119634,
-1.25719897884963));
#50258=CARTESIAN_POINT('Ctrl Pts',(-0.0435576711461274,-0.241558703022307,
-1.26143873645663));
#50259=CARTESIAN_POINT('Ctrl Pts',(-0.123493320564858,-0.22714477092498,
-1.26567849406362));
#50260=CARTESIAN_POINT('Ctrl Pts',(-0.195564244672638,-0.169115265832955,
-1.26991825167062));
#50261=CARTESIAN_POINT('Ctrl Pts',(-0.226702090152149,-0.0940959078578519,
-1.27415800927761));
#50262=CARTESIAN_POINT('Ctrl Pts',(-0.238965132039332,-0.0645509757974888,
-1.27582775631134));
#50263=CARTESIAN_POINT('Ctrl Pts',(-0.244879343685111,-0.0323708720032655,
-1.27749750334507));
#50264=CARTESIAN_POINT('Ctrl Pts',(-0.244719259061378,-0.000134367261369422,
-1.27916725037879));
#50265=CARTESIAN_POINT('Ctrl Pts',(-0.244751695427407,-0.000157197744526027,
-1.29073274962121));
#50266=CARTESIAN_POINT('Ctrl Pts',(-0.244929947499698,-0.0305843774528814,
-1.28915619615489));
#50267=CARTESIAN_POINT('Ctrl Pts',(-0.2396767583184,-0.0609522061454329,
-1.28757964268857));
#50268=CARTESIAN_POINT('Ctrl Pts',(-0.228713440581758,-0.0890956461841305,
-1.28600308922225));
#50269=CARTESIAN_POINT('Ctrl Pts',(-0.199230260489943,-0.164780592201052,
-1.28176333161526));
#50270=CARTESIAN_POINT('Ctrl Pts',(-0.128450838179383,-0.224378528661559,
-1.27752357400826));
#50271=CARTESIAN_POINT('Ctrl Pts',(-0.0488509415881311,-0.240544088895643,
-1.27328381640127));
#50272=CARTESIAN_POINT('Ctrl Pts',(0.0307489550031208,-0.256709649129727,
-1.26904405879427));
#50273=CARTESIAN_POINT('Ctrl Pts',(0.119169325875064,-0.229442833137387,
-1.26480430118728));
#50274=CARTESIAN_POINT('Ctrl Pts',(0.175840185746171,-0.171254495081629,
-1.26056454358028));
#50275=CARTESIAN_POINT('Ctrl Pts',(0.232511045617277,-0.113066157025871,
-1.25632478597329));
#50276=CARTESIAN_POINT('Ctrl Pts',(0.257432394487546,-0.0239562969066957,
-1.25208502836629));
#50277=CARTESIAN_POINT('Ctrl Pts',(0.239169553386271,0.0551887446749379,
-1.2478452707593));
#50278=CARTESIAN_POINT('Ctrl Pts',(0.220906712284997,0.134333786256571,
-1.2436055131523));
#50279=CARTESIAN_POINT('Ctrl Pts',(0.159459681212178,0.203514009300662,
-1.2393657555453));
#50280=CARTESIAN_POINT('Ctrl Pts',(0.0830222449175702,0.230987401867944,
-1.23512599793831));
#50281=CARTESIAN_POINT('Ctrl Pts',(0.00658480862296257,0.258460794435227,
-1.23088624033131));
#50282=CARTESIAN_POINT('Ctrl Pts',(-0.0848430328934345,0.2442273565257,
-1.22664648272432));
#50283=CARTESIAN_POINT('Ctrl Pts',(-0.149311376844718,0.19481782690153,
-1.22240672511732));
#50284=CARTESIAN_POINT('Ctrl Pts',(-0.20848157298366,0.149468879188461,
-1.21851539995195));
#50285=CARTESIAN_POINT('Ctrl Pts',(-0.244941369133683,0.0744879581436564,
-1.21462407478658));
#50286=CARTESIAN_POINT('Ctrl Pts',(-0.245384515459765,-0.000118217032388335,
-1.21073274962121));
#50287=CARTESIAN_POINT('Origin',(0.,0.,-0.775));
#50288=CARTESIAN_POINT('',(-0.245167484065513,0.000212043117031907,-1.1191672503788));
#50289=CARTESIAN_POINT('',(-0.245113203773488,0.00022073262402164,-1.13073274962121));
#50290=CARTESIAN_POINT('',(-0.24505,-3.00099698131059E-17,-0.775));
#50291=CARTESIAN_POINT('Ctrl Pts',(-0.245167484065513,0.000212043117031907,
-1.1191672503788));
#50292=CARTESIAN_POINT('Ctrl Pts',(-0.245305444362438,0.0153259129849596,
-1.11995374539446));
#50293=CARTESIAN_POINT('Ctrl Pts',(-0.244028163778416,0.030416526229839,
-1.12074024041012));
#50294=CARTESIAN_POINT('Ctrl Pts',(-0.241251890522508,0.0452261317696372,
-1.12152673542578));
#50295=CARTESIAN_POINT('Ctrl Pts',(-0.226285838072791,0.125060252131,-1.12576649303278));
#50296=CARTESIAN_POINT('Ctrl Pts',(-0.167759610554573,0.196728392058633,
-1.13000625063977));
#50297=CARTESIAN_POINT('Ctrl Pts',(-0.0925268390960716,0.227347007287172,
-1.13424600824677));
#50298=CARTESIAN_POINT('Ctrl Pts',(-0.0172940676375692,0.257965622515711,
-1.13848576585376));
#50299=CARTESIAN_POINT('Ctrl Pts',(0.0746452477612181,0.247534713045156,
-1.14272552346076));
#50300=CARTESIAN_POINT('Ctrl Pts',(0.141106524790587,0.200840300580519,
-1.14696528106775));
#50301=CARTESIAN_POINT('Ctrl Pts',(0.207567801819956,0.154145888115883,
-1.15120503867475));
#50302=CARTESIAN_POINT('Ctrl Pts',(0.248551040479906,0.0711879726571643,
-1.15544479628174));
#50303=CARTESIAN_POINT('Ctrl Pts',(0.245251871857863,-0.00996980568939554,
-1.15968455388874));
#50304=CARTESIAN_POINT('Ctrl Pts',(0.241952703235821,-0.091127584035954,
-1.16392431149573));
#50305=CARTESIAN_POINT('Ctrl Pts',(0.194371127331788,-0.170485225270353,
-1.16816406910273));
#50306=CARTESIAN_POINT('Ctrl Pts',(0.124339032886921,-0.211631005706291,
-1.17240382670972));
#50307=CARTESIAN_POINT('Ctrl Pts',(0.0543069384420516,-0.25277678614223,
-1.17664358431672));
#50308=CARTESIAN_POINT('Ctrl Pts',(-0.0381756745436533,-0.255710705779704,
-1.18088334192371));
#50309=CARTESIAN_POINT('Ctrl Pts',(-0.110674942130753,-0.219086592152763,
-1.18512309953071));
#50310=CARTESIAN_POINT('Ctrl Pts',(-0.183174209717853,-0.182462478525821,
-1.18936285713771));
#50311=CARTESIAN_POINT('Ctrl Pts',(-0.235690131906348,-0.106280331634464,
-1.1936026147447));
#50312=CARTESIAN_POINT('Ctrl Pts',(-0.244126790305802,-0.0254948608213339,
-1.1978423723517));
#50313=CARTESIAN_POINT('Ctrl Pts',(-0.245005578228106,-0.0170800012066754,
-1.19828399836073));
#50314=CARTESIAN_POINT('Ctrl Pts',(-0.245406108901139,-0.00861519581599708,
-1.19872562436976));
#50315=CARTESIAN_POINT('Ctrl Pts',(-0.245346864912507,-0.000144723283361653,
-1.1991672503788));
#50316=CARTESIAN_POINT('Ctrl Pts',(-0.245384515459765,-0.000118217032388335,
-1.21073274962121));
#50317=CARTESIAN_POINT('Ctrl Pts',(-0.245424195144662,-0.0067985150470858,
-1.21038431717958));
#50318=CARTESIAN_POINT('Ctrl Pts',(-0.245175109242132,-0.0134758085149568,
-1.21003588473796));
#50319=CARTESIAN_POINT('Ctrl Pts',(-0.244627705212326,-0.020128555650413,
-1.20968745229634));
#50320=CARTESIAN_POINT('Ctrl Pts',(-0.237966843242477,-0.101079787239374,
-1.20544769468934));
#50321=CARTESIAN_POINT('Ctrl Pts',(-0.18713627291661,-0.178396629078483,
-1.20120793708235));
#50322=CARTESIAN_POINT('Ctrl Pts',(-0.115458621318355,-0.216603738881799,
-1.19696817947535));
#50323=CARTESIAN_POINT('Ctrl Pts',(-0.0437809697200995,-0.254810848685115,
-1.19272842186835));
#50324=CARTESIAN_POINT('Ctrl Pts',(0.0487437631505439,-0.253908226452637,
-1.18848866426136));
#50325=CARTESIAN_POINT('Ctrl Pts',(0.119662387405715,-0.214310023021451,
-1.18424890665437));
#50326=CARTESIAN_POINT('Ctrl Pts',(0.190581011660885,-0.174711819590264,
-1.18000914904737));
#50327=CARTESIAN_POINT('Ctrl Pts',(0.239893527300583,-0.096418034960368,
-1.17576939144037));
#50328=CARTESIAN_POINT('Ctrl Pts',(0.244973837284843,-0.015352262714056,
-1.17152963383338));
#50329=CARTESIAN_POINT('Ctrl Pts',(0.250054147269103,0.0657135095322565,
-1.16728987622638));
#50330=CARTESIAN_POINT('Ctrl Pts',(0.210902251597925,0.149551269394986,
-1.16305011861939));
#50331=CARTESIAN_POINT('Ctrl Pts',(0.145482242747102,0.197693677120017,
-1.15881036101239));
#50332=CARTESIAN_POINT('Ctrl Pts',(0.0800622338962787,0.245836084845048,
-1.1545706034054));
#50333=CARTESIAN_POINT('Ctrl Pts',(-0.0116258881341887,0.258283140432381,
-1.1503308457984));
#50334=CARTESIAN_POINT('Ctrl Pts',(-0.0875127962613097,0.229323752405274,
-1.14609108819141));
#50335=CARTESIAN_POINT('Ctrl Pts',(-0.163399704388431,0.200364364378166,
-1.14185133058441));
#50336=CARTESIAN_POINT('Ctrl Pts',(-0.223485398612205,0.129998532736619,
-1.13761157297742));
#50337=CARTESIAN_POINT('Ctrl Pts',(-0.240200716576505,0.050512262695319,
-1.13337181537042));
#50338=CARTESIAN_POINT('Ctrl Pts',(-0.243668904085937,0.0340200075364671,
-1.13249212678735));
#50339=CARTESIAN_POINT('Ctrl Pts',(-0.245269985293028,0.0171351150642011,
-1.13161243820428));
#50340=CARTESIAN_POINT('Ctrl Pts',(-0.245113203773488,0.00022073262402164,
-1.13073274962121));
#50341=CARTESIAN_POINT('Origin',(0.,0.,-0.775));
#50342=CARTESIAN_POINT('',(-0.244649653071174,3.34626584120729E-5,-1.03916725037879));
#50343=CARTESIAN_POINT('',(-0.244645538675098,3.85059038551794E-6,-1.05073274962121));
#50344=CARTESIAN_POINT('',(-0.24505,-3.00099698131059E-17,-0.775));
#50345=CARTESIAN_POINT('Ctrl Pts',(-0.244649653071174,3.34626584120729E-5,
-1.03916725037879));
#50346=CARTESIAN_POINT('Ctrl Pts',(-0.244696975754832,0.0389557362310942,
-1.04118186641915));
#50347=CARTESIAN_POINT('Ctrl Pts',(-0.235956892958235,0.0778579314244324,
-1.04319648245951));
#50348=CARTESIAN_POINT('Ctrl Pts',(-0.218316444296445,0.112186486821377,
-1.04521109849987));
#50349=CARTESIAN_POINT('Ctrl Pts',(-0.18119213628617,0.184430900131816,
-1.04945085610686));
#50350=CARTESIAN_POINT('Ctrl Pts',(-0.104648852062527,0.236419045208656,
-1.05369061371385));
#50351=CARTESIAN_POINT('Ctrl Pts',(-0.0238070018601966,0.244297163999081,
-1.05793037132085));
#50352=CARTESIAN_POINT('Ctrl Pts',(0.0570348483421337,0.252175282789506,
-1.06217012892784));
#50353=CARTESIAN_POINT('Ctrl Pts',(0.142175264523152,0.215943375293518,
-1.06640988653484));
#50354=CARTESIAN_POINT('Ctrl Pts',(0.192549208199601,0.152225753725436,
-1.07064964414184));
#50355=CARTESIAN_POINT('Ctrl Pts',(0.242923151876051,0.0885081321573535,
-1.07488940174883));
#50356=CARTESIAN_POINT('Ctrl Pts',(0.258530623047931,-0.00269520348282262,
-1.07912915935583));
#50357=CARTESIAN_POINT('Ctrl Pts',(0.232210434475385,-0.0795373610092435,
-1.08336891696282));
#50358=CARTESIAN_POINT('Ctrl Pts',(0.205890245902839,-0.156379518535664,
-1.08760867456982));
#50359=CARTESIAN_POINT('Ctrl Pts',(0.137642397585865,-0.21886049794833,
-1.09184843217681));
#50360=CARTESIAN_POINT('Ctrl Pts',(0.0587810989267877,-0.238312106458149,
-1.09608818978381));
#50361=CARTESIAN_POINT('Ctrl Pts',(-0.0200801997322901,-0.257763714967968,
-1.1003279473908));
#50362=CARTESIAN_POINT('Ctrl Pts',(-0.109554948733473,-0.234185952574941,
-1.1045677049978));
#50363=CARTESIAN_POINT('Ctrl Pts',(-0.168589384543456,-0.17839702098088,
-1.10880746260479));
#50364=CARTESIAN_POINT('Ctrl Pts',(-0.216672654314996,-0.132957199098996,
-1.11226072519613));
#50365=CARTESIAN_POINT('Ctrl Pts',(-0.244561741978186,-0.0661484046745886,
-1.11571398778746));
#50366=CARTESIAN_POINT('Ctrl Pts',(-0.245167484065513,0.000212043117031907,
-1.1191672503788));
#50367=CARTESIAN_POINT('Ctrl Pts',(-0.245113203773488,0.00022073262402164,
-1.13073274962121));
#50368=CARTESIAN_POINT('Ctrl Pts',(-0.244514359207961,-0.0643856446664852,
-1.12737268059728));
#50369=CARTESIAN_POINT('Ctrl Pts',(-0.218269289868647,-0.129422263940181,
-1.12401261157336));
#50370=CARTESIAN_POINT('Ctrl Pts',(-0.172465701285927,-0.174652382769037,
-1.12065254254943));
#50371=CARTESIAN_POINT('Ctrl Pts',(-0.114670426326225,-0.231724049751042,
-1.11641278494244));
#50372=CARTESIAN_POINT('Ctrl Pts',(-0.025734934701994,-0.257260675273999,
-1.11217302733544));
#50373=CARTESIAN_POINT('Ctrl Pts',(0.0535344379030858,-0.239545271055687,
-1.10793326972845));
#50374=CARTESIAN_POINT('Ctrl Pts',(0.132803810508166,-0.221829866837375,
-1.10369351212145));
#50375=CARTESIAN_POINT('Ctrl Pts',(0.202407064094095,-0.160862432877793,
-1.09945375451446));
#50376=CARTESIAN_POINT('Ctrl Pts',(0.230408087683255,-0.0846167008153363,
-1.09521399690746));
#50377=CARTESIAN_POINT('Ctrl Pts',(0.258409111272416,-0.00837096875287918,
-1.09097423930047));
#50378=CARTESIAN_POINT('Ctrl Pts',(0.244807904864808,0.0831530614124536,
-1.08673448169347));
#50379=CARTESIAN_POINT('Ctrl Pts',(0.195845119793085,0.147961352994708,
-1.08249472408648));
#50380=CARTESIAN_POINT('Ctrl Pts',(0.146882334721362,0.212769644576962,
-1.07825496647948));
#50381=CARTESIAN_POINT('Ctrl Pts',(0.0625579709855245,0.250862197576139,
-1.07401520887249));
#50382=CARTESIAN_POINT('Ctrl Pts',(-0.0184373628622437,0.24476097846153,
-1.06977545126549));
#50383=CARTESIAN_POINT('Ctrl Pts',(-0.0994326967100126,0.23865975934692,
-1.0655356936585));
#50384=CARTESIAN_POINT('Ctrl Pts',(-0.177099000669712,0.188364768118525,
-1.0612959360515));
#50385=CARTESIAN_POINT('Ctrl Pts',(-0.215800588552335,0.116952891829257,
-1.0570561784445));
#50386=CARTESIAN_POINT('Ctrl Pts',(-0.235041211799334,0.0814502398137821,
-1.05494836883674));
#50387=CARTESIAN_POINT('Ctrl Pts',(-0.244651260008812,0.040728308239459,
-1.05284055922897));
#50388=CARTESIAN_POINT('Ctrl Pts',(-0.244645568296149,3.85030838442385E-6,
-1.05073274962121));
#50389=CARTESIAN_POINT('Origin',(0.,0.,-0.775));
#50390=CARTESIAN_POINT('',(-0.245044321574299,-0.000225594368389231,-0.959167250378794));
#50391=CARTESIAN_POINT('',(-0.245099029133644,-0.000222287294248484,-0.970732749621207));
#50392=CARTESIAN_POINT('',(-0.24505,-3.00099698131059E-17,-0.775));
#50393=CARTESIAN_POINT('Ctrl Pts',(-0.245044321574299,-0.000225594368389231,
-0.959167250378794));
#50394=CARTESIAN_POINT('Ctrl Pts',(-0.244469510773935,0.0621696777858805,
-0.962409987443846));
#50395=CARTESIAN_POINT('Ctrl Pts',(-0.220208236993727,0.124962399432046,
-0.965652724508897));
#50396=CARTESIAN_POINT('Ctrl Pts',(-0.177227576931743,0.169818325425937,
-0.968895461573948));
#50397=CARTESIAN_POINT('Ctrl Pts',(-0.121031969086925,0.228465773441711,
-0.973135219180944));
#50398=CARTESIAN_POINT('Ctrl Pts',(-0.0328363455678891,0.256451012057126,
-0.977374976787939));
#50399=CARTESIAN_POINT('Ctrl Pts',(0.0468924321585544,0.240933554080418,
-0.981614734394934));
#50400=CARTESIAN_POINT('Ctrl Pts',(0.126621209884998,0.22541609610371,-0.98585449200193));
#50401=CARTESIAN_POINT('Ctrl Pts',(0.197883141818849,0.166395941534881,
-0.990094249608925));
#50402=CARTESIAN_POINT('Ctrl Pts',(0.227981064400714,0.0909533504071397,
-0.994334007215921));
#50403=CARTESIAN_POINT('Ctrl Pts',(0.258078986982579,0.0155107592793984,
-0.998573764822916));
#50404=CARTESIAN_POINT('Ctrl Pts',(0.24701290021246,-0.0763542684072548,
-1.00281352242991));
#50405=CARTESIAN_POINT('Ctrl Pts',(0.199860264654025,-0.142491235828697,
-1.00705328003691));
#50406=CARTESIAN_POINT('Ctrl Pts',(0.15270762909559,-0.208628203250139,
-1.0112930376439));
#50407=CARTESIAN_POINT('Ctrl Pts',(0.0694684447488411,-0.249037110406371,
-1.0155327952509));
#50408=CARTESIAN_POINT('Ctrl Pts',(-0.0116645934749716,-0.245177109320242,
-1.01977255285789));
#50409=CARTESIAN_POINT('Ctrl Pts',(-0.0927976316987844,-0.241317108234113,
-1.02401231046489));
#50410=CARTESIAN_POINT('Ctrl Pts',(-0.17182452379966,-0.193188198905624,
-1.02825206807188));
#50411=CARTESIAN_POINT('Ctrl Pts',(-0.212485303951644,-0.122873403469361,
-1.03249182567888));
#50412=CARTESIAN_POINT('Ctrl Pts',(-0.233825201284185,-0.0859702621631733,
-1.03471696724552));
#50413=CARTESIAN_POINT('Ctrl Pts',(-0.244597385210529,-0.0429561527619699,
-1.03694210881216));
#50414=CARTESIAN_POINT('Ctrl Pts',(-0.244649653071174,3.34626584120729E-5,
-1.03916725037879));
#50415=CARTESIAN_POINT('Ctrl Pts',(-0.244645568296149,3.85030838442385E-6,
-1.05073274962121));
#50416=CARTESIAN_POINT('Ctrl Pts',(-0.244639811402652,-0.0411869793974703,
-1.04860080162198));
#50417=CARTESIAN_POINT('Ctrl Pts',(-0.234796816845105,-0.082380393654487,
-1.04646885362275));
#50418=CARTESIAN_POINT('Ctrl Pts',(-0.215131935267918,-0.118178354002115,
-1.04433690562352));
#50419=CARTESIAN_POINT('Ctrl Pts',(-0.176024822295332,-0.189368962194075,
-1.04009714801652));
#50420=CARTESIAN_POINT('Ctrl Pts',(-0.0980737245446141,-0.239221417227855,
-1.03585739040953));
#50421=CARTESIAN_POINT('Ctrl Pts',(-0.0170450003451614,-0.244861881251446,
-1.03161763280253));
#50422=CARTESIAN_POINT('Ctrl Pts',(0.0639837238542925,-0.250502345275036,
-1.02737787519554));
#50423=CARTESIAN_POINT('Ctrl Pts',(0.148090074502482,-0.211930818288436,
-1.02313811758854));
#50424=CARTESIAN_POINT('Ctrl Pts',(0.196683474149454,-0.146845101802087,
-1.01889835998155));
#50425=CARTESIAN_POINT('Ctrl Pts',(0.245276873796425,-0.0817593853157384,
-1.01465860237455));
#50426=CARTESIAN_POINT('Ctrl Pts',(0.258357322442181,0.00984052067035691,
-1.01041884476756));
#50427=CARTESIAN_POINT('Ctrl Pts',(0.229923108412695,0.0859257653129111,
-1.00617908716056));
#50428=CARTESIAN_POINT('Ctrl Pts',(0.201488894383209,0.162011009955465,
-1.00193932955357));
#50429=CARTESIAN_POINT('Ctrl Pts',(0.131540017678481,0.222581593254477,
-0.99769957194657));
#50430=CARTESIAN_POINT('Ctrl Pts',(0.0521711717813305,0.23984587084569,
-0.993459814339575));
#50431=CARTESIAN_POINT('Ctrl Pts',(-0.0271976741158197,0.257110148436903,
-0.98922005673258));
#50432=CARTESIAN_POINT('Ctrl Pts',(-0.115986489205392,0.231068120320316,
-0.984980299125584));
#50433=CARTESIAN_POINT('Ctrl Pts',(-0.173456237504991,0.173668669014814,
-0.980740541518589));
#50434=CARTESIAN_POINT('Ctrl Pts',(-0.218674646565952,0.128505571110223,
-0.977404610886129));
#50435=CARTESIAN_POINT('Ctrl Pts',(-0.244503815935465,0.0639294875508147,
-0.974068680253668));
#50436=CARTESIAN_POINT('Ctrl Pts',(-0.245099029133644,-0.000222287294248484,
-0.970732749621207));
#50437=CARTESIAN_POINT('Origin',(0.,0.,-0.775));
#50438=CARTESIAN_POINT('',(-0.245422031604165,8.10237884523012E-5,-0.879167250378794));
#50439=CARTESIAN_POINT('',(-0.24539320090154,0.000110883525149794,-0.890732749621207));
#50440=CARTESIAN_POINT('',(-0.24505,-3.00099698131059E-17,-0.775));
#50441=CARTESIAN_POINT('Ctrl Pts',(-0.245422031604165,8.10237884523012E-5,
-0.879167250378794));
#50442=CARTESIAN_POINT('Ctrl Pts',(-0.245441074602344,0.00450998645013945,
-0.879398350861545));
#50443=CARTESIAN_POINT('Ctrl Pts',(-0.245331595776088,0.00893798850812526,
-0.879629451344296));
#50444=CARTESIAN_POINT('Ctrl Pts',(-0.245090635265792,0.013358824071627,
-0.879860551827046));
#50445=CARTESIAN_POINT('Ctrl Pts',(-0.240669986099019,0.0944632466437396,
-0.884100309434042));
#50446=CARTESIAN_POINT('Ctrl Pts',(-0.191996042349709,0.173155614686405,
-0.888340067041037));
#50447=CARTESIAN_POINT('Ctrl Pts',(-0.121401904688346,0.213329452288258,
-0.892579824648033));
#50448=CARTESIAN_POINT('Ctrl Pts',(-0.0508077670269831,0.253503289890111,
-0.896819582255028));
#50449=CARTESIAN_POINT('Ctrl Pts',(0.0417065645464325,0.255158597051152,
-0.901059339862023));
#50450=CARTESIAN_POINT('Ctrl Pts',(0.11369267263772,0.217535867994358,-0.905299097469018));
#50451=CARTESIAN_POINT('Ctrl Pts',(0.185678780729008,0.179913138937563,
-0.909538855076014));
#50452=CARTESIAN_POINT('Ctrl Pts',(0.237136665338167,0.103012373662934,
-0.913778612683009));
#50453=CARTESIAN_POINT('Ctrl Pts',(0.24445586820471,0.0221180056932788,
-0.918018370290005));
#50454=CARTESIAN_POINT('Ctrl Pts',(0.251775071071252,-0.058776362276376,
-0.922258127897));
#50455=CARTESIAN_POINT('Ctrl Pts',(0.214955592195177,-0.143664332941056,
-0.926497885503995));
#50456=CARTESIAN_POINT('Ctrl Pts',(0.150891339590376,-0.193596697575626,
-0.93073764311099));
#50457=CARTESIAN_POINT('Ctrl Pts',(0.0868270869855739,-0.243529062210196,
-0.934977400717986));
#50458=CARTESIAN_POINT('Ctrl Pts',(-0.0044819393479547,-0.258505820814656,
-0.939217158324981));
#50459=CARTESIAN_POINT('Ctrl Pts',(-0.0811403530874316,-0.231655176450718,
-0.943456915931977));
#50460=CARTESIAN_POINT('Ctrl Pts',(-0.157798766826908,-0.20480453208678,
-0.947696673538972));
#50461=CARTESIAN_POINT('Ctrl Pts',(-0.219806567972333,-0.136126484754444,
-0.951936431145967));
#50462=CARTESIAN_POINT('Ctrl Pts',(-0.238712672459747,-0.0571326323802092,
-0.956176188752962));
#50463=CARTESIAN_POINT('Ctrl Pts',(-0.243158628169807,-0.0385564540216952,
-0.957173209294906));
#50464=CARTESIAN_POINT('Ctrl Pts',(-0.245221054428119,-0.0194098102977235,
-0.95817022983685));
#50465=CARTESIAN_POINT('Ctrl Pts',(-0.245044321574299,-0.000225594368389231,
-0.959167250378794));
#50466=CARTESIAN_POINT('Ctrl Pts',(-0.245099029133644,-0.000222287294248484,
-0.970732749621207));
#50467=CARTESIAN_POINT('Ctrl Pts',(-0.245260294400637,-0.017603375499452,
-0.969828922646673));
#50468=CARTESIAN_POINT('Ctrl Pts',(-0.243569214490148,-0.0349533165394845,
-0.968925095672138));
#50469=CARTESIAN_POINT('Ctrl Pts',(-0.239909546000387,-0.0518775738123231,
-0.968021268697603));
#50470=CARTESIAN_POINT('Ctrl Pts',(-0.22274242468656,-0.131267490839541,
-0.963781511090608));
#50471=CARTESIAN_POINT('Ctrl Pts',(-0.162257500549283,-0.201290450399556,
-0.959541753483612));
#50472=CARTESIAN_POINT('Ctrl Pts',(-0.0862071148979349,-0.2298177675197,
-0.955301995876616));
#50473=CARTESIAN_POINT('Ctrl Pts',(-0.0101567292465875,-0.258345084639844,
-0.951062238269621));
#50474=CARTESIAN_POINT('Ctrl Pts',(0.0814591179188316,-0.245376759320117,
-0.946822480662627));
#50475=CARTESIAN_POINT('Ctrl Pts',(0.146604261452242,-0.196863057608093,
-0.942582723055632));
#50476=CARTESIAN_POINT('Ctrl Pts',(0.211749404985652,-0.14834935589607,
-0.938342965448636));
#50477=CARTESIAN_POINT('Ctrl Pts',(0.250423844887055,-0.0642902777917504,
-0.93410320784164));
#50478=CARTESIAN_POINT('Ctrl Pts',(0.244882560039177,0.016745289350255,
-0.929863450234645));
#50479=CARTESIAN_POINT('Ctrl Pts',(0.239341275191298,0.0977808564922616,
-0.925623692627649));
#50480=CARTESIAN_POINT('Ctrl Pts',(0.189584265594134,0.175792912671955,
-0.921383935020655));
#50481=CARTESIAN_POINT('Ctrl Pts',(0.118441575801277,0.214987129960086,
-0.91714417741366));
#50482=CARTESIAN_POINT('Ctrl Pts',(0.0472988860084194,0.254181347248218,
-0.912904419806664));
#50483=CARTESIAN_POINT('Ctrl Pts',(-0.0452294839801312,0.254557725644789,
-0.908664662199669));
#50484=CARTESIAN_POINT('Ctrl Pts',(-0.116688675514067,0.215943571178994,
-0.904424904592673));
#50485=CARTESIAN_POINT('Ctrl Pts',(-0.188147867048003,0.1773294167132,-0.900185146985678));
#50486=CARTESIAN_POINT('Ctrl Pts',(-0.238537880127323,0.0997247293850409,
-0.895945389378683));
#50487=CARTESIAN_POINT('Ctrl Pts',(-0.244738228754766,0.0187369237801842,
-0.891705631771688));
#50488=CARTESIAN_POINT('Ctrl Pts',(-0.245212486095677,0.0125422622151333,
-0.891381337721528));
#50489=CARTESIAN_POINT('Ctrl Pts',(-0.245428210065485,0.00632780758345109,
-0.891057043671367));
#50490=CARTESIAN_POINT('Ctrl Pts',(-0.24539320090154,0.000110883525149794,
-0.890732749621207));
#50491=CARTESIAN_POINT('Origin',(0.,0.,-0.775));
#50492=CARTESIAN_POINT('',(-0.244799711053798,0.000182046184206572,-0.799167250378795));
#50493=CARTESIAN_POINT('',(-0.244760945085023,0.000162685199137168,-0.810732749621207));
#50494=CARTESIAN_POINT('',(-0.24505,-3.00099698131059E-17,-0.775));
#50495=CARTESIAN_POINT('Ctrl Pts',(-0.244799711053798,0.000182046184206572,
-0.799167250378795));
#50496=CARTESIAN_POINT('Ctrl Pts',(-0.244993156130942,0.0283308761463506,
-0.80062647188624));
#50497=CARTESIAN_POINT('Ctrl Pts',(-0.240512320471579,0.0564200071496143,
-0.802085693393685));
#50498=CARTESIAN_POINT('Ctrl Pts',(-0.231088852819787,0.0827394692876446,
-0.803544914901131));
#50499=CARTESIAN_POINT('Ctrl Pts',(-0.203709035254664,0.159210477453564,
-0.807784672508126));
#50500=CARTESIAN_POINT('Ctrl Pts',(-0.134604069490859,0.22074213836936,
-0.812024430115121));
#50501=CARTESIAN_POINT('Ctrl Pts',(-0.0554814367462919,0.239101835735599,
-0.816264187722116));
#50502=CARTESIAN_POINT('Ctrl Pts',(0.023641195998275,0.257461533101838,
-0.820503945329112));
#50503=CARTESIAN_POINT('Ctrl Pts',(0.112781495723604,0.23264926691852,-0.824743702936108));
#50504=CARTESIAN_POINT('Ctrl Pts',(0.171039154498696,0.176049667150885,
-0.828983460543103));
#50505=CARTESIAN_POINT('Ctrl Pts',(0.229296813273789,0.119450067383251,
-0.833223218150098));
#50506=CARTESIAN_POINT('Ctrl Pts',(0.256671831098645,0.0310631340313012,
-0.837462975757093));
#50507=CARTESIAN_POINT('Ctrl Pts',(0.240603708826379,-0.0485564926097166,
-0.841702733364088));
#50508=CARTESIAN_POINT('Ctrl Pts',(0.224535586554113,-0.128176119250734,
-0.845942490971084));
#50509=CARTESIAN_POINT('Ctrl Pts',(0.165024324184724,-0.199028439180819,
-0.850182248578079));
#50510=CARTESIAN_POINT('Ctrl Pts',(0.0893755170973006,-0.228604231411312,
-0.854422006185075));
#50511=CARTESIAN_POINT('Ctrl Pts',(0.0137267100098771,-0.258180023641804,
-0.85866176379207));
#50512=CARTESIAN_POINT('Ctrl Pts',(-0.0780596417955818,-0.246479288172705,
-0.862901521399065));
#50513=CARTESIAN_POINT('Ctrl Pts',(-0.143869140406192,-0.198870681887375,
-0.867141279006061));
#50514=CARTESIAN_POINT('Ctrl Pts',(-0.206091498357299,-0.153857122988121,
-0.871149936130305));
#50515=CARTESIAN_POINT('Ctrl Pts',(-0.245091712734177,-0.0767435354485706,
-0.87515859325455));
#50516=CARTESIAN_POINT('Ctrl Pts',(-0.245422031604165,8.10237884523012E-5,
-0.879167250378794));
#50517=CARTESIAN_POINT('Ctrl Pts',(-0.24539320090154,0.000110883525149794,
-0.890732749621207));
#50518=CARTESIAN_POINT('Ctrl Pts',(-0.244970507036162,-0.0749510535466689,
-0.886817286064372));
#50519=CARTESIAN_POINT('Ctrl Pts',(-0.207996739432263,-0.150372975727332,
-0.882901822507536));
#50520=CARTESIAN_POINT('Ctrl Pts',(-0.148200946425008,-0.195663876087275,
-0.878986358950701));
#50521=CARTESIAN_POINT('Ctrl Pts',(-0.0834526312922395,-0.244705946468324,
-0.874746601343706));
#50522=CARTESIAN_POINT('Ctrl Pts',(0.00805468314886303,-0.258419163348866,
-0.870506843736711));
#50523=CARTESIAN_POINT('Ctrl Pts',(0.0843346299002956,-0.230511481549932,
-0.866267086129716));
#50524=CARTESIAN_POINT('Ctrl Pts',(0.160614576651729,-0.202603799750998,
-0.862027328522721));
#50525=CARTESIAN_POINT('Ctrl Pts',(0.221667155713491,-0.133075219272589,
-0.857787570915725));
#50526=CARTESIAN_POINT('Ctrl Pts',(0.23947956825832,-0.0538275887772554,
-0.853547813308729));
#50527=CARTESIAN_POINT('Ctrl Pts',(0.257291980803149,0.0254200417180767,
-0.849308055701734));
#50528=CARTESIAN_POINT('Ctrl Pts',(0.231864226831043,0.114386722230333,
-0.845068298094739));
#50529=CARTESIAN_POINT('Ctrl Pts',(0.174863341012712,0.172251806657105,
-0.840828540487743));
#50530=CARTESIAN_POINT('Ctrl Pts',(0.117862455194381,0.230116891083877,
-0.836588782880748));
#50531=CARTESIAN_POINT('Ctrl Pts',(0.029288437529827,0.256880379425167,
-0.832349025273753));
#50532=CARTESIAN_POINT('Ctrl Pts',(-0.0502182316557958,0.240262361047521,
-0.828109267666757));
#50533=CARTESIAN_POINT('Ctrl Pts',(-0.12972490084142,0.223644342669875,
-0.823869510059762));
#50534=CARTESIAN_POINT('Ctrl Pts',(-0.200164221548112,0.163644817573289,
-0.819629752452767));
#50535=CARTESIAN_POINT('Ctrl Pts',(-0.229216469518364,0.08779341107567,
-0.815389994845771));
#50536=CARTESIAN_POINT('Ctrl Pts',(-0.23985414079302,0.0600199207465147,
-0.813837579770917));
#50537=CARTESIAN_POINT('Ctrl Pts',(-0.244943021197934,0.0301211587088129,
-0.812285164696062));
#50538=CARTESIAN_POINT('Ctrl Pts',(-0.244760945085023,0.000162685199137168,
-0.810732749621207));
#50539=CARTESIAN_POINT('Origin',(0.,0.,-0.775));
#50540=CARTESIAN_POINT('',(-0.244760954731183,-0.000162685205530727,-0.719167250378794));
#50541=CARTESIAN_POINT('',(-0.244799701406111,-0.000182046177014158,-0.730732749621206));
#50542=CARTESIAN_POINT('',(-0.24505,-3.00099698131059E-17,-0.775));
#50543=CARTESIAN_POINT('Ctrl Pts',(-0.244760954731183,-0.000162685205530727,
-0.719167250378794));
#50544=CARTESIAN_POINT('Ctrl Pts',(-0.244445767826903,0.0516975965821623,
-0.721854592910934));
#50545=CARTESIAN_POINT('Ctrl Pts',(-0.2283355747708,0.103736810422125,-0.724541935443075));
#50546=CARTESIAN_POINT('Ctrl Pts',(-0.197871599550311,0.145240172703587,
-0.727229277975215));
#50547=CARTESIAN_POINT('Ctrl Pts',(-0.149809296685806,0.210719058943139,
-0.731469035582211));
#50548=CARTESIAN_POINT('Ctrl Pts',(-0.0660195162091051,0.249973539909514,
-0.735708793189205));
#50549=CARTESIAN_POINT('Ctrl Pts',(0.0150524165496374,0.244992453825791,
-0.739948550796201));
#50550=CARTESIAN_POINT('Ctrl Pts',(0.0961243493083799,0.240011367742068,
-0.744188308403196));
#50551=CARTESIAN_POINT('Ctrl Pts',(0.174478434349164,0.190794714608247,
-0.748428066010191));
#50552=CARTESIAN_POINT('Ctrl Pts',(0.214163410394044,0.119924606832621,
-0.752667823617187));
#50553=CARTESIAN_POINT('Ctrl Pts',(0.253848386438923,0.049054499056996,
-0.756907581224182));
#50554=CARTESIAN_POINT('Ctrl Pts',(0.2548642534879,-0.0434690633604349,
-0.761147338831177));
#50555=CARTESIAN_POINT('Ctrl Pts',(0.216744900531158,-0.11519342763068,
-0.765387096438173));
#50556=CARTESIAN_POINT('Ctrl Pts',(0.178625547574417,-0.186917791900926,
-0.769626854045168));
#50557=CARTESIAN_POINT('Ctrl Pts',(0.101370974611958,-0.237842958023986,
-0.773866611652163));
#50558=CARTESIAN_POINT('Ctrl Pts',(0.0204279530028463,-0.244602895346069,
-0.778106369259159));
#50559=CARTESIAN_POINT('Ctrl Pts',(-0.0605150686062649,-0.251362832668151,
-0.782346126866154));
#50560=CARTESIAN_POINT('Ctrl Pts',(-0.145146538862028,-0.213957541189255,
-0.786585884473149));
#50561=CARTESIAN_POINT('Ctrl Pts',(-0.194634939306689,-0.149549717741786,
-0.790825642080145));
#50562=CARTESIAN_POINT('Ctrl Pts',(-0.22709063529231,-0.107309501486582,
-0.793606178179695));
#50563=CARTESIAN_POINT('Ctrl Pts',(-0.244431102848988,-0.0534553470905533,
-0.796386714279245));
#50564=CARTESIAN_POINT('Ctrl Pts',(-0.244799711053798,0.000182046184206572,
-0.799167250378795));
#50565=CARTESIAN_POINT('Ctrl Pts',(-0.244760945085023,0.000162685199137168,
-0.810732749621207));
#50566=CARTESIAN_POINT('Ctrl Pts',(-0.244445758193169,-0.0516975945447203,
-0.808045407089066));
#50567=CARTESIAN_POINT('Ctrl Pts',(-0.228335565771977,-0.103736806333797,
-0.805358064556926));
#50568=CARTESIAN_POINT('Ctrl Pts',(-0.197871591752086,-0.145240166979595,
-0.802670722024785));
#50569=CARTESIAN_POINT('Ctrl Pts',(-0.149809290781742,-0.210719050638588,
-0.79843096441779));
#50570=CARTESIAN_POINT('Ctrl Pts',(-0.0660195136072412,-0.249973530057924,
-0.794191206810795));
#50571=CARTESIAN_POINT('Ctrl Pts',(0.0150524159564132,-0.244992444170509,
-0.7899514492038));
#50572=CARTESIAN_POINT('Ctrl Pts',(0.0961243455200677,-0.240011358283093,
-0.785711691596804));
#50573=CARTESIAN_POINT('Ctrl Pts',(0.174478427472875,-0.190794707088926,
-0.781471933989809));
#50574=CARTESIAN_POINT('Ctrl Pts',(0.21416340195375,-0.119924602106329,
-0.777232176382814));
#50575=CARTESIAN_POINT('Ctrl Pts',(0.253848376434623,-0.0490544971237331,
-0.772992418775818));
#50576=CARTESIAN_POINT('Ctrl Pts',(0.254864243443564,0.0434690616472924,
-0.768752661168824));
#50577=CARTESIAN_POINT('Ctrl Pts',(0.216744891989128,0.115193423090842,
-0.764512903561828));
#50578=CARTESIAN_POINT('Ctrl Pts',(0.178625540534692,0.186917784534393,
-0.760273145954833));
#50579=CARTESIAN_POINT('Ctrl Pts',(0.101370970616877,0.237842948650467,
-0.756033388347837));
#50580=CARTESIAN_POINT('Ctrl Pts',(0.0204279521977738,0.244602885706138,
-0.751793630740841));
#50581=CARTESIAN_POINT('Ctrl Pts',(-0.0605150662213308,0.251362822761809,
-0.747553873133846));
#50582=CARTESIAN_POINT('Ctrl Pts',(-0.145146533141725,0.213957532757076,
-0.743314115526851));
#50583=CARTESIAN_POINT('Ctrl Pts',(-0.194634931636022,0.149549711847952,
-0.739074357919856));
#50584=CARTESIAN_POINT('Ctrl Pts',(-0.227090626342544,0.107309497257462,
-0.736293821820306));
#50585=CARTESIAN_POINT('Ctrl Pts',(-0.244431093215825,0.0534553449838617,
-0.733513285720756));
#50586=CARTESIAN_POINT('Ctrl Pts',(-0.244799701406111,-0.000182046177014158,
-0.730732749621206));
#50587=CARTESIAN_POINT('Origin',(0.,0.,-0.775));
#50588=CARTESIAN_POINT('',(-0.245393210572617,-0.000110883529508943,-0.639167250378794));
#50589=CARTESIAN_POINT('',(-0.245422021931952,-8.10237852447184E-5,-0.650732749621206));
#50590=CARTESIAN_POINT('',(-0.24505,-3.00099698131059E-17,-0.775));
#50591=CARTESIAN_POINT('Ctrl Pts',(-0.245393210572617,-0.000110883529508943,
-0.639167250378794));
#50592=CARTESIAN_POINT('Ctrl Pts',(-0.244970516690577,0.0749510565005375,
-0.643082713935629));
#50593=CARTESIAN_POINT('Ctrl Pts',(-0.207996747629523,0.150372981653613,
-0.646998177492464));
#50594=CARTESIAN_POINT('Ctrl Pts',(-0.148200952265686,0.195663883798494,
-0.650913641049299));
#50595=CARTESIAN_POINT('Ctrl Pts',(-0.0834526345811506,0.244705956112317,
-0.655153398656294));
#50596=CARTESIAN_POINT('Ctrl Pts',(0.00805468346630517,0.258419173533304,
-0.659393156263289));
#50597=CARTESIAN_POINT('Ctrl Pts',(0.0843346332239721,0.230511490634511,
-0.663632913870285));
#50598=CARTESIAN_POINT('Ctrl Pts',(0.160614582981637,0.20260380773572,-0.66787267147728));
#50599=CARTESIAN_POINT('Ctrl Pts',(0.221667164449512,0.133075224517152,
-0.672112429084275));
#50600=CARTESIAN_POINT('Ctrl Pts',(0.239479577696338,0.053827590898629,
-0.676352186691271));
#50601=CARTESIAN_POINT('Ctrl Pts',(0.257291990943163,-0.0254200427198954,
-0.680591944298266));
#50602=CARTESIAN_POINT('Ctrl Pts',(0.231864235968934,-0.114386726738377,
-0.684831701905261));
#50603=CARTESIAN_POINT('Ctrl Pts',(0.174863347904167,-0.172251813445643,
-0.689071459512257));
#50604=CARTESIAN_POINT('Ctrl Pts',(0.117862459839398,-0.23011690015291,
-0.693311217119252));
#50605=CARTESIAN_POINT('Ctrl Pts',(0.0292884386840905,-0.256880389548962,
-0.697550974726248));
#50606=CARTESIAN_POINT('Ctrl Pts',(-0.0502182336349338,-0.240262370516387,
-0.701790732333243));
#50607=CARTESIAN_POINT('Ctrl Pts',(-0.129724905953956,-0.223644351483812,
-0.706030489940239));
#50608=CARTESIAN_POINT('Ctrl Pts',(-0.200164229436694,-0.163644824022614,
-0.710270247547233));
#50609=CARTESIAN_POINT('Ctrl Pts',(-0.229216478551909,-0.0877934145356514,
-0.714510005154228));
#50610=CARTESIAN_POINT('Ctrl Pts',(-0.239854150245803,-0.0600199231119234,
-0.716062420229084));
#50611=CARTESIAN_POINT('Ctrl Pts',(-0.244943030851271,-0.0301211598958906,
-0.717614835303939));
#50612=CARTESIAN_POINT('Ctrl Pts',(-0.244760954731183,-0.000162685205530727,
-0.719167250378794));
#50613=CARTESIAN_POINT('Ctrl Pts',(-0.244799701406111,-0.000182046177014158,
-0.730732749621206));
#50614=CARTESIAN_POINT('Ctrl Pts',(-0.244993146475634,-0.0283308750298025,
-0.729273528113761));
#50615=CARTESIAN_POINT('Ctrl Pts',(-0.240512310992863,-0.0564200049260635,
-0.727814306606315));
#50616=CARTESIAN_POINT('Ctrl Pts',(-0.231088843712454,-0.0827394660268344,
-0.726355085098869));
#50617=CARTESIAN_POINT('Ctrl Pts',(-0.203709027226386,-0.159210471178991,
-0.722115327491874));
#50618=CARTESIAN_POINT('Ctrl Pts',(-0.134604064186045,-0.220742129669793,
-0.717875569884879));
#50619=CARTESIAN_POINT('Ctrl Pts',(-0.0554814345597428,-0.239101826312468,
-0.713635812277884));
#50620=CARTESIAN_POINT('Ctrl Pts',(0.023641195066559,-0.257461522955143,
-0.709396054670889));
#50621=CARTESIAN_POINT('Ctrl Pts',(0.112781491278821,-0.23264925774969,
-0.705156297063893));
#50622=CARTESIAN_POINT('Ctrl Pts',(0.171039147757949,-0.176049660212677,
-0.700916539456897));
#50623=CARTESIAN_POINT('Ctrl Pts',(0.229296804237077,-0.119450062675664,
-0.696676781849902));
#50624=CARTESIAN_POINT('Ctrl Pts',(0.256671820983071,-0.0310631328070899,
-0.692437024242907));
#50625=CARTESIAN_POINT('Ctrl Pts',(0.24060369934406,0.0485564906960756,
-0.688197266635912));
#50626=CARTESIAN_POINT('Ctrl Pts',(0.224535577705048,0.128176114199242,
-0.683957509028917));
#50627=CARTESIAN_POINT('Ctrl Pts',(0.165024317681031,0.199028431337,-0.679717751421921));
#50628=CARTESIAN_POINT('Ctrl Pts',(0.0893755135749676,0.228604222401896,
-0.675477993814925));
#50629=CARTESIAN_POINT('Ctrl Pts',(0.013726709468904,0.258180013466792,
-0.67123823620793));
#50630=CARTESIAN_POINT('Ctrl Pts',(-0.0780596387192057,0.246479278458826,
-0.666998478600936));
#50631=CARTESIAN_POINT('Ctrl Pts',(-0.14386913473623,0.198870674049778,
-0.66275872099394));
#50632=CARTESIAN_POINT('Ctrl Pts',(-0.206091490235119,0.153857116924535,
-0.658750063869696));
#50633=CARTESIAN_POINT('Ctrl Pts',(-0.245091703074977,0.0767435324240782,
-0.654741406745451));
#50634=CARTESIAN_POINT('Ctrl Pts',(-0.245422021931952,-8.10237852447184E-5,
-0.650732749621206));
#50635=CARTESIAN_POINT('Origin',(0.,0.,-0.775));
#50636=CARTESIAN_POINT('',(-0.245099038793128,0.000222287303026779,-0.559167250378794));
#50637=CARTESIAN_POINT('',(-0.245044311916972,0.000225594359514621,-0.570732749621207));
#50638=CARTESIAN_POINT('',(-0.24505,-3.00099698131059E-17,-0.775));
#50639=CARTESIAN_POINT('Ctrl Pts',(-0.245099038793128,0.000222287303026779,
-0.559167250378794));
#50640=CARTESIAN_POINT('Ctrl Pts',(-0.245260304066475,0.0176033761932229,
-0.560071077353328));
#50641=CARTESIAN_POINT('Ctrl Pts',(-0.243569224089339,0.0349533179170207,
-0.560974904327863));
#50642=CARTESIAN_POINT('Ctrl Pts',(-0.239909555455349,0.0518775758568482,
-0.561878731302397));
#50643=CARTESIAN_POINT('Ctrl Pts',(-0.222742433464957,0.131267496012865,
-0.566118488909392));
#50644=CARTESIAN_POINT('Ctrl Pts',(-0.162257506943935,0.201290458332522,
-0.570358246516388));
#50645=CARTESIAN_POINT('Ctrl Pts',(-0.0862071182953996,0.229817776576942,
-0.574598004123383));
#50646=CARTESIAN_POINT('Ctrl Pts',(-0.0101567296468654,0.258345094821361,
-0.578837761730378));
#50647=CARTESIAN_POINT('Ctrl Pts',(0.0814591211291825,0.245376768990544,
-0.583077519337374));
#50648=CARTESIAN_POINT('Ctrl Pts',(0.146604267229997,0.196863065366569,
-0.587317276944369));
#50649=CARTESIAN_POINT('Ctrl Pts',(0.211749413330811,0.148349361742594,
-0.591557034551365));
#50650=CARTESIAN_POINT('Ctrl Pts',(0.250423854756394,0.0642902803254605,
-0.59579679215836));
#50651=CARTESIAN_POINT('Ctrl Pts',(0.244882569690129,-0.0167452900101996,
-0.600036549765355));
#50652=CARTESIAN_POINT('Ctrl Pts',(0.239341284623863,-0.097780860345862,
-0.60427630737235));
#50653=CARTESIAN_POINT('Ctrl Pts',(0.18958427306575,-0.175792919600049,
-0.608516064979345));
#50654=CARTESIAN_POINT('Ctrl Pts',(0.11844158046912,-0.214987138432845,
-0.612755822586341));
#50655=CARTESIAN_POINT('Ctrl Pts',(0.0472988878724918,-0.254181357265641,
-0.616995580193336));
#50656=CARTESIAN_POINT('Ctrl Pts',(-0.0452294857626519,-0.254557735677044,
-0.621235337800332));
#50657=CARTESIAN_POINT('Ctrl Pts',(-0.116688680112832,-0.215943579689445,
-0.625475095407327));
#50658=CARTESIAN_POINT('Ctrl Pts',(-0.188147874463012,-0.177329423701845,
-0.629714853014322));
#50659=CARTESIAN_POINT('Ctrl Pts',(-0.238537889528229,-0.099724733315242,
-0.633954610621317));
#50660=CARTESIAN_POINT('Ctrl Pts',(-0.244738238400031,-0.0187369245186125,
-0.638194368228313));
#50661=CARTESIAN_POINT('Ctrl Pts',(-0.245212495759632,-0.0125422627094244,
-0.638518662278473));
#50662=CARTESIAN_POINT('Ctrl Pts',(-0.245428219737942,-0.00632780783282481,
-0.638842956328634));
#50663=CARTESIAN_POINT('Ctrl Pts',(-0.245393210572617,-0.000110883529508943,
-0.639167250378794));
#50664=CARTESIAN_POINT('Ctrl Pts',(-0.245422021931952,-8.10237852447184E-5,
-0.650732749621206));
#50665=CARTESIAN_POINT('Ctrl Pts',(-0.245441064929381,-0.00450998627238757,
-0.650501649138455));
#50666=CARTESIAN_POINT('Ctrl Pts',(-0.24533158610744,-0.00893798815586689,
-0.650270548655704));
#50667=CARTESIAN_POINT('Ctrl Pts',(-0.24509062560664,-0.0133588235451446,
-0.650039448172953));
#50668=CARTESIAN_POINT('Ctrl Pts',(-0.240669976614088,-0.0944632429208891,
-0.645799690565958));
#50669=CARTESIAN_POINT('Ctrl Pts',(-0.191996034783046,-0.173155607862247,
-0.641559932958963));
#50670=CARTESIAN_POINT('Ctrl Pts',(-0.121401899903836,-0.213329443880829,
-0.637320175351968));
#50671=CARTESIAN_POINT('Ctrl Pts',(-0.0508077650246259,-0.253503279899411,
-0.633080417744973));
#50672=CARTESIAN_POINT('Ctrl Pts',(0.0417065629027502,-0.255158586995217,
-0.628840660137977));
#50673=CARTESIAN_POINT('Ctrl Pts',(0.113692668157028,-0.217535859421155,
-0.624600902530982));
#50674=CARTESIAN_POINT('Ctrl Pts',(0.185678773411305,-0.179913131847094,
-0.620361144923986));
#50675=CARTESIAN_POINT('Ctrl Pts',(0.237136655992484,-0.103012369603164,
-0.616121387316991));
#50676=CARTESIAN_POINT('Ctrl Pts',(0.244455858570574,-0.0221180048216005,
-0.611881629709996));
#50677=CARTESIAN_POINT('Ctrl Pts',(0.251775061148664,0.0587763599599641,
-0.607641872103));
#50678=CARTESIAN_POINT('Ctrl Pts',(0.214955583723666,0.143664327279164,
-0.603402114496005));
#50679=CARTESIAN_POINT('Ctrl Pts',(0.150891333643671,0.193596689945875,
-0.59916235688901));
#50680=CARTESIAN_POINT('Ctrl Pts',(0.0868270835636758,0.243529052612585,
-0.594922599282015));
#50681=CARTESIAN_POINT('Ctrl Pts',(-0.00448193917131465,0.258505810626804,
-0.590682841675019));
#50682=CARTESIAN_POINT('Ctrl Pts',(-0.0811403498896434,0.231655167321066,
-0.586443084068023));
#50683=CARTESIAN_POINT('Ctrl Pts',(-0.157798760607972,0.204804524015327,
-0.582203326461028));
#50684=CARTESIAN_POINT('Ctrl Pts',(-0.219806559309638,0.13612647938963,
-0.577963568854034));
#50685=CARTESIAN_POINT('Ctrl Pts',(-0.238712663051953,0.057132630128584,
-0.573723811247038));
#50686=CARTESIAN_POINT('Ctrl Pts',(-0.243158618586795,0.0385564525021716,
-0.572726790705094));
#50687=CARTESIAN_POINT('Ctrl Pts',(-0.245221044763826,0.0194098095327841,
-0.571729770163151));
#50688=CARTESIAN_POINT('Ctrl Pts',(-0.245044311916972,0.000225594359514621,
-0.570732749621207));
#50689=CARTESIAN_POINT('Origin',(0.,0.,-0.775));
#50690=CARTESIAN_POINT('',(-0.24464554858441,-3.8505879792117E-6,-0.479167250378794));
#50691=CARTESIAN_POINT('',(-0.244649643429401,-3.34626570719463E-5,-0.490732749621207));
#50692=CARTESIAN_POINT('',(-0.24505,-3.00099698131059E-17,-0.775));
#50693=CARTESIAN_POINT('Ctrl Pts',(-0.244645577937762,-3.85030852002866E-6,
-0.479167250378794));
#50694=CARTESIAN_POINT('Ctrl Pts',(-0.244639821044035,0.0411869810206832,
-0.481299198378023));
#50695=CARTESIAN_POINT('Ctrl Pts',(-0.23479682609857,0.0823803969011494,
-0.483431146377252));
#50696=CARTESIAN_POINT('Ctrl Pts',(-0.21513194374638,0.11817835865959,-0.485563094376481));
#50697=CARTESIAN_POINT('Ctrl Pts',(-0.176024829232561,0.18936896965721,
-0.489802851983476));
#50698=CARTESIAN_POINT('Ctrl Pts',(-0.0980737284097471,0.239221426655701,
-0.494042609590472));
#50699=CARTESIAN_POINT('Ctrl Pts',(-0.0170450010169084,0.244861890901583,
-0.498282367197467));
#50700=CARTESIAN_POINT('Ctrl Pts',(0.0639837263759303,0.250502355147466,
-0.502522124804463));
#50701=CARTESIAN_POINT('Ctrl Pts',(0.148090080338794,0.21193082664074,-0.506761882411458));
#50702=CARTESIAN_POINT('Ctrl Pts',(0.196683481900857,0.146845107589328,
-0.511001640018453));
#50703=CARTESIAN_POINT('Ctrl Pts',(0.245276883462918,0.0817593885379164,
-0.515241397625448));
#50704=CARTESIAN_POINT('Ctrl Pts',(0.25835733262418,-0.00984052105818028,
-0.519481155232444));
#50705=CARTESIAN_POINT('Ctrl Pts',(0.229923117474086,-0.0859257686992934,
-0.523720912839439));
#50706=CARTESIAN_POINT('Ctrl Pts',(0.201488902323992,-0.162011016340406,
-0.527960670446434));
#50707=CARTESIAN_POINT('Ctrl Pts',(0.131540022862543,-0.222581602026536,
-0.53220042805343));
#50708=CARTESIAN_POINT('Ctrl Pts',(0.0521711738374254,-0.239845880298143,
-0.536440185660425));
#50709=CARTESIAN_POINT('Ctrl Pts',(-0.0271976751876943,-0.257110158569751,
-0.54067994326742));
#50710=CARTESIAN_POINT('Ctrl Pts',(-0.115986493776483,-0.231068129426834,
-0.544919700874415));
#50711=CARTESIAN_POINT('Ctrl Pts',(-0.173456244340995,-0.173668675859187,
-0.549159458481411));
#50712=CARTESIAN_POINT('Ctrl Pts',(-0.218674655184041,-0.128505576174691,
-0.552495389113872));
#50713=CARTESIAN_POINT('Ctrl Pts',(-0.244503825571495,-0.0639294900702973,
-0.555831319746333));
#50714=CARTESIAN_POINT('Ctrl Pts',(-0.245099038793128,0.000222287303026779,
-0.559167250378794));
#50715=CARTESIAN_POINT('Ctrl Pts',(-0.245044311916972,0.000225594359514621,
-0.570732749621207));
#50716=CARTESIAN_POINT('Ctrl Pts',(-0.244469501139266,-0.0621696753357292,
-0.567490012556155));
#50717=CARTESIAN_POINT('Ctrl Pts',(-0.220208228315207,-0.124962394507208,
-0.564247275491103));
#50718=CARTESIAN_POINT('Ctrl Pts',(-0.17722756994711,-0.169818318733306,
-0.561004538426051));
#50719=CARTESIAN_POINT('Ctrl Pts',(-0.121031964316992,-0.228465764437753,
-0.556764780819056));
#50720=CARTESIAN_POINT('Ctrl Pts',(-0.0328363442737951,-0.256451001950254,
-0.552525023212061));
#50721=CARTESIAN_POINT('Ctrl Pts',(0.0468924303104948,-0.240933544585099,
-0.548285265605066));
#50722=CARTESIAN_POINT('Ctrl Pts',(0.126621204894785,-0.225416087219944,
-0.544045507998071));
#50723=CARTESIAN_POINT('Ctrl Pts',(0.197883134020166,-0.166395934977131,
-0.539805750391075));
#50724=CARTESIAN_POINT('Ctrl Pts',(0.227981055415858,-0.0909533468226233,
-0.535565992784079));
#50725=CARTESIAN_POINT('Ctrl Pts',(0.258078976811549,-0.0155107586681155,
-0.531326235177084));
#50726=CARTESIAN_POINT('Ctrl Pts',(0.247012890477551,0.0763542653980887,
-0.527086477570089));
#50727=CARTESIAN_POINT('Ctrl Pts',(0.199860256777428,0.142491230213038,
-0.522846719963094));
#50728=CARTESIAN_POINT('Ctrl Pts',(0.152707623077304,0.208628195027989,
-0.518606962356099));
#50729=CARTESIAN_POINT('Ctrl Pts',(0.0694684420110575,0.249037100591685,
-0.514367204749104));
#50730=CARTESIAN_POINT('Ctrl Pts',(-0.0116645930152598,0.245177099657682,
-0.510127447142108));
#50731=CARTESIAN_POINT('Ctrl Pts',(-0.092797628041576,0.241317098723679,
-0.505887689535113));
#50732=CARTESIAN_POINT('Ctrl Pts',(-0.171824517027962,0.193188191291977,
-0.501647931928117));
#50733=CARTESIAN_POINT('Ctrl Pts',(-0.212485295577484,0.122873398626858,
-0.497408174321122));
#50734=CARTESIAN_POINT('Ctrl Pts',(-0.233825192069005,0.0859702587750484,
-0.495183032754483));
#50735=CARTESIAN_POINT('Ctrl Pts',(-0.244597375570812,0.0429561510690604,
-0.492957891187845));
#50736=CARTESIAN_POINT('Ctrl Pts',(-0.244649643429401,-3.34626570719463E-5,
-0.490732749621207));
#50737=CARTESIAN_POINT('Origin',(0.,0.,-0.775));
#50738=CARTESIAN_POINT('',(-0.245113213433533,-0.000220732632699366,-0.399167250378794));
#50739=CARTESIAN_POINT('',(-0.245167474403332,-0.000212043108657725,-0.410732749621206));
#50740=CARTESIAN_POINT('',(-0.24505,-3.00099698131059E-17,-0.775));
#50741=CARTESIAN_POINT('Ctrl Pts',(-0.245113213433533,-0.000220732632699366,
-0.399167250378794));
#50742=CARTESIAN_POINT('Ctrl Pts',(-0.2445143688444,0.0643856472039739,
-0.402527319402718));
#50743=CARTESIAN_POINT('Ctrl Pts',(-0.21826929847075,0.129422269040789,
-0.405887388426641));
#50744=CARTESIAN_POINT('Ctrl Pts',(-0.172465708082888,0.174652389652183,
-0.409247457450565));
#50745=CARTESIAN_POINT('Ctrl Pts',(-0.114670430845441,0.23172405888341,
-0.41348721505756));
#50746=CARTESIAN_POINT('Ctrl Pts',(-0.0257349357162201,0.257260685412779,
-0.417726972664556));
#50747=CARTESIAN_POINT('Ctrl Pts',(0.0535344400129061,0.239545280496294,
-0.421966730271551));
#50748=CARTESIAN_POINT('Ctrl Pts',(0.132803815742034,0.221829875579809,
-0.426206487878547));
#50749=CARTESIAN_POINT('Ctrl Pts',(0.202407072071065,0.160862439217467,
-0.430446245485542));
#50750=CARTESIAN_POINT('Ctrl Pts',(0.230408096763762,0.0846167041501249,
-0.434686003092537));
#50751=CARTESIAN_POINT('Ctrl Pts',(0.258409121456458,0.00837096908278148,
-0.438925760699532));
#50752=CARTESIAN_POINT('Ctrl Pts',(0.244807914512817,-0.0831530646895631,
-0.443165518306528));
#50753=CARTESIAN_POINT('Ctrl Pts',(0.195845127511443,-0.147961358825947,
-0.447405275913524));
#50754=CARTESIAN_POINT('Ctrl Pts',(0.14688234051007,-0.212769652962328,
-0.451645033520519));
#50755=CARTESIAN_POINT('Ctrl Pts',(0.0625579734509672,-0.250862207462751,
-0.455884791127514));
#50756=CARTESIAN_POINT('Ctrl Pts',(-0.0184373635888685,-0.24476098810769,
-0.460124548734509));
#50757=CARTESIAN_POINT('Ctrl Pts',(-0.0994327006287077,-0.238659768752629,
-0.464364306341504));
#50758=CARTESIAN_POINT('Ctrl Pts',(-0.177099007649279,-0.18836477554208,
-0.4686040639485));
#50759=CARTESIAN_POINT('Ctrl Pts',(-0.215800597057152,-0.116952896438431,
-0.472843821555495));
#50760=CARTESIAN_POINT('Ctrl Pts',(-0.235041221062436,-0.0814502430237733,
-0.474951631163261));
#50761=CARTESIAN_POINT('Ctrl Pts',(-0.244651269650652,-0.0407283098445718,
-0.477059440771028));
#50762=CARTESIAN_POINT('Ctrl Pts',(-0.244645577937762,-3.85030852002866E-6,
-0.479167250378794));
#50763=CARTESIAN_POINT('Ctrl Pts',(-0.244649643429401,-3.34626570719463E-5,
-0.490732749621207));
#50764=CARTESIAN_POINT('Ctrl Pts',(-0.244696966111197,-0.038955734695813,
-0.48871813358085));
#50765=CARTESIAN_POINT('Ctrl Pts',(-0.235956883659052,-0.0778579283560022,
-0.486703517540493));
#50766=CARTESIAN_POINT('Ctrl Pts',(-0.218316435692479,-0.112186482400046,
-0.484688901500136));
#50767=CARTESIAN_POINT('Ctrl Pts',(-0.181192129145293,-0.184430892863294,
-0.480449143893141));
#50768=CARTESIAN_POINT('Ctrl Pts',(-0.104648847938264,-0.236419035891254,
-0.476209386286145));
#50769=CARTESIAN_POINT('Ctrl Pts',(-0.023807000921954,-0.2442971543712,
-0.47196962867915));
#50770=CARTESIAN_POINT('Ctrl Pts',(0.0570348460943559,-0.252175272851145,
-0.467729871072154));
#50771=CARTESIAN_POINT('Ctrl Pts',(0.142175258919946,-0.215943366783077,
-0.463490113465159));
#50772=CARTESIAN_POINT('Ctrl Pts',(0.192549200611132,-0.152225747726141,
-0.459250355858164));
#50773=CARTESIAN_POINT('Ctrl Pts',(0.242923142302319,-0.0885081286692047,
-0.455010598251169));
#50774=CARTESIAN_POINT('Ctrl Pts',(0.258530612859102,0.00269520337659913,
-0.450770840644173));
#50775=CARTESIAN_POINT('Ctrl Pts',(0.232210425323849,0.0795373578746301,
-0.446531083037178));
#50776=CARTESIAN_POINT('Ctrl Pts',(0.205890237788597,0.156379512372661,
-0.442291325430183));
#50777=CARTESIAN_POINT('Ctrl Pts',(0.137642392161309,0.218860489322919,
-0.438051567823187));
#50778=CARTESIAN_POINT('Ctrl Pts',(0.0587810966101972,0.238312097066141,
-0.433811810216192));
#50779=CARTESIAN_POINT('Ctrl Pts',(-0.0200801989409146,0.257763704809364,
-0.429572052609197));
#50780=CARTESIAN_POINT('Ctrl Pts',(-0.10955494441585,0.23418594334555,-0.425332295002201));
#50781=CARTESIAN_POINT('Ctrl Pts',(-0.168589377899256,0.178397013950162,
-0.421092537395206));
#50782=CARTESIAN_POINT('Ctrl Pts',(-0.216672645775806,0.132957193859089,
-0.417639274803873));
#50783=CARTESIAN_POINT('Ctrl Pts',(-0.244561732339873,0.0661484020676576,
-0.414186012212539));
#50784=CARTESIAN_POINT('Ctrl Pts',(-0.245167474403332,-0.000212043108657725,
-0.410732749621206));
#50785=CARTESIAN_POINT('Origin',(0.,0.,-0.775));
#50786=CARTESIAN_POINT('',(-0.245384525130581,0.000118217037109843,-0.319167250378794));
#50787=CARTESIAN_POINT('',(-0.245346855243246,0.000144723277665203,-0.330732749621206));
#50788=CARTESIAN_POINT('',(-0.24505,-3.00099698131059E-17,-0.775));
#50789=CARTESIAN_POINT('Ctrl Pts',(-0.245384525130581,0.000118217037109843,
-0.319167250378794));
#50790=CARTESIAN_POINT('Ctrl Pts',(-0.245424204817052,0.00679851531508335,
-0.319515682820417));
#50791=CARTESIAN_POINT('Ctrl Pts',(-0.245175118904715,0.013475809046111,
-0.31986411526204));
#50792=CARTESIAN_POINT('Ctrl Pts',(-0.244627714853342,0.0201285564437554,
-0.320212547703663));
#50793=CARTESIAN_POINT('Ctrl Pts',(-0.237966852621071,0.1010797912231,-0.324452305310658));
#50794=CARTESIAN_POINT('Ctrl Pts',(-0.18713628029174,0.17839663610918,-0.328692062917654));
#50795=CARTESIAN_POINT('Ctrl Pts',(-0.115458625868584,0.21660374741823,
-0.332931820524649));
#50796=CARTESIAN_POINT('Ctrl Pts',(-0.0437809714454274,0.254810858727282,
-0.337171578131644));
#50797=CARTESIAN_POINT('Ctrl Pts',(0.0487437650715545,0.2539082364593,-0.34141133573864));
#50798=CARTESIAN_POINT('Ctrl Pts',(0.119662392121641,0.214310031467542,
-0.345651093345635));
#50799=CARTESIAN_POINT('Ctrl Pts',(0.190581019171727,0.174711826475785,
-0.349890850952631));
#50800=CARTESIAN_POINT('Ctrl Pts',(0.239893536754919,0.0964180387602521,
-0.354130608559626));
#50801=CARTESIAN_POINT('Ctrl Pts',(0.24497384693941,0.0153522633190858,
-0.358370366166621));
#50802=CARTESIAN_POINT('Ctrl Pts',(0.250054157123901,-0.0657135121220805,
-0.362610123773617));
#50803=CARTESIAN_POINT('Ctrl Pts',(0.210902259909693,-0.14955127528888,
-0.366849881380612));
#50804=CARTESIAN_POINT('Ctrl Pts',(0.145482248480625,-0.197693684911225,
-0.371089638987607));
#50805=CARTESIAN_POINT('Ctrl Pts',(0.0800622370515574,-0.245836094533568,
-0.375329396594603));
#50806=CARTESIAN_POINT('Ctrl Pts',(-0.0116258885923681,-0.258283150611457,
-0.379569154201598));
#50807=CARTESIAN_POINT('Ctrl Pts',(-0.0875127997102276,-0.229323761443049,
-0.383808911808593));
#50808=CARTESIAN_POINT('Ctrl Pts',(-0.163399710828089,-0.20036437227464,
-0.388048669415588));
#50809=CARTESIAN_POINT('Ctrl Pts',(-0.223485407419884,-0.129998537859931,
-0.392288427022584));
#50810=CARTESIAN_POINT('Ctrl Pts',(-0.240200726042946,-0.0505122646860321,
-0.396528184629579));
#50811=CARTESIAN_POINT('Ctrl Pts',(-0.243668913689063,-0.0340200088772053,
-0.397407873212651));
#50812=CARTESIAN_POINT('Ctrl Pts',(-0.245269994959254,-0.01713511573949,
-0.398287561795722));
#50813=CARTESIAN_POINT('Ctrl Pts',(-0.245113213433533,-0.000220732632699366,
-0.399167250378794));
#50814=CARTESIAN_POINT('Ctrl Pts',(-0.245167474403332,-0.000212043108657725,
-0.410732749621206));
#50815=CARTESIAN_POINT('Ctrl Pts',(-0.24530543469482,-0.0153259123809456,
-0.409946254605544));
#50816=CARTESIAN_POINT('Ctrl Pts',(-0.244028154161137,-0.0304165250311018,
-0.409159759589882));
#50817=CARTESIAN_POINT('Ctrl Pts',(-0.241251881014642,-0.0452261299872512,
-0.40837326457422));
#50818=CARTESIAN_POINT('Ctrl Pts',(-0.226285829154746,-0.125060247202309,
-0.404133506967224));
#50819=CARTESIAN_POINT('Ctrl Pts',(-0.167759603943079,-0.196728384305462,
-0.399893749360229));
#50820=CARTESIAN_POINT('Ctrl Pts',(-0.092526835449539,-0.227346998327305,
-0.395653991753234));
#50821=CARTESIAN_POINT('Ctrl Pts',(-0.0172940669560004,-0.257965612349148,
-0.391414234146239));
#50822=CARTESIAN_POINT('Ctrl Pts',(0.0746452448194102,-0.247534703289683,
-0.387174476539243));
#50823=CARTESIAN_POINT('Ctrl Pts',(0.141106519229503,-0.200840292665299,
-0.382934718932248));
#50824=CARTESIAN_POINT('Ctrl Pts',(0.207567793639597,-0.154145882040914,
-0.378694961325253));
#50825=CARTESIAN_POINT('Ctrl Pts',(0.248551030684372,-0.0711879698516079,
-0.374455203718257));
#50826=CARTESIAN_POINT('Ctrl Pts',(0.245251862192355,0.00996980529647849,
-0.370215446111262));
#50827=CARTESIAN_POINT('Ctrl Pts',(0.241952693700338,0.0911275804445649,
-0.365975688504267));
#50828=CARTESIAN_POINT('Ctrl Pts',(0.194371119671528,0.170485218551432,
-0.361735930897271));
#50829=CARTESIAN_POINT('Ctrl Pts',(0.124339027986658,0.211630997365796,
-0.357496173290276));
#50830=CARTESIAN_POINT('Ctrl Pts',(0.054306936301789,0.25277677618016,-0.353256415683281));
#50831=CARTESIAN_POINT('Ctrl Pts',(-0.0381756730391405,0.255710695702023,
-0.349016658076286));
#50832=CARTESIAN_POINT('Ctrl Pts',(-0.110674937768999,0.219086583518454,
-0.34477690046929));
#50833=CARTESIAN_POINT('Ctrl Pts',(-0.183174202498859,0.182462471334884,
-0.340537142862295));
#50834=CARTESIAN_POINT('Ctrl Pts',(-0.235690122617646,0.106280327445879,
-0.3362973852553));
#50835=CARTESIAN_POINT('Ctrl Pts',(-0.244126780684619,0.0254948598165568,
-0.332057627648304));
#50836=CARTESIAN_POINT('Ctrl Pts',(-0.245005568572291,0.0170800005335381,
-0.331616001639271));
#50837=CARTESIAN_POINT('Ctrl Pts',(-0.245406099229541,0.00861519547646839,
-0.331174375630239));
#50838=CARTESIAN_POINT('Ctrl Pts',(-0.245346855243246,0.000144723277665203,
-0.330732749621206));
#50839=CARTESIAN_POINT('Origin',(0.,0.,-0.775));
#50840=CARTESIAN_POINT('',(-0.244751705071012,0.000157197749167753,-0.239167250378794));
#50841=CARTESIAN_POINT('',(-0.244719249417263,0.000134367256465015,-0.250732749621206));
#50842=CARTESIAN_POINT('',(-0.24505,-3.00099698131059E-17,-0.775));
#50843=CARTESIAN_POINT('Ctrl Pts',(-0.244751705071012,0.000157197749167753,
-0.239167250378794));
#50844=CARTESIAN_POINT('Ctrl Pts',(-0.244929957152803,0.030584378658343,
-0.240743803845112));
#50845=CARTESIAN_POINT('Ctrl Pts',(-0.239676767767007,0.0609522085494251,
-0.242320357311429));
#50846=CARTESIAN_POINT('Ctrl Pts',(-0.228713449599398,0.0890956496980255,
-0.243896910777747));
#50847=CARTESIAN_POINT('Ctrl Pts',(-0.199230268348596,0.164780598699778,
-0.248136668384742));
#50848=CARTESIAN_POINT('Ctrl Pts',(-0.128450843241183,0.224378537504145,
-0.252376425991738));
#50849=CARTESIAN_POINT('Ctrl Pts',(-0.0488509435112058,0.240544098374202,
-0.256616183598733));
#50850=CARTESIAN_POINT('Ctrl Pts',(0.0307489562187699,0.25670965924426,
-0.260855941205729));
#50851=CARTESIAN_POINT('Ctrl Pts',(0.119169330571309,0.229442842180009,
-0.265095698812724));
#50852=CARTESIAN_POINT('Ctrl Pts',(0.175840192674927,0.171254501831632,
-0.269335456419719));
#50853=CARTESIAN_POINT('Ctrl Pts',(0.232511054778548,0.113066161483252,
-0.273575214026715));
#50854=CARTESIAN_POINT('Ctrl Pts',(0.257432404633245,0.0239562978507422,
-0.27781497163371));
#50855=CARTESIAN_POINT('Ctrl Pts',(0.239169562812728,-0.0551887468503754,
-0.282054729240705));
#50856=CARTESIAN_POINT('Ctrl Pts',(0.220906720992213,-0.134333791551488,
-0.286294486847701));
#50857=CARTESIAN_POINT('Ctrl Pts',(0.15945968749649,-0.203514017321211,
-0.290534244454696));
#50858=CARTESIAN_POINT('Ctrl Pts',(0.0830222481891644,-0.230987410971053,
-0.294774002061691));
#50859=CARTESIAN_POINT('Ctrl Pts',(0.00658480888183648,-0.258460804620896,
-0.299013759668687));
#50860=CARTESIAN_POINT('Ctrl Pts',(-0.0848430362370954,-0.244227366150856,
-0.303253517275682));
#50861=CARTESIAN_POINT('Ctrl Pts',(-0.149311382728958,-0.19481783457953,
-0.307493274882677));
#50862=CARTESIAN_POINT('Ctrl Pts',(-0.208481581199691,-0.149468885079323,
-0.311384600048049));
#50863=CARTESIAN_POINT('Ctrl Pts',(-0.244941378786922,-0.074487961079283,
-0.315275925213421));
#50864=CARTESIAN_POINT('Ctrl Pts',(-0.245384525130581,0.000118217037109843,
-0.319167250378794));
#50865=CARTESIAN_POINT('Ctrl Pts',(-0.245346855243246,0.000144723277665203,
-0.330732749621206));
#50866=CARTESIAN_POINT('Ctrl Pts',(-0.244837337117652,-0.072704174771635,
-0.326934618023243));
#50867=CARTESIAN_POINT('Ctrl Pts',(-0.210320237519882,-0.145972247272856,
-0.323136486425281));
#50868=CARTESIAN_POINT('Ctrl Pts',(-0.153552890361856,-0.191492513662049,
-0.319338354827318));
#50869=CARTESIAN_POINT('Ctrl Pts',(-0.0901849459569572,-0.242305628141694,
-0.315098597220323));
#50870=CARTESIAN_POINT('Ctrl Pts',(0.000908338867999472,-0.258543065731344,
-0.310858839613328));
#50871=CARTESIAN_POINT('Ctrl Pts',(0.0779305665684941,-0.232754591208473,
-0.306619082006332));
#50872=CARTESIAN_POINT('Ctrl Pts',(0.154952794268988,-0.206966116685603,
-0.302379324399337));
#50873=CARTESIAN_POINT('Ctrl Pts',(0.21790396484502,-0.139151730050211,
-0.298139566792341));
#50874=CARTESIAN_POINT('Ctrl Pts',(0.237900147459264,-0.0604267552403789,
-0.293899809185346));
#50875=CARTESIAN_POINT('Ctrl Pts',(0.257896330073507,0.0182982195694519,
-0.289660051578351));
#50876=CARTESIAN_POINT('Ctrl Pts',(0.234937524725965,0.107933782553724,
-0.285420293971356));
#50877=CARTESIAN_POINT('Ctrl Pts',(0.179557936417182,0.167352383919392,
-0.281180536364361));
#50878=CARTESIAN_POINT('Ctrl Pts',(0.124178348108397,0.226770985285061,
-0.276940778757365));
#50879=CARTESIAN_POINT('Ctrl Pts',(0.0363779768383712,0.255972625032124,
-0.27270102115037));
#50880=CARTESIAN_POINT('Ctrl Pts',(-0.0435576694298078,0.241558693502635,
-0.268461263543374));
#50881=CARTESIAN_POINT('Ctrl Pts',(-0.123493315697988,0.227144761973145,
-0.264221505936379));
#50882=CARTESIAN_POINT('Ctrl Pts',(-0.19556423696432,0.169115259167102,
-0.259981748329384));
#50883=CARTESIAN_POINT('Ctrl Pts',(-0.226702081217119,0.0940959041489634,
-0.255741990722389));
#50884=CARTESIAN_POINT('Ctrl Pts',(-0.238965122621183,0.0645509732531478,
-0.254072243688661));
#50885=CARTESIAN_POINT('Ctrl Pts',(-0.244879334034295,0.0323708707275442,
-0.252402496654933));
#50886=CARTESIAN_POINT('Ctrl Pts',(-0.244719249417263,0.000134367256465015,
-0.250732749621206));
#50887=CARTESIAN_POINT('Origin',(0.,0.,-0.775));
#50888=CARTESIAN_POINT('',(-0.244810649818844,-0.000186483096579593,-0.159167250378794));
#50889=CARTESIAN_POINT('',(-0.244854727503173,-0.000201854228764521,-0.170732749621206));
#50890=CARTESIAN_POINT('',(-0.24505,-3.00099698131059E-17,-0.775));
#50891=CARTESIAN_POINT('Ctrl Pts',(-0.244810649818844,-0.000186483096579593,
-0.159167250378794));
#50892=CARTESIAN_POINT('Ctrl Pts',(-0.244428481934693,0.0539105290607768,
-0.161971924869806));
#50893=CARTESIAN_POINT('Ctrl Pts',(-0.226760449543787,0.108234228796465,
-0.164776599360819));
#50894=CARTESIAN_POINT('Ctrl Pts',(-0.193781160300922,0.150654238495037,
-0.167581273851832));
#50895=CARTESIAN_POINT('Ctrl Pts',(-0.143927177997881,0.214779526254686,
-0.171821031458827));
#50896=CARTESIAN_POINT('Ctrl Pts',(-0.0590844826091137,0.251702945519997,
-0.176060789065822));
#50897=CARTESIAN_POINT('Ctrl Pts',(0.0218187482607599,0.244482775158905,
-0.180300546672818));
#50898=CARTESIAN_POINT('Ctrl Pts',(0.102721979130632,0.237262604797812,
-0.184540304279813));
#50899=CARTESIAN_POINT('Ctrl Pts',(0.179685745481613,0.185898844810319,
-0.188780061886808));
#50900=CARTESIAN_POINT('Ctrl Pts',(0.217396571892036,0.113958830238838,
-0.193019819493804));
#50901=CARTESIAN_POINT('Ctrl Pts',(0.25510739830246,0.0420188156673544,
-0.197259577100799));
#50902=CARTESIAN_POINT('Ctrl Pts',(0.253565284772325,-0.050497453488115,
-0.201499334707794));
#50903=CARTESIAN_POINT('Ctrl Pts',(0.213477871231587,-0.121140704416826,
-0.20573909231479));
#50904=CARTESIAN_POINT('Ctrl Pts',(0.17339045769085,-0.191783955345535,
-0.209978849921785));
#50905=CARTESIAN_POINT('Ctrl Pts',(0.0947577441395111,-0.240554188047485,
-0.21421860752878));
#50906=CARTESIAN_POINT('Ctrl Pts',(0.0136587979927169,-0.245074103890555,
-0.218458365135775));
#50907=CARTESIAN_POINT('Ctrl Pts',(-0.0674401481540807,-0.249594019733626,
-0.222698122742771));
#50908=CARTESIAN_POINT('Ctrl Pts',(-0.151005326896335,-0.209863618717812,
-0.226937880349766));
#50909=CARTESIAN_POINT('Ctrl Pts',(-0.198694447570365,-0.144112438610335,
-0.231177637956762));
#50910=CARTESIAN_POINT('Ctrl Pts',(-0.228650373219223,-0.102810828624959,
-0.233840842097439));
#50911=CARTESIAN_POINT('Ctrl Pts',(-0.244450591475787,-0.051242133715127,
-0.236504046238116));
#50912=CARTESIAN_POINT('Ctrl Pts',(-0.244751705071012,0.000157197749167753,
-0.239167250378794));
#50913=CARTESIAN_POINT('Ctrl Pts',(-0.244719249417263,0.000134367256465015,
-0.250732749621206));
#50914=CARTESIAN_POINT('Ctrl Pts',(-0.244472853316488,-0.0494828221095842,
-0.248162739047938));
#50915=CARTESIAN_POINT('Ctrl Pts',(-0.229836337324464,-0.0992336263609378,
-0.24559272847467));
#50916=CARTESIAN_POINT('Ctrl Pts',(-0.201810735292949,-0.139715067653531,
-0.243022717901403));
#50917=CARTESIAN_POINT('Ctrl Pts',(-0.155576777876713,-0.20649747720766,
-0.238782960294407));
#50918=CARTESIAN_POINT('Ctrl Pts',(-0.0729040958049717,-0.248053089085685,
-0.234543202687412));
#50919=CARTESIAN_POINT('Ctrl Pts',(0.00827454209456518,-0.245314910166111,
-0.230303445080417));
#50920=CARTESIAN_POINT('Ctrl Pts',(0.0894531799941032,-0.242576731246538,
-0.226063687473421));
#50921=CARTESIAN_POINT('Ctrl Pts',(0.169137773721435,-0.195544761529366,
-0.221823929866426));
#50922=CARTESIAN_POINT('Ctrl Pts',(0.210766588624511,-0.125798716970005,
-0.217584172259431));
#50923=CARTESIAN_POINT('Ctrl Pts',(0.252395403527586,-0.0560526724106442,
-0.213344414652435));
#50924=CARTESIAN_POINT('Ctrl Pts',(0.255968439606403,0.0364074469909048,
-0.20910465704544));
#50925=CARTESIAN_POINT('Ctrl Pts',(0.219846268834206,0.109158104554032,
-0.204864899438444));
#50926=CARTESIAN_POINT('Ctrl Pts',(0.183724098062009,0.181908762117159,
-0.200625141831449));
#50927=CARTESIAN_POINT('Ctrl Pts',(0.107906720438797,0.234949957841866,
-0.196385384224454));
#50928=CARTESIAN_POINT('Ctrl Pts',(0.0271814956909134,0.243944749294114,
-0.192145626617459));
#50929=CARTESIAN_POINT('Ctrl Pts',(-0.0535437290569703,0.252939540746362,
-0.187905869010463));
#50930=CARTESIAN_POINT('Ctrl Pts',(-0.139176800929527,0.217887927926151,
-0.183666111403468));
#50931=CARTESIAN_POINT('Ctrl Pts',(-0.19042666968436,0.154872691210361,
-0.179426353796473));
#50932=CARTESIAN_POINT('Ctrl Pts',(-0.225455879235849,0.111801870045655,
-0.17652848573805));
#50933=CARTESIAN_POINT('Ctrl Pts',(-0.244422279888803,0.0556672762822381,
-0.173630617679628));
#50934=CARTESIAN_POINT('Ctrl Pts',(-0.244854727503173,-0.000201854228764521,
-0.170732749621206));
#50935=CARTESIAN_POINT('Origin',(0.,0.,-0.775));
#50936=CARTESIAN_POINT('',(-0.245435813781494,-6.93175206961383E-5,-0.0791672503787938));
#50937=CARTESIAN_POINT('',(-0.24544712988196,-4.00287140078511E-5,-0.0907327496212059));
#50938=CARTESIAN_POINT('',(-0.24505,-3.00099698131059E-17,-0.775));
#50939=CARTESIAN_POINT('Ctrl Pts',(-0.245435813781494,-6.93175206961383E-5,
-0.0791672503787938));
#50940=CARTESIAN_POINT('Ctrl Pts',(-0.245137074140361,0.0772146059016804,
-0.0832000458945011));
#50941=CARTESIAN_POINT('Ctrl Pts',(-0.205588735409901,0.154757573364138,
-0.0872328414102084));
#50942=CARTESIAN_POINT('Ctrl Pts',(-0.142732132519899,0.199683998895668,
-0.0912656369259157));
#50943=CARTESIAN_POINT('Ctrl Pts',(-0.0766497439597067,0.246916037728415,
-0.095505394532911));
#50944=CARTESIAN_POINT('Ctrl Pts',(0.0151946451133084,0.258097885770481,
-0.0997451521399064));
#50945=CARTESIAN_POINT('Ctrl Pts',(0.0906723482987466,0.22809311535553,
-0.103984909746902));
#50946=CARTESIAN_POINT('Ctrl Pts',(0.166150051484185,0.198088344940579,
-0.108224667353897));
#50947=CARTESIAN_POINT('Ctrl Pts',(0.225261068782046,0.126896956068611,
-0.112464424960892));
#50948=CARTESIAN_POINT('Ctrl Pts',(0.240876975049947,0.0471868152081749,
-0.116704182567888));
#50949=CARTESIAN_POINT('Ctrl Pts',(0.256492881317849,-0.0325233256522602,
-0.120943940174883));
#50950=CARTESIAN_POINT('Ctrl Pts',(0.228613676555791,-0.120752218501163,
-0.125183697781878));
#50951=CARTESIAN_POINT('Ctrl Pts',(0.170034593344665,-0.17701934772879,
-0.129423455388874));
#50952=CARTESIAN_POINT('Ctrl Pts',(0.111455510133537,-0.233286476956419,
-0.133663212995869));
#50953=CARTESIAN_POINT('Ctrl Pts',(0.0221765484733384,-0.25759184256277,
-0.137902970602864));
#50954=CARTESIAN_POINT('Ctrl Pts',(-0.0568401436653837,-0.238782550966523,
-0.14214272820986));
#50955=CARTESIAN_POINT('Ctrl Pts',(-0.135856835804105,-0.219973259370277,
-0.146382485816855));
#50956=CARTESIAN_POINT('Ctrl Pts',(-0.20461125842135,-0.158049310571434,
-0.15062224342385));
#50957=CARTESIAN_POINT('Ctrl Pts',(-0.231555835121315,-0.0814237580450181,
-0.154862001030846));
#50958=CARTESIAN_POINT('Ctrl Pts',(-0.240676098748089,-0.0554873609967367,
-0.156297084146828));
#50959=CARTESIAN_POINT('Ctrl Pts',(-0.245006195747533,-0.0278665967856731,
-0.157732167262811));
#50960=CARTESIAN_POINT('Ctrl Pts',(-0.244810649818844,-0.000186483096579593,
-0.159167250378794));
#50961=CARTESIAN_POINT('Ctrl Pts',(-0.244854727503173,-0.000201854228764521,
-0.170732749621206));
#50962=CARTESIAN_POINT('Ctrl Pts',(-0.245054977108168,-0.0260726671191914,
-0.169390860072633));
#50963=CARTESIAN_POINT('Ctrl Pts',(-0.241281075540797,-0.0518865579329514,
-0.16804897052406));
#50964=CARTESIAN_POINT('Ctrl Pts',(-0.233287657827869,-0.0763200394868092,
-0.166707080975487));
#50965=CARTESIAN_POINT('Ctrl Pts',(-0.208032111579436,-0.15351867285682,
-0.162467323368491));
#50966=CARTESIAN_POINT('Ctrl Pts',(-0.140654353445459,-0.216937078985472,
-0.158227565761496));
#50967=CARTESIAN_POINT('Ctrl Pts',(-0.0620694914948961,-0.237476859134449,
-0.153987808154501));
#50968=CARTESIAN_POINT('Ctrl Pts',(0.0165153704556672,-0.258016639283427,
-0.149748050547505));
#50969=CARTESIAN_POINT('Ctrl Pts',(0.106307336222817,-0.235677793452729,
-0.14550829294051));
#50970=CARTESIAN_POINT('Ctrl Pts',(0.166107327439438,-0.180710233822531,
-0.141268535333515));
#50971=CARTESIAN_POINT('Ctrl Pts',(0.225907318656059,-0.125742674192334,
-0.137028777726519));
#50972=CARTESIAN_POINT('Ctrl Pts',(0.25571533532215,-0.038146400762637,
-0.132789020119524));
#50973=CARTESIAN_POINT('Ctrl Pts',(0.241854097822414,0.0418870367285358,
-0.128549262512529));
#50974=CARTESIAN_POINT('Ctrl Pts',(0.227992860322678,0.121920474219708,
-0.124309504905533));
#50975=CARTESIAN_POINT('Ctrl Pts',(0.170462368657113,0.194391075772358,
-0.120069747298538));
#50976=CARTESIAN_POINT('Ctrl Pts',(0.0956602294151765,0.226046509466257,
-0.115829989691543));
#50977=CARTESIAN_POINT('Ctrl Pts',(0.0208580901732384,0.257701943160157,
-0.111590232084547));
#50978=CARTESIAN_POINT('Ctrl Pts',(-0.0712156966450689,0.248542208995308,
-0.107350474477552));
#50979=CARTESIAN_POINT('Ctrl Pts',(-0.138316468287019,0.202771205622553,
-0.103110716870557));
#50980=CARTESIAN_POINT('Ctrl Pts',(-0.2036166757344,0.158228409136335,-0.0989847277874397));
#50981=CARTESIAN_POINT('Ctrl Pts',(-0.245266124651116,0.0790128155760584,
-0.0948587387043228));
#50982=CARTESIAN_POINT('Ctrl Pts',(-0.24544712988196,-4.00287140078511E-5,
-0.0907327496212059));
#50983=CARTESIAN_POINT('Origin',(0.,0.,-1.69285451186048));
#50984=CARTESIAN_POINT('',(-0.19978905918818,-5.64256782074264E-5,-0.052854511860476));
#50985=CARTESIAN_POINT('',(-0.199405777330601,0.000173947029632089,-0.0370454881395214));
#50986=CARTESIAN_POINT('',(-0.199475,-2.40257419738789E-14,-1.69285451186048));
#50987=CARTESIAN_POINT('',(0.197117919843508,-0.0326679626569813,-0.0149499999999996));
#50988=CARTESIAN_POINT('Ctrl Pts',(-0.19978905918818,-5.64256782074292E-5,
-0.0528545118604759));
#50989=CARTESIAN_POINT('Ctrl Pts',(-0.199801539091601,-0.0032849757852362,
-0.0526475497691882));
#50990=CARTESIAN_POINT('Ctrl Pts',(-0.198261725162247,-0.0726406134626104,
-0.0482008300709051));
#50991=CARTESIAN_POINT('Ctrl Pts',(-0.117789880017489,-0.204361235882386,
-0.0395143527656268));
#50992=CARTESIAN_POINT('Ctrl Pts',(0.102816622150766,-0.209511115609609,
-0.0270864775700892));
#50993=CARTESIAN_POINT('Ctrl Pts',(0.186733138685136,-0.0934018186338016,
-0.0188983599815467));
#50994=CARTESIAN_POINT('Ctrl Pts',(0.197120359334095,-0.0326678654691807,
-0.0149499999999996));
#50995=CARTESIAN_POINT('',(0.0326814423280684,-0.196779569448551,-0.01495));
#50996=CARTESIAN_POINT('Origin',(0.,0.,-0.0149499999999998));
#50997=CARTESIAN_POINT('Ctrl Pts',(-0.199405777330601,0.000173947029632086,
-0.0370454881395214));
#50998=CARTESIAN_POINT('Ctrl Pts',(-0.198920212120655,-0.0488485699620836,
-0.0339200830333429));
#50999=CARTESIAN_POINT('Ctrl Pts',(-0.155869131157208,-0.165069700487324,
-0.0265549203201691));
#51000=CARTESIAN_POINT('Ctrl Pts',(-0.0328441439546209,-0.207662155862942,
-0.0191897576069953));
#51001=CARTESIAN_POINT('Ctrl Pts',(0.0326814423280684,-0.196779569448551,
-0.01495));
#51002=CARTESIAN_POINT('Origin',(0.,0.,-1.69285451186048));
#51003=CARTESIAN_POINT('',(-0.199280164752556,-0.000151800512929585,-0.132854511860476));
#51004=CARTESIAN_POINT('',(-0.199798270692528,-3.2584075625286E-5,-0.117045488139522));
#51005=CARTESIAN_POINT('',(-0.199475,-2.40257419738789E-14,-1.69285451186048));
#51006=CARTESIAN_POINT('Ctrl Pts',(-0.199280164752556,-0.000151800512929595,
-0.132854511860476));
#51007=CARTESIAN_POINT('Ctrl Pts',(-0.199439342569838,-0.0226838987709636,
-0.131419428744494));
#51008=CARTESIAN_POINT('Ctrl Pts',(-0.185501100147388,-0.111592971135028,
-0.125744588021516));
#51009=CARTESIAN_POINT('Ctrl Pts',(-0.0546225418096208,-0.229469274023813,
-0.115829989691543));
#51010=CARTESIAN_POINT('Ctrl Pts',(0.16340138241606,-0.170114291722319,
-0.103110716870557));
#51011=CARTESIAN_POINT('Ctrl Pts',(0.231483868070962,0.0453453091881316,
-0.0903914440495704));
#51012=CARTESIAN_POINT('Ctrl Pts',(0.0871316520886174,0.219198428493199,
-0.0776721712285846));
#51013=CARTESIAN_POINT('Ctrl Pts',(-0.133507657360752,0.192336088231908,
-0.0651598604988864));
#51014=CARTESIAN_POINT('Ctrl Pts',(-0.199545879878187,0.0628540441225657,
-0.0568873073761835));
#51015=CARTESIAN_POINT('Ctrl Pts',(-0.19978905918818,-5.64256782074292E-5,
-0.0528545118604759));
#51016=CARTESIAN_POINT('Ctrl Pts',(-0.199798270692528,-3.25840756252845E-5,
-0.117045488139522));
#51017=CARTESIAN_POINT('Ctrl Pts',(-0.199802333431698,-0.00180695869165221,
-0.116931719615644));
#51018=CARTESIAN_POINT('Ctrl Pts',(-0.198975693736128,-0.0697022559227335,
-0.112578193484771));
#51019=CARTESIAN_POINT('Ctrl Pts',(-0.122283640616722,-0.201709157150624,
-0.103984909746902));
#51020=CARTESIAN_POINT('Ctrl Pts',(0.10342756844873,-0.21198412740384,-0.091265636925916));
#51021=CARTESIAN_POINT('Ctrl Pts',(0.234263184552909,-0.0277545195405686,
-0.0785463641049296));
#51022=CARTESIAN_POINT('Ctrl Pts',(0.150056069810251,0.181992167351128,
-0.0658270912839439));
#51023=CARTESIAN_POINT('Ctrl Pts',(-0.0717210418700825,0.224640263091484,
-0.0531078184629578));
#51024=CARTESIAN_POINT('Ctrl Pts',(-0.189548818024464,0.101452165564304,
-0.0435139507481504));
#51025=CARTESIAN_POINT('Ctrl Pts',(-0.199578903945434,0.0176527577918152,
-0.0381598406403383));
#51026=CARTESIAN_POINT('Ctrl Pts',(-0.199405777330601,0.000173947029632086,
-0.0370454881395214));
#51027=CARTESIAN_POINT('Origin',(0.,0.,-1.69285451186048));
#51028=CARTESIAN_POINT('',(-0.199232182693492,0.000127961726227482,-0.212854511860476));
#51029=CARTESIAN_POINT('',(-0.19931604476105,-0.000164312884269185,-0.197045488139522));
#51030=CARTESIAN_POINT('',(-0.199475,-2.40257419738789E-14,-1.69285451186048));
#51031=CARTESIAN_POINT('Ctrl Pts',(-0.199232182693492,0.000127961726227475,
-0.212854511860476));
#51032=CARTESIAN_POINT('Ctrl Pts',(-0.198987070943203,-0.0417119960123555,
-0.210191307719799));
#51033=CARTESIAN_POINT('Ctrl Pts',(-0.165649967516347,-0.15051751299201,
-0.203288345972126));
#51034=CARTESIAN_POINT('Ctrl Pts',(0.0131260578517699,-0.235515155392752,
-0.192145626617459));
#51035=CARTESIAN_POINT('Ctrl Pts',(0.205151283752445,-0.116415679756492,
-0.179426353796472));
#51036=CARTESIAN_POINT('Ctrl Pts',(0.208917206173459,0.109513919792018,
-0.166707080975487));
#51037=CARTESIAN_POINT('Ctrl Pts',(0.0209676371933062,0.234946925588856,
-0.1539878081545));
#51038=CARTESIAN_POINT('Ctrl Pts',(-0.162845934874777,0.154951522837623,
-0.142703618449497));
#51039=CARTESIAN_POINT('Ctrl Pts',(-0.198969073388792,0.0438841166471984,
-0.135659186351489));
#51040=CARTESIAN_POINT('Ctrl Pts',(-0.199280164752556,-0.000151800512929595,
-0.132854511860476));
#51041=CARTESIAN_POINT('Ctrl Pts',(-0.19931604476105,-0.000164312884269184,
-0.197045488139521));
#51042=CARTESIAN_POINT('Ctrl Pts',(-0.199479051453381,-0.0212236085435869,
-0.195703598590949));
#51043=CARTESIAN_POINT('Ctrl Pts',(-0.186700843720701,-0.10862791766991,
-0.190121951435381));
#51044=CARTESIAN_POINT('Ctrl Pts',(-0.0596484344001499,-0.228214284403755,
-0.180300546672818));
#51045=CARTESIAN_POINT('Ctrl Pts',(0.159628272860435,-0.173661646916563,
-0.167581273851832));
#51046=CARTESIAN_POINT('Ctrl Pts',(0.232421018722115,0.0402530640696309,
-0.154862001030846));
#51047=CARTESIAN_POINT('Ctrl Pts',(0.0919285295363725,0.217230088081641,
-0.14214272820986));
#51048=CARTESIAN_POINT('Ctrl Pts',(-0.130909325195414,0.195061612321686,
-0.129537223912752));
#51049=CARTESIAN_POINT('Ctrl Pts',(-0.19965092925845,0.0643178183514808,
-0.121171477222639));
#51050=CARTESIAN_POINT('Ctrl Pts',(-0.199798270692528,-3.25840756252845E-5,
-0.117045488139522));
#51051=CARTESIAN_POINT('Origin',(0.,0.,-1.69285451186048));
#51052=CARTESIAN_POINT('',(-0.199747309326353,9.62307426035103E-5,-0.292854511860476));
#51053=CARTESIAN_POINT('',(-0.199205763221826,0.000109377304542274,-0.277045488139522));
#51054=CARTESIAN_POINT('',(-0.199475,-2.40257419738789E-14,-1.69285451186048));
#51055=CARTESIAN_POINT('Ctrl Pts',(-0.199747309326353,9.62307426035014E-5,
-0.292854511860476));
#51056=CARTESIAN_POINT('Ctrl Pts',(-0.199386580426527,-0.0606345073915193,
-0.288963186695104));
#51057=CARTESIAN_POINT('Ctrl Pts',(-0.137371276050314,-0.188171277532572,
-0.280832103922736));
#51058=CARTESIAN_POINT('Ctrl Pts',(0.0797840202277238,-0.221977898961698,
-0.268461263543375));
#51059=CARTESIAN_POINT('Ctrl Pts',(0.229840910738551,-0.0530361458245903,
-0.255741990722388));
#51060=CARTESIAN_POINT('Ctrl Pts',(0.168981662475758,0.164574832115758,
-0.243022717901402));
#51061=CARTESIAN_POINT('Ctrl Pts',(-0.0469455463466026,0.231161834775108,
-0.230303445080416));
#51062=CARTESIAN_POINT('Ctrl Pts',(-0.18360132481013,0.116094458771798,
-0.220247376400108));
#51063=CARTESIAN_POINT('Ctrl Pts',(-0.199377283015938,0.024896220905409,
-0.214431065326794));
#51064=CARTESIAN_POINT('Ctrl Pts',(-0.199232182693492,0.000127961726227475,
-0.212854511860476));
#51065=CARTESIAN_POINT('Ctrl Pts',(-0.199205763221826,0.000109377304542285,
-0.277045488139522));
#51066=CARTESIAN_POINT('Ctrl Pts',(-0.199005192472171,-0.0402798854940347,
-0.274475477566255));
#51067=CARTESIAN_POINT('Ctrl Pts',(-0.167435605774816,-0.147587685310038,
-0.267665709385992));
#51068=CARTESIAN_POINT('Ctrl Pts',(0.00795180063483016,-0.23574656447556,
-0.256616183598734));
#51069=CARTESIAN_POINT('Ctrl Pts',(0.202545773298689,-0.12089201855432,
-0.243896910777748));
#51070=CARTESIAN_POINT('Ctrl Pts',(0.211271315496057,0.10490046033926,-0.231177637956761));
#51071=CARTESIAN_POINT('Ctrl Pts',(0.0261212881376767,0.234429852510476,
-0.218458365135776));
#51072=CARTESIAN_POINT('Ctrl Pts',(-0.160936868752923,0.157862587704772,
-0.207080981863362));
#51073=CARTESIAN_POINT('Ctrl Pts',(-0.198964024814612,0.0453141397118719,
-0.199943356197944));
#51074=CARTESIAN_POINT('Ctrl Pts',(-0.19931604476105,-0.000164312884269184,
-0.197045488139521));
#51075=CARTESIAN_POINT('Origin',(0.,0.,-1.69285451186048));
#51076=CARTESIAN_POINT('',(-0.19952645684413,-0.000179680236322701,-0.372854511860476));
#51077=CARTESIAN_POINT('',(-0.199716645377052,0.000117807287515384,-0.357045488139522));
#51078=CARTESIAN_POINT('',(-0.199475,-2.40257419738789E-14,-1.69285451186048));
#51079=CARTESIAN_POINT('Ctrl Pts',(-0.19952645684413,-0.000179680236322737,
-0.372854511860476));
#51080=CARTESIAN_POINT('Ctrl Pts',(-0.19965407975718,-0.0139482848893583,
-0.371974823277405));
#51081=CARTESIAN_POINT('Ctrl Pts',(-0.192069331498236,-0.0939365192239043,
-0.366855377087338));
#51082=CARTESIAN_POINT('Ctrl Pts',(-0.0840994204847348,-0.220379138866998,
-0.357496173290276));
#51083=CARTESIAN_POINT('Ctrl Pts',(0.139807809013192,-0.189982772682906,
-0.344776900469291));
#51084=CARTESIAN_POINT('Ctrl Pts',(0.235418803056905,0.014753458384602,
-0.332057627648304));
#51085=CARTESIAN_POINT('Ctrl Pts',(0.11499503919352,0.205951009552392,-0.319338354827319));
#51086=CARTESIAN_POINT('Ctrl Pts',(-0.110955238097539,0.208155260646928,
-0.306619082006331));
#51087=CARTESIAN_POINT('Ctrl Pts',(-0.19710964318935,0.0771084030278873,
-0.297791134350718));
#51088=CARTESIAN_POINT('Ctrl Pts',(-0.199779609287417,0.00553411076300435,
-0.2932029443021));
#51089=CARTESIAN_POINT('Ctrl Pts',(-0.199747309326353,9.62307426035014E-5,
-0.292854511860476));
#51090=CARTESIAN_POINT('Ctrl Pts',(-0.199716645377052,0.000117807287515386,
-0.357045488139522));
#51091=CARTESIAN_POINT('Ctrl Pts',(-0.199301888682071,-0.0591824740362239,
-0.353247356541559));
#51092=CARTESIAN_POINT('Ctrl Pts',(-0.139839812362773,-0.185400255066588,
-0.345209467336602));
#51093=CARTESIAN_POINT('Ctrl Pts',(0.0748909360789789,-0.223676151397489,
-0.332931820524649));
#51094=CARTESIAN_POINT('Ctrl Pts',(0.228621008521177,-0.0580698493273639,
-0.320212547703664));
#51095=CARTESIAN_POINT('Ctrl Pts',(0.172554397257742,0.160824914104033,
-0.307493274882677));
#51096=CARTESIAN_POINT('Ctrl Pts',(-0.0418587313987176,0.232136855608358,
-0.294774002061692));
#51097=CARTESIAN_POINT('Ctrl Pts',(-0.182297588611502,0.119059390862335,
-0.284624739813973));
#51098=CARTESIAN_POINT('Ctrl Pts',(-0.199336074909168,0.0263504567980952,
-0.27871523517325));
#51099=CARTESIAN_POINT('Ctrl Pts',(-0.199205763221826,0.000109377304542285,
-0.277045488139522));
#51100=CARTESIAN_POINT('Origin',(0.,0.,-1.69285451186048));
#51101=CARTESIAN_POINT('',(-0.199145764441746,-3.13449387460375E-6,-0.452854511860477));
#51102=CARTESIAN_POINT('',(-0.199570626225687,-0.000172606811285253,-0.437045488139522));
#51103=CARTESIAN_POINT('',(-0.199475,-2.40257419738789E-14,-1.69285451186048));
#51104=CARTESIAN_POINT('Ctrl Pts',(-0.199145793344766,-3.13421870281119E-6,
-0.452854511860477));
#51105=CARTESIAN_POINT('Ctrl Pts',(-0.199150426498933,-0.0331535588910306,
-0.450746702252711));
#51106=CARTESIAN_POINT('Ctrl Pts',(-0.175592596745264,-0.132978274684061,
-0.444399135037949));
#51107=CARTESIAN_POINT('Ctrl Pts',(-0.0177182263414914,-0.235214246654171,
-0.433811810216192));
#51108=CARTESIAN_POINT('Ctrl Pts',(0.188206317046981,-0.142190223283767,
-0.421092537395206));
#51109=CARTESIAN_POINT('Ctrl Pts',(0.221421180402404,0.081316285225576,
-0.40837326457422));
#51110=CARTESIAN_POINT('Ctrl Pts',(0.051446364370158,0.230201974289577,
-0.395653991753234));
#51111=CARTESIAN_POINT('Ctrl Pts',(-0.150717866526423,0.17215324521349,
-0.383814407515319));
#51112=CARTESIAN_POINT('Ctrl Pts',(-0.19903898684039,0.0524110466272596,
-0.3762145808844));
#51113=CARTESIAN_POINT('Ctrl Pts',(-0.19952645684413,-0.000179680236322737,
-0.372854511860476));
#51114=CARTESIAN_POINT('Ctrl Pts',(-0.199570626225687,-0.000172606811285283,
-0.437045488139522));
#51115=CARTESIAN_POINT('Ctrl Pts',(-0.199682928323807,-0.0124755616086236,
-0.43625899312386));
#51116=CARTESIAN_POINT('Ctrl Pts',(-0.193038335109565,-0.0909790538091767,
-0.431232740501203));
#51117=CARTESIAN_POINT('Ctrl Pts',(-0.0889178870534499,-0.21847947809828,
-0.421966730271551));
#51118=CARTESIAN_POINT('Ctrl Pts',(0.135602752200584,-0.193006649067832,
-0.409247457450565));
#51119=CARTESIAN_POINT('Ctrl Pts',(0.235685974516513,0.00958093959523976,
-0.396528184629579));
#51120=CARTESIAN_POINT('Ctrl Pts',(0.119489265933811,0.20337646942222,-0.383808911808593));
#51121=CARTESIAN_POINT('Ctrl Pts',(-0.106358134575664,0.210541255342925,
-0.371089638987607));
#51122=CARTESIAN_POINT('Ctrl Pts',(-0.196308748593597,0.0800545266610567,
-0.362168497764583));
#51123=CARTESIAN_POINT('Ctrl Pts',(-0.199764871021477,0.00701292029244546,
-0.357487114148555));
#51124=CARTESIAN_POINT('Ctrl Pts',(-0.199716645377052,0.000117807287515386,
-0.357045488139522));
#51125=CARTESIAN_POINT('Origin',(0.,0.,-1.69285451186048));
#51126=CARTESIAN_POINT('',(-0.199514918438111,0.000180945765229524,-0.532854511860476));
#51127=CARTESIAN_POINT('',(-0.1991491027263,-2.72391900677377E-5,-0.517045488139522));
#51128=CARTESIAN_POINT('',(-0.199475,-2.40257419738789E-14,-1.69285451186048));
#51129=CARTESIAN_POINT('Ctrl Pts',(-0.199514918438111,0.000180945765229527,
-0.532854511860476));
#51130=CARTESIAN_POINT('Ctrl Pts',(-0.199030404431233,-0.0520397267160747,
-0.529518581228016));
#51131=CARTESIAN_POINT('Ctrl Pts',(-0.15128305072811,-0.171413952745693,
-0.521942892988561));
#51132=CARTESIAN_POINT('Ctrl Pts',(0.0501362714953425,-0.230490849393937,
-0.510127447142107));
#51133=CARTESIAN_POINT('Ctrl Pts',(0.220955117411352,-0.0825742905723761,
-0.497408174321123));
#51134=CARTESIAN_POINT('Ctrl Pts',(0.189011971974381,0.141117510692855,
-0.484688901500136));
#51135=CARTESIAN_POINT('Ctrl Pts',(-0.0163801719563586,0.235311213800938,
-0.47196962867915));
#51136=CARTESIAN_POINT('Ctrl Pts',(-0.175194713167085,0.133743756730128,
-0.46135816546593));
#51137=CARTESIAN_POINT('Ctrl Pts',(-0.199141107132255,0.0335269252768801,
-0.454986459859706));
#51138=CARTESIAN_POINT('Ctrl Pts',(-0.199145793344766,-3.13421870281119E-6,
-0.452854511860477));
#51139=CARTESIAN_POINT('Ctrl Pts',(-0.1991491027263,-2.72391900677377E-5,
-0.517045488139522));
#51140=CARTESIAN_POINT('Ctrl Pts',(-0.19918762421967,-0.0317106516158013,
-0.515030872099166));
#51141=CARTESIAN_POINT('Ctrl Pts',(-0.177100415645962,-0.130021035991661,
-0.508776498451814));
#51142=CARTESIAN_POINT('Ctrl Pts',(-0.0228784244999453,-0.234768504447706,
-0.498282367197467));
#51143=CARTESIAN_POINT('Ctrl Pts',(0.185038945608821,-0.146288282497961,
-0.485563094376481));
#51144=CARTESIAN_POINT('Ctrl Pts',(0.223153210321907,0.0764350555126916,
-0.472843821555495));
#51145=CARTESIAN_POINT('Ctrl Pts',(0.0564883785752809,0.229016890368669,
-0.46012454873451));
#51146=CARTESIAN_POINT('Ctrl Pts',(-0.148502607420017,0.174999094124885,
-0.448191770929184));
#51147=CARTESIAN_POINT('Ctrl Pts',(-0.199077541556816,0.0538459600181255,
-0.440498750730856));
#51148=CARTESIAN_POINT('Ctrl Pts',(-0.199570626225687,-0.000172606811285283,
-0.437045488139522));
#51149=CARTESIAN_POINT('Origin',(0.,0.,-1.69285451186048));
#51150=CARTESIAN_POINT('',(-0.199754379428577,-9.02611387494427E-5,-0.612854511860476));
#51151=CARTESIAN_POINT('',(-0.199470369800604,0.000183637767226734,-0.597045488139522));
#51152=CARTESIAN_POINT('',(-0.199475,-2.40257419738789E-14,-1.69285451186048));
#51153=CARTESIAN_POINT('Ctrl Pts',(-0.199754379428577,-9.02611387494983E-5,
-0.612854511860476));
#51154=CARTESIAN_POINT('Ctrl Pts',(-0.199782877503472,-0.00515094661274952,
-0.612530217810316));
#51155=CARTESIAN_POINT('Ctrl Pts',(-0.197311473429714,-0.0763457633342411,
-0.60796616615316));
#51156=CARTESIAN_POINT('Ctrl Pts',(-0.112137314847476,-0.207520842308891,
-0.599162356889011));
#51157=CARTESIAN_POINT('Ctrl Pts',(0.113821844477603,-0.206601706414806,
-0.586443084068023));
#51158=CARTESIAN_POINT('Ctrl Pts',(0.235331086026933,-0.0160921509804536,
-0.573723811247038));
#51159=CARTESIAN_POINT('Ctrl Pts',(0.140886064153414,0.189184550905072,
-0.561004538426052));
#51160=CARTESIAN_POINT('Ctrl Pts',(-0.0828446663124362,0.22085388526665,
-0.548285265605067));
#51161=CARTESIAN_POINT('Ctrl Pts',(-0.191812282577816,0.0947028634056557,
-0.53890192341654));
#51162=CARTESIAN_POINT('Ctrl Pts',(-0.199646191200409,0.0143294571154524,
-0.533758338835011));
#51163=CARTESIAN_POINT('Ctrl Pts',(-0.199514918438111,0.000180945765229527,
-0.532854511860476));
#51164=CARTESIAN_POINT('Ctrl Pts',(-0.199470369800604,0.000183637767226717,
-0.597045488139522));
#51165=CARTESIAN_POINT('Ctrl Pts',(-0.199002463741088,-0.0506072066419029,
-0.593802751074471));
#51166=CARTESIAN_POINT('Ctrl Pts',(-0.15343214889695,-0.168551718593714,
-0.586320256402424));
#51167=CARTESIAN_POINT('Ctrl Pts',(0.0450634218898312,-0.231536090050329,
-0.574598004123383));
#51168=CARTESIAN_POINT('Ctrl Pts',(0.219088804207135,-0.0874057713157602,
-0.561878731302397));
#51169=CARTESIAN_POINT('Ctrl Pts',(0.192064838835073,0.136933453441709,
-0.54915945848141));
#51170=CARTESIAN_POINT('Ctrl Pts',(-0.0112096232321388,0.235614128046703,
-0.536440185660426));
#51171=CARTESIAN_POINT('Ctrl Pts',(-0.173629946925928,0.136697002188027,
-0.525735528879795));
#51172=CARTESIAN_POINT('Ctrl Pts',(-0.199106555772246,0.0349670607406491,
-0.519270629706161));
#51173=CARTESIAN_POINT('Ctrl Pts',(-0.1991491027263,-2.72391900677377E-5,
-0.517045488139522));
#51174=CARTESIAN_POINT('Origin',(0.,0.,-1.69285451186048));
#51175=CARTESIAN_POINT('',(-0.199239712079179,-0.000132428612020959,-0.692854511860477));
#51176=CARTESIAN_POINT('',(-0.199777832380642,-6.59547829733875E-5,-0.677045488139522));
#51177=CARTESIAN_POINT('',(-0.199475,-2.40257419738789E-14,-1.69285451186048));
#51178=CARTESIAN_POINT('Ctrl Pts',(-0.199239712079179,-0.000132428612020962,
-0.692854511860477));
#51179=CARTESIAN_POINT('Ctrl Pts',(-0.199387925235899,-0.0245191527044881,
-0.691302096785622));
#51180=CARTESIAN_POINT('Ctrl Pts',(-0.183932189689554,-0.11532642708485,
-0.685509924103772));
#51181=CARTESIAN_POINT('Ctrl Pts',(-0.0482595044417223,-0.23089109468499,
-0.675477993814925));
#51182=CARTESIAN_POINT('Ctrl Pts',(0.168042917961313,-0.165533244687709,
-0.662758720993941));
#51183=CARTESIAN_POINT('Ctrl Pts',(0.230138834184335,0.0517280810978802,
-0.650039448172953));
#51184=CARTESIAN_POINT('Ctrl Pts',(0.0810452162903746,0.221520541463405,
-0.637320175351968));
#51185=CARTESIAN_POINT('Ctrl Pts',(-0.136722929391739,0.188885971979512,
-0.624925196581142));
#51186=CARTESIAN_POINT('Ctrl Pts',(-0.199410299191403,0.0610114751905463,
-0.616769975417311));
#51187=CARTESIAN_POINT('Ctrl Pts',(-0.199754379428577,-9.02611387494983E-5,
-0.612854511860476));
#51188=CARTESIAN_POINT('Ctrl Pts',(-0.199777832380642,-6.59547829734257E-5,
-0.677045488139522));
#51189=CARTESIAN_POINT('Ctrl Pts',(-0.199793333714704,-0.0036712079644515,
-0.676814387656772));
#51190=CARTESIAN_POINT('Ctrl Pts',(-0.198069267605619,-0.0734031236255173,
-0.672343529567026));
#51191=CARTESIAN_POINT('Ctrl Pts',(-0.116666698598652,-0.205008669149152,
-0.663632913870284));
#51192=CARTESIAN_POINT('Ctrl Pts',(0.109258160368663,-0.209051016216307,
-0.650913641049299));
#51193=CARTESIAN_POINT('Ctrl Pts',(0.234921018494109,-0.0212553065822581,
-0.638194368228312));
#51194=CARTESIAN_POINT('Ctrl Pts',(0.145005916359623,0.186045578310588,
-0.625475095407328));
#51195=CARTESIAN_POINT('Ctrl Pts',(-0.0779755238778273,0.222619609792564,
-0.612755822586341));
#51196=CARTESIAN_POINT('Ctrl Pts',(-0.19079618970027,0.0976627030116315,
-0.603279286830406));
#51197=CARTESIAN_POINT('Ctrl Pts',(-0.199614233439153,0.015799925552125,
-0.598042508681467));
#51198=CARTESIAN_POINT('Ctrl Pts',(-0.199470369800604,0.000183637767226717,
-0.597045488139522));
#51199=CARTESIAN_POINT('Origin',(0.,0.,-1.69285451186048));
#51200=CARTESIAN_POINT('',(-0.199271260405861,0.000148188788378376,-0.772854511860477));
#51201=CARTESIAN_POINT('',(-0.199271252552475,-0.00014818878255532,-0.757045488139522));
#51202=CARTESIAN_POINT('',(-0.199475,-2.40257419738789E-14,-1.69285451186048));
#51203=CARTESIAN_POINT('Ctrl Pts',(-0.199271260405861,0.000148188788378367,
-0.772854511860477));
#51204=CARTESIAN_POINT('Ctrl Pts',(-0.198971206859014,-0.0435135905361769,
-0.770073975760927));
#51205=CARTESIAN_POINT('Ctrl Pts',(-0.163332551127985,-0.154196284756057,
-0.763053682054382));
#51206=CARTESIAN_POINT('Ctrl Pts',(0.0196311741237908,-0.235062320196826,
-0.751793630740842));
#51207=CARTESIAN_POINT('Ctrl Pts',(0.208290908157902,-0.110700383705523,
-0.739074357919856));
#51208=CARTESIAN_POINT('Ctrl Pts',(0.205810107346701,0.115247026372627,
-0.726355085098869));
#51209=CARTESIAN_POINT('Ctrl Pts',(0.0144653069364513,0.235436684204114,
-0.713635812277884));
#51210=CARTESIAN_POINT('Ctrl Pts',(-0.16517954457325,0.151275282131266,
-0.702468954531752));
#51211=CARTESIAN_POINT('Ctrl Pts',(-0.198983144408374,0.0420827507783096,
-0.695541854392617));
#51212=CARTESIAN_POINT('Ctrl Pts',(-0.199239712079179,-0.000132428612020962,
-0.692854511860477));
#51213=CARTESIAN_POINT('Ctrl Pts',(-0.199271252552475,-0.000148188782555318,
-0.757045488139522));
#51214=CARTESIAN_POINT('Ctrl Pts',(-0.19942872023353,-0.0230618294085849,
-0.755586266632077));
#51215=CARTESIAN_POINT('Ctrl Pts',(-0.185183518334068,-0.112361096942695,
-0.749887287517637));
#51216=CARTESIAN_POINT('Ctrl Pts',(-0.0533174176740989,-0.229775816744889,
-0.739948550796201));
#51217=CARTESIAN_POINT('Ctrl Pts',(0.164367878228055,-0.169182958938016,
-0.727229277975214));
#51218=CARTESIAN_POINT('Ctrl Pts',(0.231219110206101,0.0466625766939018,
-0.714510005154229));
#51219=CARTESIAN_POINT('Ctrl Pts',(0.085889480416779,0.219687664974506,
-0.701790732333243));
#51220=CARTESIAN_POINT('Ctrl Pts',(-0.134185014399097,0.191633020719834,
-0.689302559995007));
#51221=CARTESIAN_POINT('Ctrl Pts',(-0.199508947034822,0.0624705820456586,
-0.681054145263767));
#51222=CARTESIAN_POINT('Ctrl Pts',(-0.199777832380642,-6.59547829734257E-5,
-0.677045488139522));
#51223=CARTESIAN_POINT('Origin',(0.,0.,-1.69285451186048));
#51224=CARTESIAN_POINT('',(-0.199777840253992,6.59547855500507E-5,-0.852854511860477));
#51225=CARTESIAN_POINT('',(-0.199239704227035,0.000132428606779117,-0.837045488139522));
#51226=CARTESIAN_POINT('',(-0.199475,-2.40257419738789E-14,-1.69285451186048));
#51227=CARTESIAN_POINT('Ctrl Pts',(-0.199777840253992,6.59547855500525E-5,
-0.852854511860478));
#51228=CARTESIAN_POINT('Ctrl Pts',(-0.199508954897568,-0.0624705845076746,
-0.848845854736233));
#51229=CARTESIAN_POINT('Ctrl Pts',(-0.134185019687388,-0.191633028272198,
-0.840597440004992));
#51230=CARTESIAN_POINT('Ctrl Pts',(0.0858894838017356,-0.219687673632512,
-0.828109267666759));
#51231=CARTESIAN_POINT('Ctrl Pts',(0.23121911931857,-0.0466625785328924,
-0.81538999484577));
#51232=CARTESIAN_POINT('Ctrl Pts',(0.164367884705876,0.169182965605612,
-0.802670722024787));
#51233=CARTESIAN_POINT('Ctrl Pts',(-0.0533174197753734,0.229775825800475,
-0.789951449203798));
#51234=CARTESIAN_POINT('Ctrl Pts',(-0.185183525632255,0.112361101370898,
-0.780012712482364));
#51235=CARTESIAN_POINT('Ctrl Pts',(-0.199428728093124,0.0230618303174506,
-0.774313733367923));
#51236=CARTESIAN_POINT('Ctrl Pts',(-0.199271260405861,0.000148188788378367,
-0.772854511860477));
#51237=CARTESIAN_POINT('Ctrl Pts',(-0.199239704227035,0.000132428606779098,
-0.837045488139522));
#51238=CARTESIAN_POINT('Ctrl Pts',(-0.198983136566337,-0.0420827491198241,
-0.834358145607383));
#51239=CARTESIAN_POINT('Ctrl Pts',(-0.165179538063425,-0.151275276169436,
-0.827431045468248));
#51240=CARTESIAN_POINT('Ctrl Pts',(0.0144653063663763,-0.235436674925429,
-0.816264187722117));
#51241=CARTESIAN_POINT('Ctrl Pts',(0.205810099235619,-0.115247021830672,
-0.80354491490113));
#51242=CARTESIAN_POINT('Ctrl Pts',(0.208290899949043,0.110700379342769,
-0.790825642080145));
#51243=CARTESIAN_POINT('Ctrl Pts',(0.019631173350109,0.235062310932895,
-0.778106369259159));
#51244=CARTESIAN_POINT('Ctrl Pts',(-0.16333254469097,0.154196278679093,
-0.766846317945618));
#51245=CARTESIAN_POINT('Ctrl Pts',(-0.198971199017457,0.0435135888212697,
-0.759826024239072));
#51246=CARTESIAN_POINT('Ctrl Pts',(-0.199271252552475,-0.000148188782555318,
-0.757045488139522));
#51247=CARTESIAN_POINT('Origin',(0.,0.,-1.69285451186048));
#51248=CARTESIAN_POINT('',(-0.199470377661838,-0.000183637774485374,-0.932854511860477));
#51249=CARTESIAN_POINT('',(-0.199754371556151,9.02611351696198E-5,-0.917045488139523));
#51250=CARTESIAN_POINT('',(-0.199475,-2.40257419738789E-14,-1.69285451186048));
#51251=CARTESIAN_POINT('Ctrl Pts',(-0.199470377661838,-0.000183637774485384,
-0.932854511860477));
#51252=CARTESIAN_POINT('Ctrl Pts',(-0.199614241306055,-0.0157999261748247,
-0.931857491318533));
#51253=CARTESIAN_POINT('Ctrl Pts',(-0.190796197219643,-0.0976627068605806,
-0.926620713169594));
#51254=CARTESIAN_POINT('Ctrl Pts',(-0.0779755269508779,-0.222619618566124,
-0.917144177413659));
#51255=CARTESIAN_POINT('Ctrl Pts',(0.145005922074389,-0.186045585642739,
-0.904424904592673));
#51256=CARTESIAN_POINT('Ctrl Pts',(0.234921027752471,0.0212553074199478,
-0.891705631771688));
#51257=CARTESIAN_POINT('Ctrl Pts',(0.109258164674579,0.209051024455123,
-0.878986358950702));
#51258=CARTESIAN_POINT('Ctrl Pts',(-0.116666703196555,0.20500867722865,
-0.866267086129715));
#51259=CARTESIAN_POINT('Ctrl Pts',(-0.19806927541164,0.0734031265183624,
-0.857556470432975));
#51260=CARTESIAN_POINT('Ctrl Pts',(-0.199793341588666,0.00367120810911873,
-0.853085612343228));
#51261=CARTESIAN_POINT('Ctrl Pts',(-0.199777840253992,6.59547855500525E-5,
-0.852854511860478));
#51262=CARTESIAN_POINT('Ctrl Pts',(-0.199754371556151,9.02611351696076E-5,
-0.917045488139523));
#51263=CARTESIAN_POINT('Ctrl Pts',(-0.19941029133253,-0.0610114727860687,
-0.913130024582688));
#51264=CARTESIAN_POINT('Ctrl Pts',(-0.136722924003404,-0.188885964535421,
-0.904974803418858));
#51265=CARTESIAN_POINT('Ctrl Pts',(0.0810452130963459,-0.22152053273316,
-0.892579824648032));
#51266=CARTESIAN_POINT('Ctrl Pts',(0.230138825114443,-0.0517280790592424,
-0.879860551827046));
#51267=CARTESIAN_POINT('Ctrl Pts',(0.168042911338648,0.165533238163961,
-0.86714127900606));
#51268=CARTESIAN_POINT('Ctrl Pts',(-0.0482595025397965,0.230891085585448,
-0.854422006185075));
#51269=CARTESIAN_POINT('Ctrl Pts',(-0.183932182440697,0.115326422539765,
-0.844390075896228));
#51270=CARTESIAN_POINT('Ctrl Pts',(-0.199387917377917,0.0245191517381582,
-0.838597903214378));
#51271=CARTESIAN_POINT('Ctrl Pts',(-0.199239704227035,0.000132428606779098,
-0.837045488139522));
#51272=CARTESIAN_POINT('Origin',(0.,0.,-1.69285451186048));
#51273=CARTESIAN_POINT('',(-0.199149110574872,2.7239191122689E-5,-1.01285451186048));
#51274=CARTESIAN_POINT('',(-0.199514910575122,-0.000180945758118223,-0.997045488139523));
#51275=CARTESIAN_POINT('',(-0.199475,-2.40257419738789E-14,-1.69285451186048));
#51276=CARTESIAN_POINT('Ctrl Pts',(-0.199149110574872,2.72391911226855E-5,
-1.01285451186048));
#51277=CARTESIAN_POINT('Ctrl Pts',(-0.199106563619138,-0.0349670621187339,
-1.01062937029384));
#51278=CARTESIAN_POINT('Ctrl Pts',(-0.173629953768769,-0.136697007575336,
-1.0041644711202));
#51279=CARTESIAN_POINT('Ctrl Pts',(-0.011209623673909,-0.235614137332382,
-0.993459814339576));
#51280=CARTESIAN_POINT('Ctrl Pts',(0.192064846404454,-0.136933458838324,
-0.980740541518589));
#51281=CARTESIAN_POINT('Ctrl Pts',(0.219088812841539,0.0874057747604746,
-0.968021268697603));
#51282=CARTESIAN_POINT('Ctrl Pts',(0.045063423665798,0.231536099175291,
-0.955301995876618));
#51283=CARTESIAN_POINT('Ctrl Pts',(-0.153432154943803,0.168551725236421,
-0.943579743597575));
#51284=CARTESIAN_POINT('Ctrl Pts',(-0.199002471583887,0.0506072086363436,
-0.936097248925528));
#51285=CARTESIAN_POINT('Ctrl Pts',(-0.199470377661838,-0.000183637774485384,
-0.932854511860477));
#51286=CARTESIAN_POINT('Ctrl Pts',(-0.199514910575122,-0.000180945758118245,
-0.997045488139523));
#51287=CARTESIAN_POINT('Ctrl Pts',(-0.199646183332245,-0.0143294565507365,
-0.996141661164988));
#51288=CARTESIAN_POINT('Ctrl Pts',(-0.191812275018386,-0.094702859673376,
-0.990998076583459));
#51289=CARTESIAN_POINT('Ctrl Pts',(-0.0828446630474759,-0.220853876562684,
-0.981614734394935));
#51290=CARTESIAN_POINT('Ctrl Pts',(0.140886058601026,-0.189184543449203,
-0.968895461573948));
#51291=CARTESIAN_POINT('Ctrl Pts',(0.23533107675241,0.0160921503462616,
-0.956176188752962));
#51292=CARTESIAN_POINT('Ctrl Pts',(0.113821839991816,0.206601698272528,
-0.943456915931977));
#51293=CARTESIAN_POINT('Ctrl Pts',(-0.112137310428092,0.20752083413038,
-0.93073764311099));
#51294=CARTESIAN_POINT('Ctrl Pts',(-0.19731146565357,0.0763457603254025,
-0.921933833846839));
#51295=CARTESIAN_POINT('Ctrl Pts',(-0.199782869629924,0.00515094640973097,
-0.917369782189683));
#51296=CARTESIAN_POINT('Ctrl Pts',(-0.199754371556151,9.02611351696076E-5,
-0.917045488139523));
#51297=CARTESIAN_POINT('Origin',(0.,0.,-1.69285451186048));
#51298=CARTESIAN_POINT('',(-0.199570634090872,0.000172606818067552,-1.09285451186048));
#51299=CARTESIAN_POINT('',(-0.199145756921865,3.13449059798551E-6,-1.07704548813952));
#51300=CARTESIAN_POINT('',(-0.199475,-2.40257419738789E-14,-1.69285451186048));
#51301=CARTESIAN_POINT('Ctrl Pts',(-0.199570634090872,0.000172606818067534,
-1.09285451186048));
#51302=CARTESIAN_POINT('Ctrl Pts',(-0.199077549402563,-0.0538459621402391,
-1.08940124926914));
#51303=CARTESIAN_POINT('Ctrl Pts',(-0.148502613272573,-0.174999101021697,
-1.08170822907082));
#51304=CARTESIAN_POINT('Ctrl Pts',(0.0564883808015244,-0.229016899394345,
-1.06977545126549));
#51305=CARTESIAN_POINT('Ctrl Pts',(0.223153219116496,-0.0764350585250314,
-1.0570561784445));
#51306=CARTESIAN_POINT('Ctrl Pts',(0.1850389529013,0.146288288263266,-1.04433690562352));
#51307=CARTESIAN_POINT('Ctrl Pts',(-0.022878425401603,0.234768513700057,
-1.03161763280253));
#51308=CARTESIAN_POINT('Ctrl Pts',(-0.177100422625592,0.130021041115852,
-1.02112350154819));
#51309=CARTESIAN_POINT('Ctrl Pts',(-0.199187632069763,0.0317106528655207,
-1.01486912790083));
#51310=CARTESIAN_POINT('Ctrl Pts',(-0.199149110574872,2.72391911226855E-5,
-1.01285451186048));
#51311=CARTESIAN_POINT('Ctrl Pts',(-0.199145785496325,3.13421856075122E-6,
-1.07704548813952));
#51312=CARTESIAN_POINT('Ctrl Pts',(-0.199141099283995,-0.0335269239555814,
-1.07491354014029));
#51313=CARTESIAN_POINT('Ctrl Pts',(-0.175194706262559,-0.133743751459225,
-1.06854183453407));
#51314=CARTESIAN_POINT('Ctrl Pts',(-0.0163801713107981,-0.235311204527198,
-1.05793037132085));
#51315=CARTESIAN_POINT('Ctrl Pts',(0.189011964525323,-0.141117505131332,
-1.04521109849986));
#51316=CARTESIAN_POINT('Ctrl Pts',(0.22095510870339,0.0825742873180875,
-1.03249182567888));
#51317=CARTESIAN_POINT('Ctrl Pts',(0.0501362695194371,0.230490840310171,
-1.01977255285789));
#51318=CARTESIAN_POINT('Ctrl Pts',(-0.151283044765976,0.171413945990171,
-1.00795710701144));
#51319=CARTESIAN_POINT('Ctrl Pts',(-0.199030396587344,0.0520397246651457,
-1.00038141877198));
#51320=CARTESIAN_POINT('Ctrl Pts',(-0.199514910575122,-0.000180945758118245,
-0.997045488139523));
#51321=CARTESIAN_POINT('Origin',(0.,0.,-1.69285451186048));
#51322=CARTESIAN_POINT('',(-0.199716653248,-0.000117807292186744,-1.17285451186048));
#51323=CARTESIAN_POINT('',(-0.199526448980684,0.000179680229220276,-1.15704548813952));
#51324=CARTESIAN_POINT('',(-0.199475,-2.40257419738789E-14,-1.69285451186048));
#51325=CARTESIAN_POINT('Ctrl Pts',(-0.199716653248,-0.000117807292186758,
-1.17285451186048));
#51326=CARTESIAN_POINT('Ctrl Pts',(-0.199764878894326,-0.00701292056885365,
-1.17241288585144));
#51327=CARTESIAN_POINT('Ctrl Pts',(-0.196308756330249,-0.0800545298160815,
-1.16773150223542));
#51328=CARTESIAN_POINT('Ctrl Pts',(-0.106358138767262,-0.21054126364045,
-1.15881036101239));
#51329=CARTESIAN_POINT('Ctrl Pts',(0.11948927064294,-0.203376477437402,
-1.14609108819141));
#51330=CARTESIAN_POINT('Ctrl Pts',(0.23568598380503,-0.00958093997281493,
-1.13337181537042));
#51331=CARTESIAN_POINT('Ctrl Pts',(0.13560275754475,0.193006656674328,-1.12065254254944));
#51332=CARTESIAN_POINT('Ctrl Pts',(-0.0889178905577564,0.218479486708672,
-1.10793326972845));
#51333=CARTESIAN_POINT('Ctrl Pts',(-0.193038342717315,0.0909790573946992,
-1.0986672594988));
#51334=CARTESIAN_POINT('Ctrl Pts',(-0.199682936193419,0.0124755621002766,
-1.09364100687614));
#51335=CARTESIAN_POINT('Ctrl Pts',(-0.199570634090872,0.000172606818067534,
-1.09285451186048));
#51336=CARTESIAN_POINT('Ctrl Pts',(-0.199526448980684,0.000179680229220268,
-1.15704548813952));
#51337=CARTESIAN_POINT('Ctrl Pts',(-0.199038978996149,-0.0524110445617291,
-1.1536854191156));
#51338=CARTESIAN_POINT('Ctrl Pts',(-0.150717860586543,-0.172153238428849,
-1.14608559248468));
#51339=CARTESIAN_POINT('Ctrl Pts',(0.051446362342642,-0.230201965217191,
-1.13424600824677));
#51340=CARTESIAN_POINT('Ctrl Pts',(0.221421171676079,-0.0813162820208495,
-1.12152673542578));
#51341=CARTESIAN_POINT('Ctrl Pts',(0.188206309629664,0.142190217679984,
-1.10880746260479));
#51342=CARTESIAN_POINT('Ctrl Pts',(-0.0177182256432174,0.235214237384252,
-1.09608818978381));
#51343=CARTESIAN_POINT('Ctrl Pts',(-0.175592589825075,0.132978269443307,
-1.08550086496205));
#51344=CARTESIAN_POINT('Ctrl Pts',(-0.199150418650312,0.0331535575844161,
-1.07915329774729));
#51345=CARTESIAN_POINT('Ctrl Pts',(-0.199145785496325,3.13421856075122E-6,
-1.07704548813952));
#51346=CARTESIAN_POINT('Origin',(0.,0.,-1.69285451186048));
#51347=CARTESIAN_POINT('',(-0.199205771072305,-0.000109377308561953,-1.25285451186048));
#51348=CARTESIAN_POINT('',(-0.199747301454138,-9.62307387931682E-5,-1.23704548813952));
#51349=CARTESIAN_POINT('',(-0.199475,-2.40257419738789E-14,-1.69285451186048));
#51350=CARTESIAN_POINT('Ctrl Pts',(-0.199205771072305,-0.000109377308561975,
-1.25285451186048));
#51351=CARTESIAN_POINT('Ctrl Pts',(-0.199336082765098,-0.0263504578365746,
-1.25118476482675));
#51352=CARTESIAN_POINT('Ctrl Pts',(-0.182297595797127,-0.119059395555614,
-1.24527526018603));
#51353=CARTESIAN_POINT('Ctrl Pts',(-0.0418587330474375,-0.232136864756142,
-1.23512599793831));
#51354=CARTESIAN_POINT('Ctrl Pts',(0.172554404057684,-0.16082492044269,
-1.22240672511732));
#51355=CARTESIAN_POINT('Ctrl Pts',(0.228621017531538,0.0580698516161886,
-1.20968745229634));
#51356=CARTESIAN_POINT('Ctrl Pts',(0.0748909390303039,0.223676160212552,
-1.19696817947535));
#51357=CARTESIAN_POINT('Ctrl Pts',(-0.13983981787387,0.185400262373372,
-1.1846905326634));
#51358=CARTESIAN_POINT('Ctrl Pts',(-0.199301896536666,0.0591824763686249,
-1.17665264345844));
#51359=CARTESIAN_POINT('Ctrl Pts',(-0.199716653248,-0.000117807292186758,
-1.17285451186048));
#51360=CARTESIAN_POINT('Ctrl Pts',(-0.199747301454138,-9.62307387932064E-5,
-1.23704548813952));
#51361=CARTESIAN_POINT('Ctrl Pts',(-0.199779601413921,-0.00553411054487472,
-1.2366970556979));
#51362=CARTESIAN_POINT('Ctrl Pts',(-0.197109635420976,-0.0771083999889113,
-1.23210886564928));
#51363=CARTESIAN_POINT('Ctrl Pts',(-0.110955233724902,-0.208155252443532,
-1.22328091799367));
#51364=CARTESIAN_POINT('Ctrl Pts',(0.11499503466161,-0.20595100143569,-1.21056164517268));
#51365=CARTESIAN_POINT('Ctrl Pts',(0.235418793778872,-0.0147534578031819,
-1.19784237235169));
#51366=CARTESIAN_POINT('Ctrl Pts',(0.139807803503312,0.189982765195607,
-1.18512309953071));
#51367=CARTESIAN_POINT('Ctrl Pts',(-0.0840994171703575,0.220379130181726,
-1.17240382670972));
#51368=CARTESIAN_POINT('Ctrl Pts',(-0.192069323928686,0.0939365155218052,
-1.16304462291266));
#51369=CARTESIAN_POINT('Ctrl Pts',(-0.199654071888705,0.0139482843396326,
-1.15792517672259));
#51370=CARTESIAN_POINT('Ctrl Pts',(-0.199526448980684,0.000179680229220268,
-1.15704548813952));
#51371=CARTESIAN_POINT('Origin',(0.,0.,-1.69285451186048));
#51372=CARTESIAN_POINT('',(-0.199316052586657,0.000164312921044613,-1.33285451186048));
#51373=CARTESIAN_POINT('',(-0.199232174843428,-0.0001279617224864,-1.31704548813952));
#51374=CARTESIAN_POINT('',(-0.199475,-2.40257419738789E-14,-1.69285451186048));
#51375=CARTESIAN_POINT('Ctrl Pts',(-0.199316052586657,0.000164312921044612,
-1.33285451186048));
#51376=CARTESIAN_POINT('Ctrl Pts',(-0.198964032636456,-0.0453141414772884,
-1.32995664380206));
#51377=CARTESIAN_POINT('Ctrl Pts',(-0.160936875144002,-0.157862593974603,
-1.32281901813664));
#51378=CARTESIAN_POINT('Ctrl Pts',(0.0261212891997552,-0.23442986171762,
-1.31144163486423));
#51379=CARTESIAN_POINT('Ctrl Pts',(0.211271323804121,-0.104900464490951,
-1.29872236204324));
#51380=CARTESIAN_POINT('Ctrl Pts',(0.202545781291298,0.120892023328345,
-1.28600308922225));
#51381=CARTESIAN_POINT('Ctrl Pts',(0.00795180094256099,0.2357465737612,
-1.27328381640127));
#51382=CARTESIAN_POINT('Ctrl Pts',(-0.167435612371573,0.147587691128348,
-1.26223429061401));
#51383=CARTESIAN_POINT('Ctrl Pts',(-0.199005200314261,0.0402798870822277,
-1.25542452243375));
#51384=CARTESIAN_POINT('Ctrl Pts',(-0.199205771072305,-0.000109377308561975,
-1.25285451186048));
#51385=CARTESIAN_POINT('Ctrl Pts',(-0.199232174843428,-0.000127961722486429,
-1.31704548813952));
#51386=CARTESIAN_POINT('Ctrl Pts',(-0.199377275158137,-0.0248962199241702,
-1.31546893467321));
#51387=CARTESIAN_POINT('Ctrl Pts',(-0.183601317566453,-0.116094454191202,
-1.30965262359989));
#51388=CARTESIAN_POINT('Ctrl Pts',(-0.0469455445028857,-0.231161825669147,
-1.29959655491958));
#51389=CARTESIAN_POINT('Ctrl Pts',(0.168981655819671,-0.164574825627453,
-1.2868772820986));
#51390=CARTESIAN_POINT('Ctrl Pts',(0.229840901678433,0.0530361437331597,
-1.27415800927761));
#51391=CARTESIAN_POINT('Ctrl Pts',(0.0797840170844622,0.22197789021412,
-1.26143873645663));
#51392=CARTESIAN_POINT('Ctrl Pts',(-0.137371270637,0.188171270116292,-1.24906789607726));
#51393=CARTESIAN_POINT('Ctrl Pts',(-0.199386572568632,0.0606345050018434,
-1.24093681330489));
#51394=CARTESIAN_POINT('Ctrl Pts',(-0.199747301454138,-9.62307387932064E-5,
-1.23704548813952));
#51395=CARTESIAN_POINT('Origin',(0.,0.,-1.69285451186048));
#51396=CARTESIAN_POINT('',(-0.199798277749891,3.2585087406417E-5,-1.41285451186048));
#51397=CARTESIAN_POINT('',(-0.199280157075849,0.000151800363860324,-1.39704548813952));
#51398=CARTESIAN_POINT('',(-0.199475,-2.40257419738789E-14,-1.69285451186048));
#51399=CARTESIAN_POINT('Ctrl Pts',(-0.199798277749891,3.25850874064147E-5,
-1.41285451186048));
#51400=CARTESIAN_POINT('Ctrl Pts',(-0.199650935957592,-0.0643178193354115,
-1.40872852277736));
#51401=CARTESIAN_POINT('Ctrl Pts',(-0.13090933192774,-0.195061621925552,
-1.40036277608725));
#51402=CARTESIAN_POINT('Ctrl Pts',(0.0919285341003431,-0.217230095550597,
-1.38775727179014));
#51403=CARTESIAN_POINT('Ctrl Pts',(0.232421027333792,-0.0402530662671006,
-1.37503799896916));
#51404=CARTESIAN_POINT('Ctrl Pts',(0.159628279467637,0.173661654101238,
-1.36231872614817));
#51405=CARTESIAN_POINT('Ctrl Pts',(-0.059648436931805,0.228214293208638,
-1.34959945332718));
#51406=CARTESIAN_POINT('Ctrl Pts',(-0.186700851040545,0.108627921988768,
-1.33977804856462));
#51407=CARTESIAN_POINT('Ctrl Pts',(-0.199479059280731,0.0212236094148981,
-1.33419640140905));
#51408=CARTESIAN_POINT('Ctrl Pts',(-0.199316052586657,0.000164312921044612,
-1.33285451186048));
#51409=CARTESIAN_POINT('Ctrl Pts',(-0.199280157075849,0.000151800363860317,
-1.39704548813952));
#51410=CARTESIAN_POINT('Ctrl Pts',(-0.198969065654869,-0.0438841150085429,
-1.39424081364851));
#51411=CARTESIAN_POINT('Ctrl Pts',(-0.162845928153855,-0.154951516497137,
-1.3871963815505));
#51412=CARTESIAN_POINT('Ctrl Pts',(0.0209676361572253,-0.234946916486012,
-1.3759121918455));
#51413=CARTESIAN_POINT('Ctrl Pts',(0.208917198058643,-0.109513915389758,
-1.36319291902451));
#51414=CARTESIAN_POINT('Ctrl Pts',(0.205151275600481,0.116415675121088,
-1.35047364620353));
#51415=CARTESIAN_POINT('Ctrl Pts',(0.0131260573719064,0.235515146136983,
-1.33775437338254));
#51416=CARTESIAN_POINT('Ctrl Pts',(-0.165649961001676,0.150517507050773,
-1.32661165402787));
#51417=CARTESIAN_POINT('Ctrl Pts',(-0.198987063106209,0.0417119943648623,
-1.3197086922802));
#51418=CARTESIAN_POINT('Ctrl Pts',(-0.199232174843428,-0.000127961722486429,
-1.31704548813952));
#51419=CARTESIAN_POINT('Origin',(0.,0.,-1.69285451186048));
#51420=CARTESIAN_POINT('',(-0.199405781844198,-0.000173944371801526,-1.49285451186048));
#51421=CARTESIAN_POINT('',(-0.199789055725603,5.64207037231385E-5,-1.47704548813952));
#51422=CARTESIAN_POINT('',(-0.199475,-2.40257419738789E-14,-1.69285451186048));
#51423=CARTESIAN_POINT('Ctrl Pts',(-0.199405781844198,-0.000173944371801573,
-1.49285451186048));
#51424=CARTESIAN_POINT('Ctrl Pts',(-0.19957890617447,-0.0176527449068341,
-1.49174015935966));
#51425=CARTESIAN_POINT('Ctrl Pts',(-0.189548811499923,-0.101452112831176,
-1.48638604925185));
#51426=CARTESIAN_POINT('Ctrl Pts',(-0.0717210652972735,-0.224640326086787,
-1.47679218153704));
#51427=CARTESIAN_POINT('Ctrl Pts',(0.150056091147136,-0.181992142895108,
-1.46407290871606));
#51428=CARTESIAN_POINT('Ctrl Pts',(0.234263183139456,0.0277545022598852,
-1.45135363589507));
#51429=CARTESIAN_POINT('Ctrl Pts',(0.103427579470953,0.211984146348435,
-1.43863436307408));
#51430=CARTESIAN_POINT('Ctrl Pts',(-0.122283649797262,0.201709159043015,
-1.4259150902531));
#51431=CARTESIAN_POINT('Ctrl Pts',(-0.198975701192239,0.069702259029704,
-1.41732180651523));
#51432=CARTESIAN_POINT('Ctrl Pts',(-0.199802340498938,0.00180695975846793,
-1.41296828038436));
#51433=CARTESIAN_POINT('Ctrl Pts',(-0.199798277749891,3.25850874064147E-5,
-1.41285451186048));
#51434=CARTESIAN_POINT('Ctrl Pts',(-0.199789055725603,5.64207037231446E-5,
-1.47704548813952));
#51435=CARTESIAN_POINT('Ctrl Pts',(-0.199545877469372,-0.0628540486324878,
-1.47301269262382));
#51436=CARTESIAN_POINT('Ctrl Pts',(-0.133507643719009,-0.192336071597138,
-1.46474013950111));
#51437=CARTESIAN_POINT('Ctrl Pts',(0.0871316433491625,-0.219198425104216,
-1.45222782877142));
#51438=CARTESIAN_POINT('Ctrl Pts',(0.231483862146741,-0.0453453044496629,
-1.43950855595043));
#51439=CARTESIAN_POINT('Ctrl Pts',(0.163401374080225,0.170114283366123,
-1.42678928312944));
#51440=CARTESIAN_POINT('Ctrl Pts',(-0.0546225385477825,0.229469265901282,
-1.41407001030846));
#51441=CARTESIAN_POINT('Ctrl Pts',(-0.185501093092507,0.1115929665413,-1.40415541197848));
#51442=CARTESIAN_POINT('Ctrl Pts',(-0.199439334922407,0.0226838977071687,
-1.39848057125551));
#51443=CARTESIAN_POINT('Ctrl Pts',(-0.199280157075849,0.000151800363860317,
-1.39704548813952));
#51444=CARTESIAN_POINT('Origin',(5.69858952725515E-17,8.58067791224701E-18,
-0.0149499999999998));
#51445=CARTESIAN_POINT('',(-0.0796899944392906,0.231730462577249,-0.0149499999999998));
#51446=CARTESIAN_POINT('Ctrl Pts',(0.197120359334095,-0.0326678654691807,
-0.0149499999999996));
#51447=CARTESIAN_POINT('Ctrl Pts',(0.198391584513283,-0.0282478211509381,
-0.0149499999999996));
#51448=CARTESIAN_POINT('Ctrl Pts',(0.199497230955055,-0.0237887632912905,
-0.0149499999999994));
#51449=CARTESIAN_POINT('Ctrl Pts',(0.200432280241851,-0.0192980722140279,
-0.0149499999999992));
#51450=CARTESIAN_POINT('Ctrl Pts',(0.202577210314895,-0.00899677743053964,
-0.014949999999999));
#51451=CARTESIAN_POINT('Ctrl Pts',(0.203826056148701,0.00147035978450179,
-0.014949999999999));
#51452=CARTESIAN_POINT('Ctrl Pts',(0.204234176055474,0.012009143396064,
-0.014949999999999));
#51453=CARTESIAN_POINT('Ctrl Pts',(0.204460723116552,0.0178592144534165,
-0.014949999999999));
#51454=CARTESIAN_POINT('Ctrl Pts',(0.20442720843244,0.0237345702014736,
-0.0149499999999995));
#51455=CARTESIAN_POINT('Ctrl Pts',(0.204142818256796,0.02959475413324,-0.0149499999999996));
#51456=CARTESIAN_POINT('Ctrl Pts',(0.203701771739557,0.03868302065875,-0.0149499999999997));
#51457=CARTESIAN_POINT('Ctrl Pts',(0.202658984688022,0.0477465139947516,
-0.0149499999999992));
#51458=CARTESIAN_POINT('Ctrl Pts',(0.201046156693127,0.0567277105127938,
-0.014949999999999));
#51459=CARTESIAN_POINT('Ctrl Pts',(0.200183599069131,0.061530950259233,
-0.0149499999999989));
#51460=CARTESIAN_POINT('Ctrl Pts',(0.199157809647221,0.0663107083864419,
-0.0149499999999991));
#51461=CARTESIAN_POINT('Ctrl Pts',(0.19797238261792,0.0710583673294022,
-0.0149499999999992));
#51462=CARTESIAN_POINT('Ctrl Pts',(0.196938500061177,0.0751990876311717,
-0.0149499999999992));
#51463=CARTESIAN_POINT('Ctrl Pts',(0.195783593393406,0.079312838501636,
-0.014949999999999));
#51464=CARTESIAN_POINT('Ctrl Pts',(0.194513872543076,0.0833835575473151,
-0.0149499999999991));
#51465=CARTESIAN_POINT('Ctrl Pts',(0.190330656324442,0.0967949289751111,
-0.0149499999999993));
#51466=CARTESIAN_POINT('Ctrl Pts',(0.184897520196834,0.109771278820074,
-0.0149499999999998));
#51467=CARTESIAN_POINT('Ctrl Pts',(0.178311313802482,0.12211617811317,-0.0149499999999997));
#51468=CARTESIAN_POINT('Ctrl Pts',(0.173661048230523,0.130832433987144,
-0.0149499999999997));
#51469=CARTESIAN_POINT('Ctrl Pts',(0.168434777087133,0.139234261100576,
-0.0149499999999995));
#51470=CARTESIAN_POINT('Ctrl Pts',(0.16265144281701,0.147249217570727,-0.0149499999999996));
#51471=CARTESIAN_POINT('Ctrl Pts',(0.160514169925959,0.150211202541075,
-0.0149499999999997));
#51472=CARTESIAN_POINT('Ctrl Pts',(0.158302456051775,0.153117610750161,
-0.0149499999999994));
#51473=CARTESIAN_POINT('Ctrl Pts',(0.156022862593314,0.155958527256897,
-0.0149499999999994));
#51474=CARTESIAN_POINT('Ctrl Pts',(0.150502215199784,0.162838569068711,
-0.0149499999999995));
#51475=CARTESIAN_POINT('Ctrl Pts',(0.144575729488352,0.169346199310948,
-0.0149499999999991));
#51476=CARTESIAN_POINT('Ctrl Pts',(0.138263937757876,0.175434414556545,
-0.0149499999999992));
#51477=CARTESIAN_POINT('Ctrl Pts',(0.131281545757466,0.182169476048256,
-0.0149499999999993));
#51478=CARTESIAN_POINT('Ctrl Pts',(0.123827770680868,0.188391667069538,
-0.0149499999999997));
#51479=CARTESIAN_POINT('Ctrl Pts',(0.115968513453136,0.194097818772095,
-0.0149499999999997));
#51480=CARTESIAN_POINT('Ctrl Pts',(0.111698380331938,0.197198115234424,
-0.0149499999999997));
#51481=CARTESIAN_POINT('Ctrl Pts',(0.107308365134894,0.200145943520289,
-0.0149499999999997));
#51482=CARTESIAN_POINT('Ctrl Pts',(0.102807943122472,0.202939758658773,
-0.0149499999999997));
#51483=CARTESIAN_POINT('Ctrl Pts',(0.0986065241053424,0.20554795585023,
-0.0149499999999998));
#51484=CARTESIAN_POINT('Ctrl Pts',(0.0943067130227581,0.208022653727126,
-0.0149500000000002));
#51485=CARTESIAN_POINT('Ctrl Pts',(0.0899371597296005,0.210351797381489,
-0.0149500000000001));
#51486=CARTESIAN_POINT('Ctrl Pts',(0.0771241543606563,0.217181632869509,
-0.0149499999999997));
#51487=CARTESIAN_POINT('Ctrl Pts',(0.063678628286122,0.222786554309641,
-0.0149499999999996));
#51488=CARTESIAN_POINT('Ctrl Pts',(0.0498091452572496,0.227155755310556,
-0.0149499999999995));
#51489=CARTESIAN_POINT('Ctrl Pts',(0.0425067586415354,0.229456172337205,
-0.0149499999999994));
#51490=CARTESIAN_POINT('Ctrl Pts',(0.0350861724152127,0.231413431882226,
-0.0149499999999995));
#51491=CARTESIAN_POINT('Ctrl Pts',(0.0275745532422898,0.233021449591895,
-0.0149499999999995));
#51492=CARTESIAN_POINT('Ctrl Pts',(0.0230174457248419,0.233996992870145,
-0.0149499999999994));
#51493=CARTESIAN_POINT('Ctrl Pts',(0.0184267979876164,0.234843932724277,
-0.0149499999999994));
#51494=CARTESIAN_POINT('Ctrl Pts',(0.0138084601729489,0.235560277476396,
-0.0149499999999995));
#51495=CARTESIAN_POINT('Ctrl Pts',(0.00959333086335831,0.236214081048503,
-0.0149499999999995));
#51496=CARTESIAN_POINT('Ctrl Pts',(0.00536398260013057,0.23675765141323,
-0.01495));
#51497=CARTESIAN_POINT('Ctrl Pts',(0.00112883840488462,0.237190302563417,
-0.01495));
#51498=CARTESIAN_POINT('Ctrl Pts',(-0.0140084017468552,0.238736683054937,
-0.01495));
#51499=CARTESIAN_POINT('Ctrl Pts',(-0.0292325594370678,0.238871969867428,
-0.0149499999999999));
#51500=CARTESIAN_POINT('Ctrl Pts',(-0.0443347582390812,0.237560856560192,
-0.0149499999999998));
#51501=CARTESIAN_POINT('Ctrl Pts',(-0.0562275002790541,0.236528375624631,
-0.0149499999999998));
#51502=CARTESIAN_POINT('Ctrl Pts',(-0.0680455254831802,0.234598199446658,
-0.0149499999999998));
#51503=CARTESIAN_POINT('Ctrl Pts',(-0.0796899944392906,0.231730462577249,
-0.0149499999999998));
#51504=CARTESIAN_POINT('',(-0.24505,-3.00099698131059E-17,-0.01495));
#51505=CARTESIAN_POINT('Origin',(0.,0.,-0.0149499999999999));
#51506=CARTESIAN_POINT('',(-0.231938272394163,0.0797165085725884,-0.0149499999999999));
#51507=CARTESIAN_POINT('Origin',(0.,0.,-0.0149499999999999));
#51508=CARTESIAN_POINT('Ctrl Pts',(-0.232146082211074,0.0797430227058928,
-0.0149499999999999));
#51509=CARTESIAN_POINT('Ctrl Pts',(-0.23350718091485,0.0743161424960959,
-0.0149499999999999));
#51510=CARTESIAN_POINT('Ctrl Pts',(-0.234667147495365,0.0688472522854195,
-0.01495));
#51511=CARTESIAN_POINT('Ctrl Pts',(-0.235618162261078,0.0633433287759428,
-0.01495));
#51512=CARTESIAN_POINT('Ctrl Pts',(-0.237412919095364,0.0529563140941966,
-0.01495));
#51513=CARTESIAN_POINT('Ctrl Pts',(-0.238464189863105,0.0424443716233503,
-0.0149500000000004));
#51514=CARTESIAN_POINT('Ctrl Pts',(-0.238796729904135,0.0318787064057965,
-0.0149500000000006));
#51515=CARTESIAN_POINT('Ctrl Pts',(-0.238949765616349,0.0270163623206224,
-0.0149500000000007));
#51516=CARTESIAN_POINT('Ctrl Pts',(-0.23895041575299,0.0221426647714983,
-0.0149500000000005));
#51517=CARTESIAN_POINT('Ctrl Pts',(-0.238800283436524,0.0172647976316243,
-0.0149500000000006));
#51518=CARTESIAN_POINT('Ctrl Pts',(-0.238643002975604,0.0121546840322981,
-0.0149500000000006));
#51519=CARTESIAN_POINT('Ctrl Pts',(-0.23832047459253,0.00704905816868219,
-0.0149500000000003));
#51520=CARTESIAN_POINT('Ctrl Pts',(-0.237836102473065,0.00195870824191732,
-0.0149500000000004));
#51521=CARTESIAN_POINT('Ctrl Pts',(-0.236971800239444,-0.00712439261134424,
-0.0149500000000004));
#51522=CARTESIAN_POINT('Ctrl Pts',(-0.235592455321206,-0.0161618930984169,
-0.0149500000000005));
#51523=CARTESIAN_POINT('Ctrl Pts',(-0.233711732266915,-0.0251065474147256,
-0.0149500000000005));
#51524=CARTESIAN_POINT('Ctrl Pts',(-0.232387572468453,-0.0314042059826735,
-0.0149500000000005));
#51525=CARTESIAN_POINT('Ctrl Pts',(-0.23081472952064,-0.0376558054885507,
-0.0149500000000003));
#51526=CARTESIAN_POINT('Ctrl Pts',(-0.228996206985243,-0.0438437591894054,
-0.0149500000000002));
#51527=CARTESIAN_POINT('Ctrl Pts',(-0.227643304056364,-0.0484473318824611,
-0.0149500000000002));
#51528=CARTESIAN_POINT('Ctrl Pts',(-0.226156739718812,-0.053007313491729,
-0.0149500000000003));
#51529=CARTESIAN_POINT('Ctrl Pts',(-0.22454077011411,-0.0575117245253547,
-0.0149500000000003));
#51530=CARTESIAN_POINT('Ctrl Pts',(-0.219610988257616,-0.0712531734505997,
-0.0149500000000004));
#51531=CARTESIAN_POINT('Ctrl Pts',(-0.213475163641887,-0.0844959724585875,
-0.0149500000000002));
#51532=CARTESIAN_POINT('Ctrl Pts',(-0.206180419574474,-0.0970381019544846,
-0.0149500000000001));
#51533=CARTESIAN_POINT('Ctrl Pts',(-0.202999702259208,-0.102506829587592,
-0.0149500000000001));
#51534=CARTESIAN_POINT('Ctrl Pts',(-0.1995981365692,-0.107841939337988,
-0.0149500000000007));
#51535=CARTESIAN_POINT('Ctrl Pts',(-0.195977488873056,-0.113024301602003,
-0.0149500000000007));
#51536=CARTESIAN_POINT('Ctrl Pts',(-0.193573372357027,-0.116465399371397,
-0.0149500000000008));
#51537=CARTESIAN_POINT('Ctrl Pts',(-0.191072637928957,-0.119839117844746,
-0.0149500000000006));
#51538=CARTESIAN_POINT('Ctrl Pts',(-0.188475540395292,-0.123139391550832,
-0.0149500000000006));
#51539=CARTESIAN_POINT('Ctrl Pts',(-0.185966800671422,-0.126327384161342,
-0.0149500000000005));
#51540=CARTESIAN_POINT('Ctrl Pts',(-0.183373622103193,-0.129439792556405,
-0.0149500000000006));
#51541=CARTESIAN_POINT('Ctrl Pts',(-0.180698977833861,-0.132470011526652,
-0.0149500000000007));
#51542=CARTESIAN_POINT('Ctrl Pts',(-0.175543672442891,-0.138310677656444,
-0.0149500000000007));
#51543=CARTESIAN_POINT('Ctrl Pts',(-0.170083732537213,-0.143849024363428,
-0.0149500000000004));
#51544=CARTESIAN_POINT('Ctrl Pts',(-0.164325057077125,-0.149051164015221,
-0.0149500000000004));
#51545=CARTESIAN_POINT('Ctrl Pts',(-0.153833964139055,-0.158528366011066,
-0.0149500000000006));
#51546=CARTESIAN_POINT('Ctrl Pts',(-0.142351798966231,-0.166892708688512,
-0.0149500000000005));
#51547=CARTESIAN_POINT('Ctrl Pts',(-0.130079353982082,-0.174080052076584,
-0.0149500000000005));
#51548=CARTESIAN_POINT('Ctrl Pts',(-0.125535338402389,-0.176741249610913,
-0.0149500000000005));
#51549=CARTESIAN_POINT('Ctrl Pts',(-0.120878764860052,-0.179242193486494,
-0.0149500000000003));
#51550=CARTESIAN_POINT('Ctrl Pts',(-0.116145470012991,-0.181566385959855,
-0.0149500000000003));
#51551=CARTESIAN_POINT('Ctrl Pts',(-0.104698292289123,-0.18718730017853,
-0.0149500000000001));
#51552=CARTESIAN_POINT('Ctrl Pts',(-0.0927779473770901,-0.191793807979919,
-0.0149500000000003));
#51553=CARTESIAN_POINT('Ctrl Pts',(-0.0805361235299436,-0.19534629546693,
-0.0149500000000004));
#51554=CARTESIAN_POINT('Ctrl Pts',(-0.0695096581407387,-0.198546094844067,
-0.0149500000000005));
#51555=CARTESIAN_POINT('Ctrl Pts',(-0.0582215533463788,-0.200890382869549,
-0.0149500000000003));
#51556=CARTESIAN_POINT('Ctrl Pts',(-0.0467843692613105,-0.202323848970006,
-0.0149500000000003));
#51557=CARTESIAN_POINT('Ctrl Pts',(-0.0426471414161356,-0.202842383586728,
-0.0149500000000003));
#51558=CARTESIAN_POINT('Ctrl Pts',(-0.0384978609908941,-0.203240430888916,
-0.0149500000000004));
#51559=CARTESIAN_POINT('Ctrl Pts',(-0.0343490018043639,-0.203515797544261,
-0.0149500000000004));
#51560=CARTESIAN_POINT('Ctrl Pts',(-0.0213910422852966,-0.204375838777875,
-0.0149500000000003));
#51561=CARTESIAN_POINT('Ctrl Pts',(-0.00841434859516882,-0.204045491679898,
-0.0149500000000002));
#51562=CARTESIAN_POINT('Ctrl Pts',(0.00441495196016681,-0.202455457095622,
-0.0149500000000002));
#51563=CARTESIAN_POINT('Ctrl Pts',(0.013943768462285,-0.201274477063217,
-0.0149500000000001));
#51564=CARTESIAN_POINT('Ctrl Pts',(0.0233913298848719,-0.199397633716378,
-0.0149500000000001));
#51565=CARTESIAN_POINT('Ctrl Pts',(0.0326814423280684,-0.196779569448551,
-0.01495));
#51566=CARTESIAN_POINT('Ctrl Pts',(-0.0648690538289174,-0.188632662814108,
-1.54126273851832));
#51567=CARTESIAN_POINT('Ctrl Pts',(-0.00205630422489446,-0.210233395022512,
-1.53702298091132));
#51568=CARTESIAN_POINT('Ctrl Pts',(0.14575417320045,-0.185369963268203,
-1.52854346569733));
#51569=CARTESIAN_POINT('Ctrl Pts',(0.234947663922723,0.022663611902651,
-1.51582419287635));
#51570=CARTESIAN_POINT('Ctrl Pts',(0.107989171190762,0.209631807114936,
-1.50310492005536));
#51571=CARTESIAN_POINT('Ctrl Pts',(-0.117789854919609,0.204361256460409,
-1.49038564723437));
#51572=CARTESIAN_POINT('Ctrl Pts',(-0.235621695359832,0.01148780516709,
-1.47766637441339));
#51573=CARTESIAN_POINT('Ctrl Pts',(-0.137157166917276,-0.191891750082203,
-1.4649471015924));
#51574=CARTESIAN_POINT('Ctrl Pts',(0.0871316433491625,-0.219198425104216,
-1.45222782877142));
#51575=CARTESIAN_POINT('Ctrl Pts',(0.231483862146741,-0.0453453044496629,
-1.43950855595043));
#51576=CARTESIAN_POINT('Ctrl Pts',(0.163401374080225,0.170114283366123,
-1.42678928312944));
#51577=CARTESIAN_POINT('Ctrl Pts',(-0.0546225385477825,0.229469265901282,
-1.41407001030846));
#51578=CARTESIAN_POINT('Ctrl Pts',(-0.222524453105232,0.0782477276413624,
-1.40135073748747));
#51579=CARTESIAN_POINT('Ctrl Pts',(-0.186222683554777,-0.144777986019408,
-1.38863146466649));
#51580=CARTESIAN_POINT('Ctrl Pts',(0.0209676361572253,-0.234946916486012,
-1.3759121918455));
#51581=CARTESIAN_POINT('Ctrl Pts',(0.208917198058643,-0.109513915389758,
-1.36319291902451));
#51582=CARTESIAN_POINT('Ctrl Pts',(0.205151275600481,0.116415675121088,
-1.35047364620353));
#51583=CARTESIAN_POINT('Ctrl Pts',(0.0131260573719064,0.235515146136983,
-1.33775437338254));
#51584=CARTESIAN_POINT('Ctrl Pts',(-0.190944500197199,0.138491419139472,
-1.32503510056156));
#51585=CARTESIAN_POINT('Ctrl Pts',(-0.219792619778126,-0.0856205274590762,
-1.31231582774057));
#51586=CARTESIAN_POINT('Ctrl Pts',(-0.0469455445028857,-0.231161825669147,
-1.29959655491958));
#51587=CARTESIAN_POINT('Ctrl Pts',(0.168981655819671,-0.164574825627453,
-1.2868772820986));
#51588=CARTESIAN_POINT('Ctrl Pts',(0.229840901678433,0.0530361437331597,
-1.27415800927761));
#51589=CARTESIAN_POINT('Ctrl Pts',(0.0797840170844622,0.22197789021412,
-1.26143873645663));
#51590=CARTESIAN_POINT('Ctrl Pts',(-0.143487584872076,0.187219085557888,
-1.24871946363564));
#51591=CARTESIAN_POINT('Ctrl Pts',(-0.235086162299716,-0.019343454534662,
-1.23600019081465));
#51592=CARTESIAN_POINT('Ctrl Pts',(-0.110955233724902,-0.208155252443532,
-1.22328091799367));
#51593=CARTESIAN_POINT('Ctrl Pts',(0.11499503466161,-0.20595100143569,-1.21056164517268));
#51594=CARTESIAN_POINT('Ctrl Pts',(0.235418793778872,-0.0147534578031819,
-1.19784237235169));
#51595=CARTESIAN_POINT('Ctrl Pts',(0.139807803503312,0.189982765195607,
-1.18512309953071));
#51596=CARTESIAN_POINT('Ctrl Pts',(-0.0840994171703575,0.220379130181726,
-1.17240382670972));
#51597=CARTESIAN_POINT('Ctrl Pts',(-0.230831845515026,0.0485420650925855,
-1.15968455388874));
#51598=CARTESIAN_POINT('Ctrl Pts',(-0.165738789974153,-0.167840181382976,
-1.14696528106775));
#51599=CARTESIAN_POINT('Ctrl Pts',(0.051446362342642,-0.230201965217191,
-1.13424600824677));
#51600=CARTESIAN_POINT('Ctrl Pts',(0.221421171676079,-0.0813162820208495,
-1.12152673542578));
#51601=CARTESIAN_POINT('Ctrl Pts',(0.188206309629664,0.142190217679984,
-1.10880746260479));
#51602=CARTESIAN_POINT('Ctrl Pts',(-0.0177182256432174,0.235214237384252,
-1.09608818978381));
#51603=CARTESIAN_POINT('Ctrl Pts',(-0.207383428447063,0.112391221159588,
-1.08336891696282));
#51604=CARTESIAN_POINT('Ctrl Pts',(-0.206740855544523,-0.113568884985925,
-1.07064964414184));
#51605=CARTESIAN_POINT('Ctrl Pts',(-0.0163801713107981,-0.235311204527198,
-1.05793037132085));
#51606=CARTESIAN_POINT('Ctrl Pts',(0.189011964525323,-0.141117505131332,
-1.04521109849986));
#51607=CARTESIAN_POINT('Ctrl Pts',(0.22095510870339,0.0825742873180875,
-1.03249182567888));
#51608=CARTESIAN_POINT('Ctrl Pts',(0.0501362695194371,0.230490840310171,
-1.01977255285789));
#51609=CARTESIAN_POINT('Ctrl Pts',(-0.166690690978327,0.16689483673674,
-1.00705328003691));
#51610=CARTESIAN_POINT('Ctrl Pts',(-0.230552031857313,-0.0498541231462333,
-0.99433400721592));
#51611=CARTESIAN_POINT('Ctrl Pts',(-0.0828446630474759,-0.220853876562684,
-0.981614734394935));
#51612=CARTESIAN_POINT('Ctrl Pts',(0.140886058601026,-0.189184543449203,
-0.968895461573948));
#51613=CARTESIAN_POINT('Ctrl Pts',(0.23533107675241,0.0160921503462616,
-0.956176188752962));
#51614=CARTESIAN_POINT('Ctrl Pts',(0.113821839991816,0.206601698272528,
-0.943456915931977));
#51615=CARTESIAN_POINT('Ctrl Pts',(-0.112137310428092,0.20752083413038,
-0.93073764311099));
#51616=CARTESIAN_POINT('Ctrl Pts',(-0.235192375014876,0.0180061023843909,
-0.918018370290004));
#51617=CARTESIAN_POINT('Ctrl Pts',(-0.142420465925963,-0.188032135215358,
-0.905299097469019));
#51618=CARTESIAN_POINT('Ctrl Pts',(0.0810452130963459,-0.22152053273316,
-0.892579824648032));
#51619=CARTESIAN_POINT('Ctrl Pts',(0.230138825114443,-0.0517280790592424,
-0.879860551827046));
#51620=CARTESIAN_POINT('Ctrl Pts',(0.168042911338648,0.165533238163961,
-0.86714127900606));
#51621=CARTESIAN_POINT('Ctrl Pts',(-0.0482595025397965,0.230891085585448,
-0.854422006185075));
#51622=CARTESIAN_POINT('Ctrl Pts',(-0.220276031794642,0.0843690867855101,
-0.841702733364088));
#51623=CARTESIAN_POINT('Ctrl Pts',(-0.190153740381844,-0.139575169736631,
-0.828983460543103));
#51624=CARTESIAN_POINT('Ctrl Pts',(0.0144653063663763,-0.235436674925429,
-0.816264187722117));
#51625=CARTESIAN_POINT('Ctrl Pts',(0.205810099235619,-0.115247021830672,
-0.80354491490113));
#51626=CARTESIAN_POINT('Ctrl Pts',(0.208290899949043,0.110700379342769,
-0.790825642080145));
#51627=CARTESIAN_POINT('Ctrl Pts',(0.019631173350109,0.235062310932895,
-0.778106369259159));
#51628=CARTESIAN_POINT('Ctrl Pts',(-0.187043324066072,0.143716623640167,
-0.765387096438172));
#51629=CARTESIAN_POINT('Ctrl Pts',(-0.222075375264048,-0.0795122675412271,
-0.752667823617187));
#51630=CARTESIAN_POINT('Ctrl Pts',(-0.0533174176740989,-0.229775816744889,
-0.739948550796201));
#51631=CARTESIAN_POINT('Ctrl Pts',(0.164367878228055,-0.169182958938016,
-0.727229277975214));
#51632=CARTESIAN_POINT('Ctrl Pts',(0.231219110206101,0.0466625766939018,
-0.714510005154229));
#51633=CARTESIAN_POINT('Ctrl Pts',(0.085889480416779,0.219687664974506,
-0.701790732333243));
#51634=CARTESIAN_POINT('Ctrl Pts',(-0.138257613704705,0.191113854131237,
-0.689071459512257));
#51635=CARTESIAN_POINT('Ctrl Pts',(-0.235531026859181,-0.0128377714138675,
-0.676352186691271));
#51636=CARTESIAN_POINT('Ctrl Pts',(-0.116666698598652,-0.205008669149152,
-0.663632913870284));
#51637=CARTESIAN_POINT('Ctrl Pts',(0.109258160368663,-0.209051016216307,
-0.650913641049299));
#51638=CARTESIAN_POINT('Ctrl Pts',(0.234921018494109,-0.0212553065822581,
-0.638194368228312));
#51639=CARTESIAN_POINT('Ctrl Pts',(0.145005916359623,0.186045578310588,
-0.625475095407328));
#51640=CARTESIAN_POINT('Ctrl Pts',(-0.0779755238778273,0.222619609792564,
-0.612755822586341));
#51641=CARTESIAN_POINT('Ctrl Pts',(-0.229401832541543,0.0549042094451505,
-0.600036549765355));
#51642=CARTESIAN_POINT('Ctrl Pts',(-0.17031492507753,-0.163194666837034,
-0.587317276944369));
#51643=CARTESIAN_POINT('Ctrl Pts',(0.0450634218898312,-0.231536090050329,
-0.574598004123383));
#51644=CARTESIAN_POINT('Ctrl Pts',(0.219088804207135,-0.0874057713157602,
-0.561878731302397));
#51645=CARTESIAN_POINT('Ctrl Pts',(0.192064838835073,0.136933453441709,
-0.54915945848141));
#51646=CARTESIAN_POINT('Ctrl Pts',(-0.0112096232321388,0.235614128046703,
-0.536440185660426));
#51647=CARTESIAN_POINT('Ctrl Pts',(-0.204197446295501,0.118080802481237,
-0.523720912839439));
#51648=CARTESIAN_POINT('Ctrl Pts',(-0.209801146623257,-0.10781072239708,
-0.511001640018453));
#51649=CARTESIAN_POINT('Ctrl Pts',(-0.0228784244999453,-0.234768504447706,
-0.498282367197467));
#51650=CARTESIAN_POINT('Ctrl Pts',(0.185038945608821,-0.146288282497961,
-0.485563094376481));
#51651=CARTESIAN_POINT('Ctrl Pts',(0.223153210321907,0.0764350555126916,
-0.472843821555495));
#51652=CARTESIAN_POINT('Ctrl Pts',(0.0564883785752809,0.229016890368669,
-0.46012454873451));
#51653=CARTESIAN_POINT('Ctrl Pts',(-0.162013660032506,0.171438755686017,
-0.447405275913523));
#51654=CARTESIAN_POINT('Ctrl Pts',(-0.231842009976495,-0.0434621145155262,
-0.434686003092537));
#51655=CARTESIAN_POINT('Ctrl Pts',(-0.0889178870534499,-0.21847947809828,
-0.421966730271551));
#51656=CARTESIAN_POINT('Ctrl Pts',(0.135602752200584,-0.193006649067832,
-0.409247457450565));
#51657=CARTESIAN_POINT('Ctrl Pts',(0.235685974516513,0.00958093959523976,
-0.396528184629579));
#51658=CARTESIAN_POINT('Ctrl Pts',(0.119489265933811,0.20337646942222,-0.383808911808593));
#51659=CARTESIAN_POINT('Ctrl Pts',(-0.106358134575664,0.210541255342925,
-0.371089638987607));
#51660=CARTESIAN_POINT('Ctrl Pts',(-0.234604776065496,0.0245004495613401,
-0.358370366166621));
#51661=CARTESIAN_POINT('Ctrl Pts',(-0.147563660825225,-0.184023474027218,
-0.345651093345635));
#51662=CARTESIAN_POINT('Ctrl Pts',(0.0748909360789789,-0.223676151397489,
-0.332931820524649));
#51663=CARTESIAN_POINT('Ctrl Pts',(0.228621008521177,-0.0580698493273639,
-0.320212547703664));
#51664=CARTESIAN_POINT('Ctrl Pts',(0.172554397257742,0.160824914104033,
-0.307493274882677));
#51665=CARTESIAN_POINT('Ctrl Pts',(-0.0418587313987176,0.232136855608358,
-0.294774002061692));
#51666=CARTESIAN_POINT('Ctrl Pts',(-0.217859715111443,0.0904257549484663,
-0.282054729240705));
#51667=CARTESIAN_POINT('Ctrl Pts',(-0.193939241065975,-0.134265572685697,
-0.26933545641972));
#51668=CARTESIAN_POINT('Ctrl Pts',(0.00795180063483016,-0.23574656447556,
-0.256616183598734));
#51669=CARTESIAN_POINT('Ctrl Pts',(0.202545773298689,-0.12089201855432,
-0.243896910777748));
#51670=CARTESIAN_POINT('Ctrl Pts',(0.211271315496057,0.10490046033926,-0.231177637956761));
#51671=CARTESIAN_POINT('Ctrl Pts',(0.0261212881376767,0.234429852510476,
-0.218458365135776));
#51672=CARTESIAN_POINT('Ctrl Pts',(-0.182999181298496,0.148831968805373,
-0.20573909231479));
#51673=CARTESIAN_POINT('Ctrl Pts',(-0.224188466684687,-0.0733431981456951,
-0.193019819493804));
#51674=CARTESIAN_POINT('Ctrl Pts',(-0.0596484344001499,-0.228214284403755,
-0.180300546672818));
#51675=CARTESIAN_POINT('Ctrl Pts',(0.159628272860435,-0.173661646916563,
-0.167581273851832));
#51676=CARTESIAN_POINT('Ctrl Pts',(0.232421018722115,0.0402530640696309,
-0.154862001030846));
#51677=CARTESIAN_POINT('Ctrl Pts',(0.0919285295363725,0.217230088081641,
-0.14214272820986));
#51678=CARTESIAN_POINT('Ctrl Pts',(-0.132920504851494,0.194861535061435,
-0.129423455388874));
#51679=CARTESIAN_POINT('Ctrl Pts',(-0.235798703843206,-0.00632031137431454,
-0.116704182567888));
#51680=CARTESIAN_POINT('Ctrl Pts',(-0.122283640616722,-0.201709157150624,
-0.103984909746902));
#51681=CARTESIAN_POINT('Ctrl Pts',(0.10342756844873,-0.21198412740384,-0.091265636925916));
#51682=CARTESIAN_POINT('Ctrl Pts',(0.234263184552909,-0.0277545195405686,
-0.0785463641049296));
#51683=CARTESIAN_POINT('Ctrl Pts',(0.150056069810251,0.181992167351128,
-0.0658270912839439));
#51684=CARTESIAN_POINT('Ctrl Pts',(-0.0717210418700825,0.224640263091484,
-0.0531078184629578));
#51685=CARTESIAN_POINT('Ctrl Pts',(-0.227933705557797,0.0613210400915578,
-0.040388545641972));
#51686=CARTESIAN_POINT('Ctrl Pts',(-0.174482868217891,-0.158625442429202,
-0.0276692728209859));
#51687=CARTESIAN_POINT('Ctrl Pts',(-0.0328441439546209,-0.207662155862942,
-0.0191897576069953));
#51688=CARTESIAN_POINT('Ctrl Pts',(0.0326814423280684,-0.196779569448551,
-0.01495));
#51689=CARTESIAN_POINT('Ctrl Pts',(-0.0698093673657081,-0.202998596068489,
-1.53249182567888));
#51690=CARTESIAN_POINT('Ctrl Pts',(-0.00221290875353342,-0.226244402213306,
-1.52825206807188));
#51691=CARTESIAN_POINT('Ctrl Pts',(0.156854555777397,-0.199487415039017,
-1.51977255285789));
#51692=CARTESIAN_POINT('Ctrl Pts',(0.252840866551755,0.0243896328951931,
-1.50705328003691));
#51693=CARTESIAN_POINT('Ctrl Pts',(0.116213437351133,0.225596998424227,
-1.49433400721592));
#51694=CARTESIAN_POINT('Ctrl Pts',(-0.126760523989183,0.219925051861978,
-1.48161473439493));
#51695=CARTESIAN_POINT('Ctrl Pts',(-0.253566231042706,0.0123626962904411,
-1.46889546157395));
#51696=CARTESIAN_POINT('Ctrl Pts',(-0.147602816551325,-0.2065058897154,
-1.45617618875296));
#51697=CARTESIAN_POINT('Ctrl Pts',(0.0937674367161456,-0.235892193285902,
-1.44345691593198));
#51698=CARTESIAN_POINT('Ctrl Pts',(0.249113267698544,-0.0487987234249642,
-1.43073764311099));
#51699=CARTESIAN_POINT('Ctrl Pts',(0.175845736571276,0.183069889272311,
-1.41801837029));
#51700=CARTESIAN_POINT('Ctrl Pts',(-0.0587824954251087,0.24694524333112,
-1.40529909746902));
#51701=CARTESIAN_POINT('Ctrl Pts',(-0.239471525754721,0.084206937546123,
-1.39257982464803));
#51702=CARTESIAN_POINT('Ctrl Pts',(-0.200405077009279,-0.155804023890208,
-1.37986055182705));
#51703=CARTESIAN_POINT('Ctrl Pts',(0.0225644946070967,-0.252840062191573,
-1.36714127900606));
#51704=CARTESIAN_POINT('Ctrl Pts',(0.224827965993676,-0.117854303398096,
-1.35442200618508));
#51705=CARTESIAN_POINT('Ctrl Pts',(0.220775237476226,0.125281689063758,
-1.34170273336409));
#51706=CARTESIAN_POINT('Ctrl Pts',(0.0141257149141647,0.253451567217642,
-1.3289834605431));
#51707=CARTESIAN_POINT('Ctrl Pts',(-0.205486498938039,0.149038683086135,
-1.31626418772212));
#51708=CARTESIAN_POINT('Ctrl Pts',(-0.236531640785584,-0.0921412368862326,
-1.30354491490113));
#51709=CARTESIAN_POINT('Ctrl Pts',(-0.0505208349581985,-0.248766705486787,
-1.29082564208014));
#51710=CARTESIAN_POINT('Ctrl Pts',(0.181851002795451,-0.177108556133318,
-1.27810636925916));
#51711=CARTESIAN_POINT('Ctrl Pts',(0.247345182238226,0.0570752835595998,
-1.26538709643817));
#51712=CARTESIAN_POINT('Ctrl Pts',(0.0858602281027615,0.238883337590998,
-1.25266782361719));
#51713=CARTESIAN_POINT('Ctrl Pts',(-0.154415348051328,0.201477363243982,
-1.2399485507962));
#51714=CARTESIAN_POINT('Ctrl Pts',(-0.252989912722593,-0.020816618156529,
-1.22722927797522));
#51715=CARTESIAN_POINT('Ctrl Pts',(-0.119405390013515,-0.224007991934886,
-1.21451000515423));
#51716=CARTESIAN_POINT('Ctrl Pts',(0.123752855114802,-0.221635869030513,
-1.20179073233324));
#51717=CARTESIAN_POINT('Ctrl Pts',(0.253347876832675,-0.0158770553122787,
-1.18907145951226));
#51718=CARTESIAN_POINT('Ctrl Pts',(0.15045532097779,0.204451519882976,-1.17635218669127));
#51719=CARTESIAN_POINT('Ctrl Pts',(-0.0905042815017902,0.237162818794389,
-1.16363291387028));
#51720=CARTESIAN_POINT('Ctrl Pts',(-0.248411594622011,0.0522389437600805,
-1.1509136410493));
#51721=CARTESIAN_POINT('Ctrl Pts',(-0.178361165966253,-0.180622595664678,
-1.13819436822831));
#51722=CARTESIAN_POINT('Ctrl Pts',(0.0553644272025067,-0.247733743743779,
-1.12547509540733));
#51723=CARTESIAN_POINT('Ctrl Pts',(0.238284220344061,-0.0875091876533035,
-1.11275582258634));
#51724=CARTESIAN_POINT('Ctrl Pts',(0.202539772572176,0.153019175645918,
-1.10003654976536));
#51725=CARTESIAN_POINT('Ctrl Pts',(-0.0190676146789165,0.253127741781273,
-1.08731727694437));
#51726=CARTESIAN_POINT('Ctrl Pts',(-0.223177387174513,0.120950739736435,
-1.07459800412338));
#51727=CARTESIAN_POINT('Ctrl Pts',(-0.222485877045032,-0.122218092377381,
-1.0618787313024));
#51728=CARTESIAN_POINT('Ctrl Pts',(-0.0176276564718308,-0.253232093772011,
-1.04915945848141));
#51729=CARTESIAN_POINT('Ctrl Pts',(0.203406784733772,-0.151864767188167,
-1.03644018566043));
#51730=CARTESIAN_POINT('Ctrl Pts',(0.237782662831572,0.0888630004308762,
-1.02372091283944));
#51731=CARTESIAN_POINT('Ctrl Pts',(0.053954560004209,0.248044619057944,
-1.01100164001845));
#51732=CARTESIAN_POINT('Ctrl Pts',(-0.179385562083873,0.179605255225736,
-0.998282367197467));
#51733=CARTESIAN_POINT('Ctrl Pts',(-0.248110470846155,-0.0536509258573303,
-0.98556309437648));
#51734=CARTESIAN_POINT('Ctrl Pts',(-0.0891539675023196,-0.237673721028313,
-0.972843821555496));
#51735=CARTESIAN_POINT('Ctrl Pts',(0.151615694095433,-0.203592506966266,
-0.960124548734509));
#51736=CARTESIAN_POINT('Ctrl Pts',(0.253253479431093,0.0173177003350314,
-0.947405275913524));
#51737=CARTESIAN_POINT('Ctrl Pts',(0.122490311993534,0.222336121798901,
-0.934686003092538));
#51738=CARTESIAN_POINT('Ctrl Pts',(-0.120677491608289,0.22332525743404,
-0.92196673027155));
#51739=CARTESIAN_POINT('Ctrl Pts',(-0.253104214412132,0.0193774156085542,
-0.909247457450568));
#51740=CARTESIAN_POINT('Ctrl Pts',(-0.15326695919509,-0.202352333339499,
-0.896528184629577));
#51741=CARTESIAN_POINT('Ctrl Pts',(0.087217474594219,-0.238391148565243,
-0.883808911808594));
#51742=CARTESIAN_POINT('Ctrl Pts',(0.24766579500138,-0.0556675989708875,
-0.871089638987607));
#51743=CARTESIAN_POINT('Ctrl Pts',(0.180840765178744,0.17813995969017,-0.858370366166622));
#51744=CARTESIAN_POINT('Ctrl Pts',(-0.0519348617381085,0.248475346312451,
-0.845651093345635));
#51745=CARTESIAN_POINT('Ctrl Pts',(-0.237051868614696,0.0907944886825747,
-0.83293182052465));
#51746=CARTESIAN_POINT('Ctrl Pts',(-0.204635516239977,-0.150204970230839,
-0.820212547703662));
#51747=CARTESIAN_POINT('Ctrl Pts',(0.0155669587666708,-0.253367119776039,
-0.807493274882678));
#51748=CARTESIAN_POINT('Ctrl Pts',(0.22148423596564,-0.124024033185368,
-0.794774002061692));
#51749=CARTESIAN_POINT('Ctrl Pts',(0.224153970116863,0.119131126367953,
-0.782054729240706));
#51750=CARTESIAN_POINT('Ctrl Pts',(0.0211262491330936,0.252964244877444,
-0.769335456419719));
#51751=CARTESIAN_POINT('Ctrl Pts',(-0.201288216064753,0.154661830010893,
-0.756616183598734));
#51752=CARTESIAN_POINT('Ctrl Pts',(-0.238988246931607,-0.0855677825902145,
-0.743896910777748));
#51753=CARTESIAN_POINT('Ctrl Pts',(-0.0573779788313004,-0.247275140550125,
-0.731177637956761));
#51754=CARTESIAN_POINT('Ctrl Pts',(0.176885847982398,-0.182067636806757,
-0.718458365135776));
#51755=CARTESIAN_POINT('Ctrl Pts',(0.248828352713755,0.0502163168164291,
-0.705739092314789));
#51756=CARTESIAN_POINT('Ctrl Pts',(0.0924306728301907,0.236418692807924,
-0.693019819493804));
#51757=CARTESIAN_POINT('Ctrl Pts',(-0.148787071438908,0.205668750571112,
-0.680300546672817));
#51758=CARTESIAN_POINT('Ctrl Pts',(-0.253468657387831,-0.0138154736024218,
-0.667581273851832));
#51759=CARTESIAN_POINT('Ctrl Pts',(-0.125551830049769,-0.220621770367303,
-0.654862001030845));
#51760=CARTESIAN_POINT('Ctrl Pts',(0.117579070522484,-0.224971975507879,
-0.64214272820986));
#51761=CARTESIAN_POINT('Ctrl Pts',(0.25281219185396,-0.0228740735079175,
-0.629423455388874));
#51762=CARTESIAN_POINT('Ctrl Pts',(0.156049313005971,0.200214483739847,
-0.616704182567888));
#51763=CARTESIAN_POINT('Ctrl Pts',(-0.0839140032206536,0.239573929408717,
-0.603984909746902));
#51764=CARTESIAN_POINT('Ctrl Pts',(-0.246872674364797,0.0590856178847445,
-0.591265636925916));
#51765=CARTESIAN_POINT('Ctrl Pts',(-0.183285811505085,-0.175623286866439,
-0.57854636410493));
#51766=CARTESIAN_POINT('Ctrl Pts',(0.0484953731830222,-0.249169473187805,
-0.565827091283944));
#51767=CARTESIAN_POINT('Ctrl Pts',(0.235774223853273,-0.0940624417886129,
-0.553107818462958));
#51768=CARTESIAN_POINT('Ctrl Pts',(0.206692160604566,0.147362065449236,
-0.540388545641972));
#51769=CARTESIAN_POINT('Ctrl Pts',(-0.0120633285064898,0.253558087416263,
-0.527669272820986));
#51770=CARTESIAN_POINT('Ctrl Pts',(-0.219748766201783,0.127073629607583,
-0.51495));
#51771=CARTESIAN_POINT('Ctrl Pts',(-0.225779234532946,-0.116021398209831,
-0.502230727179014));
#51772=CARTESIAN_POINT('Ctrl Pts',(-0.024620805243708,-0.252648062604875,
-0.489511454358028));
#51773=CARTESIAN_POINT('Ctrl Pts',(0.199131187654392,-0.157429341903644,
-0.476792181537042));
#51774=CARTESIAN_POINT('Ctrl Pts',(0.2401481680199,0.0822562154825955,-0.464072908716056));
#51775=CARTESIAN_POINT('Ctrl Pts',(0.0607904345615275,0.246458415670172,
-0.45135363589507));
#51776=CARTESIAN_POINT('Ctrl Pts',(-0.174352336651932,0.18449523108459,
-0.438634363074084));
#51777=CARTESIAN_POINT('Ctrl Pts',(-0.249498691439802,-0.0467721130434017,
-0.425915090253098));
#51778=CARTESIAN_POINT('Ctrl Pts',(-0.0956897176127717,-0.235118492535058,
-0.413195817432112));
#51779=CARTESIAN_POINT('Ctrl Pts',(0.145930020331997,-0.207705697455295,
-0.400476544611126));
#51780=CARTESIAN_POINT('Ctrl Pts',(0.253635405587391,0.0103106071760593,
-0.38775727179014));
#51781=CARTESIAN_POINT('Ctrl Pts',(0.128589359170113,0.218865265167579,
-0.375037998969154));
#51782=CARTESIAN_POINT('Ctrl Pts',(-0.114458183843801,0.226575708636578,
-0.362318726148168));
#51783=CARTESIAN_POINT('Ctrl Pts',(-0.252471864955808,0.0263663608931849,
-0.349599453327182));
#51784=CARTESIAN_POINT('Ctrl Pts',(-0.158801850810788,-0.198038379535493,
-0.336880180506196));
#51785=CARTESIAN_POINT('Ctrl Pts',(0.0805944986169714,-0.240710935371991,
-0.32416090768521));
#51786=CARTESIAN_POINT('Ctrl Pts',(0.246032384154468,-0.0624923473565169,
-0.311441634864224));
#51787=CARTESIAN_POINT('Ctrl Pts',(0.185695837964635,0.173073057915355,
-0.298722362043239));
#51788=CARTESIAN_POINT('Ctrl Pts',(-0.0450466190763633,0.249815991998634,
-0.286003089222252));
#51789=CARTESIAN_POINT('Ctrl Pts',(-0.234451529484512,0.0973124220859982,
-0.273283816401267));
#51790=CARTESIAN_POINT('Ctrl Pts',(-0.208709314026801,-0.14449100356701,
-0.26056454358028));
#51791=CARTESIAN_POINT('Ctrl Pts',(0.00855739584547627,-0.25370060997161,
-0.247845270759295));
#51792=CARTESIAN_POINT('Ctrl Pts',(0.217971304682049,-0.130098942973611,
-0.235125997938309));
#51793=CARTESIAN_POINT('Ctrl Pts',(0.227361368892445,0.112889495690325,
-0.222406725117322));
#51794=CARTESIAN_POINT('Ctrl Pts',(0.0281106396969799,0.252283619529175,
-0.209687452296337));
#51795=CARTESIAN_POINT('Ctrl Pts',(-0.196936078466359,0.160166750905562,
-0.196968179475351));
#51796=CARTESIAN_POINT('Ctrl Pts',(-0.241262267694262,-0.0789288876731861,
-0.184248906654365));
#51797=CARTESIAN_POINT('Ctrl Pts',(-0.0641911547039274,-0.245594684640545,
-0.171529633833379));
#51798=CARTESIAN_POINT('Ctrl Pts',(0.171785282570279,-0.186887413818386,
-0.158810361012393));
#51799=CARTESIAN_POINT('Ctrl Pts',(0.250121796477491,0.0433186669354408,
-0.146091088191407));
#51800=CARTESIAN_POINT('Ctrl Pts',(0.0989296453547647,0.233773951162762,
-0.133371815370421));
#51801=CARTESIAN_POINT('Ctrl Pts',(-0.143043497722123,0.209701848317776,
-0.120652542549435));
#51802=CARTESIAN_POINT('Ctrl Pts',(-0.253756720182186,-0.00680165522004821,
-0.107933269728449));
#51803=CARTESIAN_POINT('Ctrl Pts',(-0.131596548535188,-0.217070973313282,
-0.0952139969074629));
#51804=CARTESIAN_POINT('Ctrl Pts',(0.111304430932834,-0.228128467306803,
-0.0824947240864769));
#51805=CARTESIAN_POINT('Ctrl Pts',(0.25210425843184,-0.0298682551432968,
-0.0697754512654907));
#51806=CARTESIAN_POINT('Ctrl Pts',(0.161484077299248,0.195852372100306,
-0.0570561784445048));
#51807=CARTESIAN_POINT('Ctrl Pts',(-0.0771831908164463,0.241748472124187,
-0.0443369056235189));
#51808=CARTESIAN_POINT('Ctrl Pts',(-0.245292737401046,0.0659911431156193,
-0.0316176328025329));
#51809=CARTESIAN_POINT('Ctrl Pts',(-0.187771177895848,-0.170706078329624,
-0.018898359981547));
#51810=CARTESIAN_POINT('Ctrl Pts',(-0.0353454964394484,-0.223477341982261,
-0.0104188447675563));
#51811=CARTESIAN_POINT('Ctrl Pts',(0.0351704037419476,-0.211765956844829,
-0.006179087160561));
#51812=CARTESIAN_POINT('Ctrl Pts',(-0.0747496809024987,-0.217364529322869,
-1.52372091283944));
#51813=CARTESIAN_POINT('Ctrl Pts',(-0.00236951328217214,-0.2422554094041,
-1.51948115523244));
#51814=CARTESIAN_POINT('Ctrl Pts',(0.167954938354344,-0.213604866809831,
-1.51100164001845));
#51815=CARTESIAN_POINT('Ctrl Pts',(0.270734069180786,0.0261156538877355,
-1.49828236719747));
#51816=CARTESIAN_POINT('Ctrl Pts',(0.124437703511504,0.241562189733518,
-1.48556309437648));
#51817=CARTESIAN_POINT('Ctrl Pts',(-0.135731193058758,0.235488847263547,
-1.47284382155549));
#51818=CARTESIAN_POINT('Ctrl Pts',(-0.271510766725581,0.0132375874137922,
-1.46012454873451));
#51819=CARTESIAN_POINT('Ctrl Pts',(-0.158048466185375,-0.221120029348596,
-1.44740527591352));
#51820=CARTESIAN_POINT('Ctrl Pts',(0.100403230083129,-0.252585961467587,
-1.43468600309254));
#51821=CARTESIAN_POINT('Ctrl Pts',(0.266742673250346,-0.0522521424002653,
-1.42196673027155));
#51822=CARTESIAN_POINT('Ctrl Pts',(0.188290099062327,0.196025495178498,
-1.40924745745057));
#51823=CARTESIAN_POINT('Ctrl Pts',(-0.062942452302435,0.264421220760959,
-1.39652818462958));
#51824=CARTESIAN_POINT('Ctrl Pts',(-0.25641859840421,0.0901661474508833,
-1.38380891180859));
#51825=CARTESIAN_POINT('Ctrl Pts',(-0.21458747046378,-0.166830061761007,
-1.37108963898761));
#51826=CARTESIAN_POINT('Ctrl Pts',(0.0241613530569681,-0.270733207897134,
-1.35837036616662));
#51827=CARTESIAN_POINT('Ctrl Pts',(0.240738733928709,-0.126194691406434,
-1.34565109334564));
#51828=CARTESIAN_POINT('Ctrl Pts',(0.236399199351971,0.134147703006429,
-1.33293182052465));
#51829=CARTESIAN_POINT('Ctrl Pts',(0.0151253724564228,0.2713879882983,-1.32021254770366));
#51830=CARTESIAN_POINT('Ctrl Pts',(-0.220028497678877,0.1595859470328,-1.30749327488268));
#51831=CARTESIAN_POINT('Ctrl Pts',(-0.253270661793043,-0.0986619463133894,
-1.29477400206169));
#51832=CARTESIAN_POINT('Ctrl Pts',(-0.0540961254135104,-0.266371585304427,
-1.28205472924071));
#51833=CARTESIAN_POINT('Ctrl Pts',(0.194720349771229,-0.189642286639183,
-1.26933545641972));
#51834=CARTESIAN_POINT('Ctrl Pts',(0.264849462798021,0.0611144233860401,
-1.25661618359873));
#51835=CARTESIAN_POINT('Ctrl Pts',(0.0919364391210603,0.255788784967876,
-1.24389691077775));
#51836=CARTESIAN_POINT('Ctrl Pts',(-0.165343111230579,0.215735640930078,
-1.23117763795676));
#51837=CARTESIAN_POINT('Ctrl Pts',(-0.270893663145469,-0.0222897817783964,
-1.21845836513578));
#51838=CARTESIAN_POINT('Ctrl Pts',(-0.127855546302129,-0.23986073142624,
-1.20573909231479));
#51839=CARTESIAN_POINT('Ctrl Pts',(0.132510675567995,-0.237320736625336,
-1.1930198194938));
#51840=CARTESIAN_POINT('Ctrl Pts',(0.271276959886478,-0.0170006528213758,
-1.18030054667282));
#51841=CARTESIAN_POINT('Ctrl Pts',(0.161102838452268,0.218920274570346,
-1.16758127385183));
#51842=CARTESIAN_POINT('Ctrl Pts',(-0.0969091458332232,0.253946507407051,
-1.15486200103085));
#51843=CARTESIAN_POINT('Ctrl Pts',(-0.265991343728995,0.0559358224275761,
-1.14214272820986));
#51844=CARTESIAN_POINT('Ctrl Pts',(-0.190983541958354,-0.193405009946382,
-1.12942345538888));
#51845=CARTESIAN_POINT('Ctrl Pts',(0.0592824920623715,-0.265265522270368,
-1.11670418256789));
#51846=CARTESIAN_POINT('Ctrl Pts',(0.255147269012042,-0.093702093285758,
-1.1039849097469));
#51847=CARTESIAN_POINT('Ctrl Pts',(0.216873235514688,0.163848133611853,
-1.09126563692592));
#51848=CARTESIAN_POINT('Ctrl Pts',(-0.0204170037146158,0.271041246178294,
-1.07854636410493));
#51849=CARTESIAN_POINT('Ctrl Pts',(-0.238971345901963,0.129510258313282,
-1.06582709128394));
#51850=CARTESIAN_POINT('Ctrl Pts',(-0.238230898545541,-0.130867299768838,
-1.05310781846296));
#51851=CARTESIAN_POINT('Ctrl Pts',(-0.0188751416328633,-0.271152983016823,
-1.04038854564197));
#51852=CARTESIAN_POINT('Ctrl Pts',(0.21780160494222,-0.162612029245002,
-1.02766927282099));
#51853=CARTESIAN_POINT('Ctrl Pts',(0.254610216959755,0.0951517135436653,
-1.01495));
#51854=CARTESIAN_POINT('Ctrl Pts',(0.0577728504889806,0.265598397805716,
-1.00223072717901));
#51855=CARTESIAN_POINT('Ctrl Pts',(-0.192080433189419,0.192315673714733,
-0.989511454358027));
#51856=CARTESIAN_POINT('Ctrl Pts',(-0.265668909834996,-0.0574477285684278,
-0.976792181537043));
#51857=CARTESIAN_POINT('Ctrl Pts',(-0.0954632719571637,-0.254493565493941,
-0.964072908716056));
#51858=CARTESIAN_POINT('Ctrl Pts',(0.162345329589841,-0.218000470483329,
-0.95135363589507));
#51859=CARTESIAN_POINT('Ctrl Pts',(0.271175882109777,0.0185432503238013,
-0.938634363074085));
#51860=CARTESIAN_POINT('Ctrl Pts',(0.131158783995253,0.238070545325274,
-0.925915090253097));
#51861=CARTESIAN_POINT('Ctrl Pts',(-0.129217672788485,0.2391296807377,-0.913195817432114));
#51862=CARTESIAN_POINT('Ctrl Pts',(-0.271016053809387,0.0207487288327176,
-0.900476544611126));
#51863=CARTESIAN_POINT('Ctrl Pts',(-0.164113452464216,-0.21667253146364,
-0.887757271790141));
#51864=CARTESIAN_POINT('Ctrl Pts',(0.0933897360920922,-0.255261764397326,
-0.875037998969154));
#51865=CARTESIAN_POINT('Ctrl Pts',(0.265192764888317,-0.0596071188825326,
-0.862318726148169));
#51866=CARTESIAN_POINT('Ctrl Pts',(0.193638619018841,0.190746681216378,
-0.849599453327181));
#51867=CARTESIAN_POINT('Ctrl Pts',(-0.0556102209364207,0.266059607039455,
-0.836880180506197));
#51868=CARTESIAN_POINT('Ctrl Pts',(-0.253827705434749,0.097219890579639,
-0.82416090768521));
#51869=CARTESIAN_POINT('Ctrl Pts',(-0.21911729209811,-0.160834770725045,
-0.811441634864225));
#51870=CARTESIAN_POINT('Ctrl Pts',(0.0166686111669654,-0.27129756462665,
-0.798722362043238));
#51871=CARTESIAN_POINT('Ctrl Pts',(0.237158372695661,-0.132801044540064,
-0.786003089222253));
#51872=CARTESIAN_POINT('Ctrl Pts',(0.240017040284684,0.127561873393136,
-0.773283816401267));
#51873=CARTESIAN_POINT('Ctrl Pts',(0.0226213249160781,0.270866178821993,
-0.76056454358028));
#51874=CARTESIAN_POINT('Ctrl Pts',(-0.215533108063434,0.165607036381619,
-0.747845270759295));
#51875=CARTESIAN_POINT('Ctrl Pts',(-0.255901118599167,-0.0916232976392016,
-0.735125997938309));
#51876=CARTESIAN_POINT('Ctrl Pts',(-0.0614385399885019,-0.26477446435536,
-0.722406725117323));
#51877=CARTESIAN_POINT('Ctrl Pts',(0.189403817736741,-0.194952314675497,
-0.709687452296337));
#51878=CARTESIAN_POINT('Ctrl Pts',(0.26643759522141,0.0537700569389561,
-0.69696817947535));
#51879=CARTESIAN_POINT('Ctrl Pts',(0.0989718652436024,0.253149720641341,
-0.684248906654365));
#51880=CARTESIAN_POINT('Ctrl Pts',(-0.159316529173112,0.220223647010986,
-0.671529633833378));
#51881=CARTESIAN_POINT('Ctrl Pts',(-0.271406287916481,-0.0147931757909765,
-0.658810361012393));
#51882=CARTESIAN_POINT('Ctrl Pts',(-0.134436961500886,-0.236234871585454,
-0.646091088191406));
#51883=CARTESIAN_POINT('Ctrl Pts',(0.125899980676306,-0.240892934799451,
-0.633371815370422));
#51884=CARTESIAN_POINT('Ctrl Pts',(0.270703365213811,-0.0244928404335767,
-0.620652542549433));
#51885=CARTESIAN_POINT('Ctrl Pts',(0.167092709652319,0.214383389169106,
-0.60793326972845));
#51886=CARTESIAN_POINT('Ctrl Pts',(-0.0898524825634798,0.256528249024871,
-0.595213996907462));
#51887=CARTESIAN_POINT('Ctrl Pts',(-0.26434351618805,0.0632670263243382,
-0.582494724086477));
#51888=CARTESIAN_POINT('Ctrl Pts',(-0.196256697932639,-0.188051906895844,
-0.569775451265491));
#51889=CARTESIAN_POINT('Ctrl Pts',(0.051927324476213,-0.266802856325281,
-0.557056178444504));
#51890=CARTESIAN_POINT('Ctrl Pts',(0.25245964349941,-0.100719112261466,
-0.544336905623519));
#51891=CARTESIAN_POINT('Ctrl Pts',(0.22131948237406,0.157790677456764,-0.531617632802532));
#51892=CARTESIAN_POINT('Ctrl Pts',(-0.0129170337808407,0.271502046785822,
-0.518898359981547));
#51893=CARTESIAN_POINT('Ctrl Pts',(-0.235300086108064,0.136066456733929,
-0.506179087160561));
#51894=CARTESIAN_POINT('Ctrl Pts',(-0.241757322442635,-0.124232074022583,
-0.493459814339575));
#51895=CARTESIAN_POINT('Ctrl Pts',(-0.0263631859874709,-0.270527620762044,
-0.480740541518589));
#51896=CARTESIAN_POINT('Ctrl Pts',(0.213223429699964,-0.168570401309326,
-0.468021268697603));
#51897=CARTESIAN_POINT('Ctrl Pts',(0.257143125717892,0.0880773754524993,
-0.455301995876617));
#51898=CARTESIAN_POINT('Ctrl Pts',(0.0650924905477743,0.263899940971675,
-0.442582723055631));
#51899=CARTESIAN_POINT('Ctrl Pts',(-0.186691013271359,0.197551706483163,
-0.429863450234646));
#51900=CARTESIAN_POINT('Ctrl Pts',(-0.267155372903108,-0.050082111571277,
-0.417144177413658));
#51901=CARTESIAN_POINT('Ctrl Pts',(-0.102461548172094,-0.251757506971836,
-0.404424904592674));
#51902=CARTESIAN_POINT('Ctrl Pts',(0.156257288463409,-0.222404745842757,
-0.391705631771687));
#51903=CARTESIAN_POINT('Ctrl Pts',(0.271584836658268,0.0110402747568785,
-0.378986358950701));
#51904=CARTESIAN_POINT('Ctrl Pts',(0.137689452406416,0.234354060912939,
-0.366267086129715));
#51905=CARTESIAN_POINT('Ctrl Pts',(-0.122558233111938,0.242610161930231,
-0.353547813308729));
#51906=CARTESIAN_POINT('Ctrl Pts',(-0.27033895384612,0.0282322722250301,
-0.340828540487743));
#51907=CARTESIAN_POINT('Ctrl Pts',(-0.170040040796351,-0.212053285043769,
-0.328109267666758));
#51908=CARTESIAN_POINT('Ctrl Pts',(0.0862980611549639,-0.257745719346492,
-0.315389994845771));
#51909=CARTESIAN_POINT('Ctrl Pts',(0.263443759787759,-0.0669148453856698,
-0.302670722024786));
#51910=CARTESIAN_POINT('Ctrl Pts',(0.198837278671528,0.185321201726677,
-0.289951449203799));
#51911=CARTESIAN_POINT('Ctrl Pts',(-0.0482345067540092,0.267495128388911,
-0.277232176382814));
#51912=CARTESIAN_POINT('Ctrl Pts',(-0.25104334385758,0.10419908922353,-0.264512903561827));
#51913=CARTESIAN_POINT('Ctrl Pts',(-0.223479386987627,-0.154716434448323,
-0.251793630740842));
#51914=CARTESIAN_POINT('Ctrl Pts',(0.00916299105612257,-0.27165465546766,
-0.239074357919855));
#51915=CARTESIAN_POINT('Ctrl Pts',(0.233396836065409,-0.139305867392902,
-0.22635508509887));
#51916=CARTESIAN_POINT('Ctrl Pts',(0.243451422288832,0.120878531041389,
-0.213635812277883));
#51917=CARTESIAN_POINT('Ctrl Pts',(0.0300999912562831,0.270137386547874,
-0.200916539456898));
#51918=CARTESIAN_POINT('Ctrl Pts',(-0.210872975634221,0.171501533005751,
-0.188197266635911));
#51919=CARTESIAN_POINT('Ctrl Pts',(-0.258336068703837,-0.084514577200677,
-0.175477993814926));
#51920=CARTESIAN_POINT('Ctrl Pts',(-0.068733875007705,-0.262975084877335,
-0.16275872099394));
#51921=CARTESIAN_POINT('Ctrl Pts',(0.183942292280123,-0.200113180720208,
-0.150039448172954));
#51922=CARTESIAN_POINT('Ctrl Pts',(0.267822574232866,0.0463842698012505,
-0.137320175351968));
#51923=CARTESIAN_POINT('Ctrl Pts',(0.105930761173157,0.250317814243884,
-0.124600902530982));
#51924=CARTESIAN_POINT('Ctrl Pts',(-0.153166490592751,0.224542161574117,
-0.111881629709996));
#51925=CARTESIAN_POINT('Ctrl Pts',(-0.271714736521166,-0.00728299906578173,
-0.0991623568890098));
#51926=CARTESIAN_POINT('Ctrl Pts',(-0.140909456453654,-0.232432789475941,
-0.0864430840680238));
#51927=CARTESIAN_POINT('Ctrl Pts',(0.119181293416937,-0.244272807209766,
-0.0737238112470379));
#51928=CARTESIAN_POINT('Ctrl Pts',(0.26994533231077,-0.0319819907460251,
-0.0610045384260516));
#51929=CARTESIAN_POINT('Ctrl Pts',(0.172912084788245,0.209712576849484,
-0.0482852656050659));
#51930=CARTESIAN_POINT('Ctrl Pts',(-0.0826453397628101,0.258856681156889,
-0.0355659927840798));
#51931=CARTESIAN_POINT('Ctrl Pts',(-0.262651769244295,0.0706612461396808,
-0.0228467199630939));
#51932=CARTESIAN_POINT('Ctrl Pts',(-0.201059487573804,-0.182786714230045,
-0.0101274471421079));
#51933=CARTESIAN_POINT('Ctrl Pts',(-0.0378468489242762,-0.23929252810158,
-0.00164793192811731));
#51934=CARTESIAN_POINT('Ctrl Pts',(0.0376593651558268,-0.226752344241108,
0.00259182567887802));
#51935=CARTESIAN_POINT('Ctrl Pts',(-0.0796899944392894,-0.231730462577249,
-1.51495));
#51936=CARTESIAN_POINT('Ctrl Pts',(-0.00252611781081108,-0.258266416594894,
-1.510710242393));
#51937=CARTESIAN_POINT('Ctrl Pts',(0.179055320931291,-0.227722318580645,
-1.50223072717901));
#51938=CARTESIAN_POINT('Ctrl Pts',(0.288627271809818,0.0278416748802775,
-1.48951145435803));
#51939=CARTESIAN_POINT('Ctrl Pts',(0.132661969671875,0.25752738104281,-1.47679218153704));
#51940=CARTESIAN_POINT('Ctrl Pts',(-0.144701862128332,0.251052642665116,
-1.46407290871606));
#51941=CARTESIAN_POINT('Ctrl Pts',(-0.289455302408456,0.0141124785371433,
-1.45135363589507));
#51942=CARTESIAN_POINT('Ctrl Pts',(-0.168494115819424,-0.235734168981793,
-1.43863436307408));
#51943=CARTESIAN_POINT('Ctrl Pts',(0.107039023450112,-0.269279729649273,
-1.4259150902531));
#51944=CARTESIAN_POINT('Ctrl Pts',(0.284372078802149,-0.0557055613755665,
-1.41319581743211));
#51945=CARTESIAN_POINT('Ctrl Pts',(0.200734461553377,0.208981101084686,
-1.40047654461112));
#51946=CARTESIAN_POINT('Ctrl Pts',(-0.0671024091797608,0.281897198190798,
-1.38775727179014));
#51947=CARTESIAN_POINT('Ctrl Pts',(-0.2733656710537,0.0961253573556439,
-1.37503799896915));
#51948=CARTESIAN_POINT('Ctrl Pts',(-0.22876986391828,-0.177856099631807,
-1.36231872614817));
#51949=CARTESIAN_POINT('Ctrl Pts',(0.0257582115068392,-0.288626353602694,
-1.34959945332718));
#51950=CARTESIAN_POINT('Ctrl Pts',(0.256649501863742,-0.134535079414771,
-1.3368801805062));
#51951=CARTESIAN_POINT('Ctrl Pts',(0.252023161227715,0.143013716949099,
-1.32416090768521));
#51952=CARTESIAN_POINT('Ctrl Pts',(0.0161250299986812,0.289324409378958,
-1.31144163486423));
#51953=CARTESIAN_POINT('Ctrl Pts',(-0.234570496419716,0.170133210979464,
-1.29872236204324));
#51954=CARTESIAN_POINT('Ctrl Pts',(-0.270009682800502,-0.105182655740546,
-1.28600308922225));
#51955=CARTESIAN_POINT('Ctrl Pts',(-0.0576714158688228,-0.283976465122066,
-1.27328381640127));
#51956=CARTESIAN_POINT('Ctrl Pts',(0.207589696747008,-0.202176017145047,
-1.26056454358028));
#51957=CARTESIAN_POINT('Ctrl Pts',(0.282353743357815,0.0651535632124803,
-1.2478452707593));
#51958=CARTESIAN_POINT('Ctrl Pts',(0.0980126501393592,0.272694232344753,
-1.23512599793831));
#51959=CARTESIAN_POINT('Ctrl Pts',(-0.176270874409831,0.229993918616173,
-1.22240672511732));
#51960=CARTESIAN_POINT('Ctrl Pts',(-0.288797413568345,-0.0237629454002635,
-1.20968745229634));
#51961=CARTESIAN_POINT('Ctrl Pts',(-0.136305702590742,-0.255713470917593,
-1.19696817947535));
#51962=CARTESIAN_POINT('Ctrl Pts',(0.141268496021188,-0.253005604220159,
-1.18424890665437));
#51963=CARTESIAN_POINT('Ctrl Pts',(0.289206042940281,-0.0181242503304727,
-1.17152963383338));
#51964=CARTESIAN_POINT('Ctrl Pts',(0.171750355926746,0.233389029257715,
-1.15881036101239));
#51965=CARTESIAN_POINT('Ctrl Pts',(-0.103314010164656,0.270730196019714,
-1.14609108819141));
#51966=CARTESIAN_POINT('Ctrl Pts',(-0.283571092835979,0.0596327010950711,
-1.13337181537042));
#51967=CARTESIAN_POINT('Ctrl Pts',(-0.203605917950455,-0.206187424228085,
-1.12065254254943));
#51968=CARTESIAN_POINT('Ctrl Pts',(0.0632005569222366,-0.282797300796956,
-1.10793326972845));
#51969=CARTESIAN_POINT('Ctrl Pts',(0.272010317680024,-0.0998949989182119,
-1.09521399690746));
#51970=CARTESIAN_POINT('Ctrl Pts',(0.2312066984572,0.174677091577786,-1.08249472408648));
#51971=CARTESIAN_POINT('Ctrl Pts',(-0.0217663927503151,0.288954750575316,
-1.06977545126549));
#51972=CARTESIAN_POINT('Ctrl Pts',(-0.254765304629413,0.138069776890128,
-1.0570561784445));
#51973=CARTESIAN_POINT('Ctrl Pts',(-0.25397592004605,-0.139516507160294,
-1.04433690562352));
#51974=CARTESIAN_POINT('Ctrl Pts',(-0.0201226267938958,-0.289073872261636,
-1.03161763280253));
#51975=CARTESIAN_POINT('Ctrl Pts',(0.232196425150669,-0.173359291301837,
-1.01889835998155));
#51976=CARTESIAN_POINT('Ctrl Pts',(0.271437771087937,0.101440426656454,
-1.00617908716056));
#51977=CARTESIAN_POINT('Ctrl Pts',(0.0615911409737527,0.283152176553489,
-0.993459814339575));
#51978=CARTESIAN_POINT('Ctrl Pts',(-0.204775304294965,0.205026092203729,
-0.980740541518589));
#51979=CARTESIAN_POINT('Ctrl Pts',(-0.283227348823837,-0.0612445312795246,
-0.968021268697604));
#51980=CARTESIAN_POINT('Ctrl Pts',(-0.101772576412007,-0.27131340995957,
-0.955301995876616));
#51981=CARTESIAN_POINT('Ctrl Pts',(0.173074965084248,-0.232408434000391,
-0.942582723055633));
#51982=CARTESIAN_POINT('Ctrl Pts',(0.28909828478846,0.0197688003125712,
-0.929863450234644));
#51983=CARTESIAN_POINT('Ctrl Pts',(0.139827255996971,0.253804968851647,
-0.91714417741366));
#51984=CARTESIAN_POINT('Ctrl Pts',(-0.137757853968682,0.25493410404136,
-0.904424904592673));
#51985=CARTESIAN_POINT('Ctrl Pts',(-0.288927893206643,0.0221200420568807,
-0.891705631771688));
#51986=CARTESIAN_POINT('Ctrl Pts',(-0.174959945733342,-0.230992729587781,
-0.8789863589507));
#51987=CARTESIAN_POINT('Ctrl Pts',(0.0995619975899653,-0.272132380229409,
-0.866267086129716));
#51988=CARTESIAN_POINT('Ctrl Pts',(0.282719734775254,-0.0635466387941777,
-0.853547813308729));
#51989=CARTESIAN_POINT('Ctrl Pts',(0.206436472858937,0.203353402742587,
-0.840828540487744));
#51990=CARTESIAN_POINT('Ctrl Pts',(-0.0592855801347328,0.283643867766458,
-0.828109267666757));
#51991=CARTESIAN_POINT('Ctrl Pts',(-0.270603542254802,0.103645292476704,
-0.815389994845772));
#51992=CARTESIAN_POINT('Ctrl Pts',(-0.233599067956243,-0.171464571219253,
-0.802670722024785));
#51993=CARTESIAN_POINT('Ctrl Pts',(0.0177702635672599,-0.28922800947726,
-0.7899514492038));
#51994=CARTESIAN_POINT('Ctrl Pts',(0.252832509425682,-0.14157805589476,
-0.777232176382813));
#51995=CARTESIAN_POINT('Ctrl Pts',(0.255880110452505,0.135992620418319,
-0.764512903561829));
#51996=CARTESIAN_POINT('Ctrl Pts',(0.0241164006990628,0.288768112766542,
-0.75179363074084));
#51997=CARTESIAN_POINT('Ctrl Pts',(-0.229778000062115,0.176552242752344,
-0.739074357919857));
#51998=CARTESIAN_POINT('Ctrl Pts',(-0.272813990266727,-0.0976788126881887,
-0.726355085098868));
#51999=CARTESIAN_POINT('Ctrl Pts',(-0.0654991011457034,-0.282273788160596,
-0.713635812277885));
#52000=CARTESIAN_POINT('Ctrl Pts',(0.201921787491083,-0.207836992544237,
-0.700916539456897));
#52001=CARTESIAN_POINT('Ctrl Pts',(0.284046837729065,0.0573237970614832,
-0.688197266635913));
#52002=CARTESIAN_POINT('Ctrl Pts',(0.105513057657014,0.269880748474758,
-0.675477993814925));
#52003=CARTESIAN_POINT('Ctrl Pts',(-0.169845986907316,0.23477854345086,
-0.662758720993941));
#52004=CARTESIAN_POINT('Ctrl Pts',(-0.289343918445131,-0.0157708779795308,
-0.650039448172953));
#52005=CARTESIAN_POINT('Ctrl Pts',(-0.143322092952003,-0.251847972803605,
-0.637320175351968));
#52006=CARTESIAN_POINT('Ctrl Pts',(0.134220890830127,-0.256813894091022,
-0.624600902530981));
#52007=CARTESIAN_POINT('Ctrl Pts',(0.288594538573662,-0.0261116073592364,
-0.611881629709995));
#52008=CARTESIAN_POINT('Ctrl Pts',(0.178136106298667,0.228552294598365,
-0.599162356889011));
#52009=CARTESIAN_POINT('Ctrl Pts',(-0.0957909619063059,0.273482568641024,
-0.586443084068023));
#52010=CARTESIAN_POINT('Ctrl Pts',(-0.281814358011304,0.0674484347639324,
-0.573723811247039));
#52011=CARTESIAN_POINT('Ctrl Pts',(-0.209227584360194,-0.20048052692525,
-0.561004538426051));
#52012=CARTESIAN_POINT('Ctrl Pts',(0.055359275769404,-0.284436239462757,
-0.548285265605067));
#52013=CARTESIAN_POINT('Ctrl Pts',(0.269145063145547,-0.107375782734319,
-0.535565992784079));
#52014=CARTESIAN_POINT('Ctrl Pts',(0.235946804143553,0.168219289464292,
-0.522846719963094));
#52015=CARTESIAN_POINT('Ctrl Pts',(-0.0137707390551913,0.289446006155381,
-0.510127447142108));
#52016=CARTESIAN_POINT('Ctrl Pts',(-0.250851406014347,0.145059283860275,
-0.497408174321121));
#52017=CARTESIAN_POINT('Ctrl Pts',(-0.257735410352323,-0.132442749835334,
-0.484688901500136));
#52018=CARTESIAN_POINT('Ctrl Pts',(-0.028105566731234,-0.288407178919214,
-0.471969628679149));
#52019=CARTESIAN_POINT('Ctrl Pts',(0.227315671745536,-0.179711460715009,
-0.459250355858164));
#52020=CARTESIAN_POINT('Ctrl Pts',(0.274138083415885,0.0938985354224031,
-0.446531083037178));
#52021=CARTESIAN_POINT('Ctrl Pts',(0.069394546534021,0.281341466273177,
-0.433811810216192));
#52022=CARTESIAN_POINT('Ctrl Pts',(-0.199029689890786,0.210608181881736,
-0.421092537395206));
#52023=CARTESIAN_POINT('Ctrl Pts',(-0.284812054366414,-0.0533921100991525,
-0.40837326457422));
#52024=CARTESIAN_POINT('Ctrl Pts',(-0.109233378731415,-0.268396521408613,
-0.395653991753234));
#52025=CARTESIAN_POINT('Ctrl Pts',(0.166584556594821,-0.237103794230219,
-0.382934718932248));
#52026=CARTESIAN_POINT('Ctrl Pts',(0.289534267729147,0.0117699423376978,
-0.370215446111262));
#52027=CARTESIAN_POINT('Ctrl Pts',(0.146789545642719,0.249842856658299,
-0.357496173290276));
#52028=CARTESIAN_POINT('Ctrl Pts',(-0.130658282380074,0.258644615223885,
-0.34477690046929));
#52029=CARTESIAN_POINT('Ctrl Pts',(-0.288206042736432,0.030098183556875,
-0.332057627648304));
#52030=CARTESIAN_POINT('Ctrl Pts',(-0.181278230781915,-0.226068190552044,
-0.319338354827318));
#52031=CARTESIAN_POINT('Ctrl Pts',(0.0920016236929569,-0.274780503320994,
-0.306619082006332));
#52032=CARTESIAN_POINT('Ctrl Pts',(0.28085513542105,-0.0713373434148228,
-0.293899809185346));
#52033=CARTESIAN_POINT('Ctrl Pts',(0.211978719378421,0.197569345537999,
-0.281180536364361));
#52034=CARTESIAN_POINT('Ctrl Pts',(-0.0514223944316555,0.285174264779187,
-0.268461263543374));
#52035=CARTESIAN_POINT('Ctrl Pts',(-0.267635158230649,0.111085756361062,
-0.255741990722389));
#52036=CARTESIAN_POINT('Ctrl Pts',(-0.238249459948454,-0.164941865329635,
-0.243022717901402));
#52037=CARTESIAN_POINT('Ctrl Pts',(0.00976858626676915,-0.28960870096371,
-0.230303445080417));
#52038=CARTESIAN_POINT('Ctrl Pts',(0.248822367448769,-0.148512791812193,
-0.217584172259431));
#52039=CARTESIAN_POINT('Ctrl Pts',(0.25954147568522,0.128867566392453,-0.204864899438444));
#52040=CARTESIAN_POINT('Ctrl Pts',(0.032089342815586,0.287991153566572,
-0.192145626617459));
#52041=CARTESIAN_POINT('Ctrl Pts',(-0.224809872802084,0.182836315105941,
-0.179426353796473));
#52042=CARTESIAN_POINT('Ctrl Pts',(-0.275409869713412,-0.0901002667281681,
-0.166707080975487));
#52043=CARTESIAN_POINT('Ctrl Pts',(-0.0732765953114828,-0.280355485114124,
-0.153987808154501));
#52044=CARTESIAN_POINT('Ctrl Pts',(0.196099301989967,-0.213338947622031,
-0.141268535333515));
#52045=CARTESIAN_POINT('Ctrl Pts',(0.285523351988242,0.0494498726670601,
-0.128549262512529));
#52046=CARTESIAN_POINT('Ctrl Pts',(0.112931876991549,0.266861677325006,
-0.115829989691543));
#52047=CARTESIAN_POINT('Ctrl Pts',(-0.16328948346338,0.239382474830457,
-0.103110716870557));
#52048=CARTESIAN_POINT('Ctrl Pts',(-0.289672752860146,-0.00776434291151507,
-0.0903914440495708));
#52049=CARTESIAN_POINT('Ctrl Pts',(-0.15022236437212,-0.2477946056386,-0.0776721712285848));
#52050=CARTESIAN_POINT('Ctrl Pts',(0.127058155901041,-0.260417147112729,
-0.0649528984075989));
#52051=CARTESIAN_POINT('Ctrl Pts',(0.2877864061897,-0.0340957263487534,
-0.0522336255866126));
#52052=CARTESIAN_POINT('Ctrl Pts',(0.184340092277242,0.223572781598662,
-0.0395143527656268));
#52053=CARTESIAN_POINT('Ctrl Pts',(-0.0881074887091739,0.275964890189591,
-0.0267950799446408));
#52054=CARTESIAN_POINT('Ctrl Pts',(-0.280010801087544,0.0753313491637424,
-0.0140758071236549));
#52055=CARTESIAN_POINT('Ctrl Pts',(-0.214347797251761,-0.194867350130467,
-0.00135653430266889));
#52056=CARTESIAN_POINT('Ctrl Pts',(-0.0403482014091038,-0.255107714220899,
0.00712298091132171));
#52057=CARTESIAN_POINT('Ctrl Pts',(0.0401483265697059,-0.241738731637386,
0.011362738518317));
#52058=CARTESIAN_POINT('Ctrl Pts',(-0.24544712988196,-4.00287140078511E-5,
-0.0907327496212059));
#52059=CARTESIAN_POINT('Ctrl Pts',(-0.245452120854431,-0.00221980312011781,
-0.0906189810973275));
#52060=CARTESIAN_POINT('Ctrl Pts',(-0.245425583143613,-0.00439945378707234,
-0.0905052125734492));
#52061=CARTESIAN_POINT('Ctrl Pts',(-0.24536714321268,-0.0065782504090337,
-0.0903914440495708));
#52062=CARTESIAN_POINT('Ctrl Pts',(-0.243189290030804,-0.0877744304872093,
-0.0861516864425755));
#52063=CARTESIAN_POINT('Ctrl Pts',(-0.196705827201461,-0.167784518062905,
-0.0819119288355801));
#52064=CARTESIAN_POINT('Ctrl Pts',(-0.127250675741264,-0.209893318763107,
-0.0776721712285849));
#52065=CARTESIAN_POINT('Ctrl Pts',(-0.0577955242810662,-0.25200211946331,
-0.0734324136215895));
#52066=CARTESIAN_POINT('Ctrl Pts',(0.0346313158099865,-0.256209633288019,
-0.0691926560145943));
#52067=CARTESIAN_POINT('Ctrl Pts',(0.10763277757029,-0.220593153406378,
-0.0649528984075989));
#52068=CARTESIAN_POINT('Ctrl Pts',(0.180634239330593,-0.184976673524737,
-0.0607131408006035));
#52069=CARTESIAN_POINT('Ctrl Pts',(0.234210322760147,-0.109536199936745,
-0.056473383193608));
#52070=CARTESIAN_POINT('Ctrl Pts',(0.24375731215618,-0.0288712118181801,
-0.0522336255866127));
#52071=CARTESIAN_POINT('Ctrl Pts',(0.253304301552214,0.0517937763003857,
-0.0479938679796173));
#52072=CARTESIAN_POINT('Ctrl Pts',(0.218822196914728,0.137683278949523,
-0.0437541103726222));
#52073=CARTESIAN_POINT('Ctrl Pts',(0.156173214431582,0.189360048372581,
-0.0395143527656269));
#52074=CARTESIAN_POINT('Ctrl Pts',(0.093524231948437,0.241036817795638,
-0.0352745951586316));
#52075=CARTESIAN_POINT('Ctrl Pts',(0.00270837161963094,0.258500853992614,
-0.0310348375516362));
#52076=CARTESIAN_POINT('Ctrl Pts',(-0.0746834439411661,0.233793948586794,
-0.0267950799446409));
#52077=CARTESIAN_POINT('Ctrl Pts',(-0.146756136718545,0.210785143458111,
-0.0228467199630937));
#52078=CARTESIAN_POINT('Ctrl Pts',(-0.20718663585062,0.151202989772472,
-0.0188983599815467));
#52079=CARTESIAN_POINT('Ctrl Pts',(-0.232146082211076,0.0797430227058862,
-0.0149499999999996));
#52080=CARTESIAN_POINT('',(0.197117931249732,0.0326679887445553,-1.51495));
#52081=CARTESIAN_POINT('Ctrl Pts',(0.197120364464142,0.0326678919976635,
-1.51495));
#52082=CARTESIAN_POINT('Ctrl Pts',(0.19839158954313,0.0282478473569942,
-1.51495));
#52083=CARTESIAN_POINT('Ctrl Pts',(0.19949723577291,0.0237887889107814,
-1.51495));
#52084=CARTESIAN_POINT('Ctrl Pts',(0.200432284720987,0.0192980969514664,
-1.51495));
#52085=CARTESIAN_POINT('Ctrl Pts',(0.202577213948768,0.00899680047248181,
-1.51495));
#52086=CARTESIAN_POINT('Ctrl Pts',(0.203826058329088,-0.00147033997848461,
-1.51495));
#52087=CARTESIAN_POINT('Ctrl Pts',(0.20423417638802,-0.01200912787121,-1.51495));
#52088=CARTESIAN_POINT('Ctrl Pts',(0.204460722409734,-0.0178592009530887,
-1.51495));
#52089=CARTESIAN_POINT('Ctrl Pts',(0.204427206594989,-0.0237345590497023,
-1.51495));
#52090=CARTESIAN_POINT('Ctrl Pts',(0.204142815235946,-0.0295947455656042,
-1.51495));
#52091=CARTESIAN_POINT('Ctrl Pts',(0.203701770180365,-0.038682948161926,
-1.51495));
#52092=CARTESIAN_POINT('Ctrl Pts',(0.202658993444603,-0.047746378507929,
-1.51495));
#52093=CARTESIAN_POINT('Ctrl Pts',(0.201046184074424,-0.0567275139665697,
-1.51495));
#52094=CARTESIAN_POINT('Ctrl Pts',(0.200183877514263,-0.0615293784440873,
-1.51495));
#52095=CARTESIAN_POINT('Ctrl Pts',(0.199158432739084,-0.0663077749781463,
-1.51495));
#52096=CARTESIAN_POINT('Ctrl Pts',(0.197973440998626,-0.0710540933796172,
-1.51495));
#52097=CARTESIAN_POINT('Ctrl Pts',(0.196939744036605,-0.0751944217421482,
-1.51495));
#52098=CARTESIAN_POINT('Ctrl Pts',(0.195785043563296,-0.0793077977796779,
-1.51495));
#52099=CARTESIAN_POINT('Ctrl Pts',(0.194515550626655,-0.0833781506086003,
-1.51495));
#52100=CARTESIAN_POINT('Ctrl Pts',(0.19033267790619,-0.0967896216923322,
-1.51495));
#52101=CARTESIAN_POINT('Ctrl Pts',(0.184899873663921,-0.109766099393497,
-1.51495));
#52102=CARTESIAN_POINT('Ctrl Pts',(0.178313994607811,-0.122111154788251,
-1.51495));
#52103=CARTESIAN_POINT('Ctrl Pts',(0.173663514747407,-0.130828355787502,
-1.51495));
#52104=CARTESIAN_POINT('Ctrl Pts',(0.168436916876066,-0.139231082048986,
-1.51495));
#52105=CARTESIAN_POINT('Ctrl Pts',(0.162653150682954,-0.147246871784982,
-1.51495));
#52106=CARTESIAN_POINT('Ctrl Pts',(0.160516541128603,-0.150208024148989,
-1.51495));
#52107=CARTESIAN_POINT('Ctrl Pts',(0.158305528707968,-0.153113639786799,
-1.51495));
#52108=CARTESIAN_POINT('Ctrl Pts',(0.156026676769085,-0.155953801417746,
-1.51495));
#52109=CARTESIAN_POINT('Ctrl Pts',(0.150504934476818,-0.162835617795061,
-1.51495));
#52110=CARTESIAN_POINT('Ctrl Pts',(0.144577160304343,-0.169344859396806,
-1.51495));
#52111=CARTESIAN_POINT('Ctrl Pts',(0.138263901802813,-0.175434489995263,
-1.51495));
#52112=CARTESIAN_POINT('Ctrl Pts',(0.131281509670573,-0.182169552208951,
-1.51495));
#52113=CARTESIAN_POINT('Ctrl Pts',(0.123827735071421,-0.188391742560213,
-1.51495));
#52114=CARTESIAN_POINT('Ctrl Pts',(0.115968478775398,-0.194097892548868,
-1.51495));
#52115=CARTESIAN_POINT('Ctrl Pts',(0.11169834481699,-0.197198189055378,
-1.51495));
#52116=CARTESIAN_POINT('Ctrl Pts',(0.107308328841664,-0.200146016980857,
-1.51495));
#52117=CARTESIAN_POINT('Ctrl Pts',(0.102807906095061,-0.202939831405905,
-1.51495));
#52118=CARTESIAN_POINT('Ctrl Pts',(0.0986064882257294,-0.205548026793295,
-1.51495));
#52119=CARTESIAN_POINT('Ctrl Pts',(0.0943066784205236,-0.208022722670441,
-1.51495));
#52120=CARTESIAN_POINT('Ctrl Pts',(0.0899371264991721,-0.210351864187837,
-1.51495));
#52121=CARTESIAN_POINT('Ctrl Pts',(0.0771241238284205,-0.217181694115504,
-1.51495));
#52122=CARTESIAN_POINT('Ctrl Pts',(0.0636786011257452,-0.222786608559561,
-1.51495));
#52123=CARTESIAN_POINT('Ctrl Pts',(0.0498091216440218,-0.227155802214754,
-1.51495));
#52124=CARTESIAN_POINT('Ctrl Pts',(0.0425067356028674,-0.229456215781162,
-1.51495));
#52125=CARTESIAN_POINT('Ctrl Pts',(0.0350861499587181,-0.23141347164588,
-1.51495));
#52126=CARTESIAN_POINT('Ctrl Pts',(0.0275745313202283,-0.233021485604181,
-1.51495));
#52127=CARTESIAN_POINT('Ctrl Pts',(0.0230174188518951,-0.233997027735816,
-1.51495));
#52128=CARTESIAN_POINT('Ctrl Pts',(0.0184267660685815,-0.234843966119456,
-1.51495));
#52129=CARTESIAN_POINT('Ctrl Pts',(0.0138084231203835,-0.235560309102908,
-1.51495));
#52130=CARTESIAN_POINT('Ctrl Pts',(0.00959330062632784,-0.236214109276883,
-1.51495));
#52131=CARTESIAN_POINT('Ctrl Pts',(0.0053639592813879,-0.236757676588111,
-1.51495));
#52132=CARTESIAN_POINT('Ctrl Pts',(0.00112882195410514,-0.237190325076065,
-1.51495));
#52133=CARTESIAN_POINT('Ctrl Pts',(-0.0140084176727373,-0.23873669850631,
-1.51495));
#52134=CARTESIAN_POINT('Ctrl Pts',(-0.029232575277218,-0.238871978685379,
-1.51495));
#52135=CARTESIAN_POINT('Ctrl Pts',(-0.0443347748320724,-0.237560860275706,
-1.51495));
#52136=CARTESIAN_POINT('Ctrl Pts',(-0.0562275106107457,-0.23652837591711,
-1.51495));
#52137=CARTESIAN_POINT('Ctrl Pts',(-0.0680455301589941,-0.234598198295124,
-1.51495));
#52138=CARTESIAN_POINT('Ctrl Pts',(-0.0796899944392881,-0.23173046257725,
-1.51495));
#52139=CARTESIAN_POINT('Ctrl Pts',(0.197120364464142,0.0326678919976615,
-1.51495));
#52140=CARTESIAN_POINT('Ctrl Pts',(0.186733145342478,0.0934018504203839,
-1.51100164001845));
#52141=CARTESIAN_POINT('Ctrl Pts',(0.102816589942559,0.209511059178545,
-1.50281352242991));
#52142=CARTESIAN_POINT('Ctrl Pts',(-0.117789854919609,0.204361256460409,
-1.49038564723437));
#52143=CARTESIAN_POINT('Ctrl Pts',(-0.19826172011417,0.0726406085090636,
-1.48169916992909));
#52144=CARTESIAN_POINT('Ctrl Pts',(-0.199801535574945,0.00328497078691713,
-1.47725245023081));
#52145=CARTESIAN_POINT('Ctrl Pts',(-0.199789055725603,5.64207037231446E-5,
-1.47704548813952));
#52146=CARTESIAN_POINT('Origin',(-5.69858952725515E-17,8.58067791224701E-18,
-1.51495));
#52147=CARTESIAN_POINT('',(0.0326814423280644,0.196779569448552,-1.51495));
#52148=CARTESIAN_POINT('Ctrl Pts',(-0.232146081401957,-0.0797429895224413,
-1.51495));
#52149=CARTESIAN_POINT('Ctrl Pts',(-0.233507180164754,-0.0743161098729126,
-1.51495));
#52150=CARTESIAN_POINT('Ctrl Pts',(-0.234667146884371,-0.0688472205568463,
-1.51495));
#52151=CARTESIAN_POINT('Ctrl Pts',(-0.235618161880822,-0.0633432983169081,
-1.51495));
#52152=CARTESIAN_POINT('Ctrl Pts',(-0.237412919419644,-0.0529562844737211,
-1.51495));
#52153=CARTESIAN_POINT('Ctrl Pts',(-0.238464190995544,-0.0424443441387855,
-1.51495));
#52154=CARTESIAN_POINT('Ctrl Pts',(-0.238796731864267,-0.031878682006575,
-1.51495));
#52155=CARTESIAN_POINT('Ctrl Pts',(-0.238949768024948,-0.0270163371947305,
-1.51495));
#52156=CARTESIAN_POINT('Ctrl Pts',(-0.238950418479618,-0.0221426391101435,
-1.51495));
#52157=CARTESIAN_POINT('Ctrl Pts',(-0.238800286344163,-0.0172647716021107,
-1.51495));
#52158=CARTESIAN_POINT('Ctrl Pts',(-0.23864300623783,-0.0121546629767112,
-1.51495));
#52159=CARTESIAN_POINT('Ctrl Pts',(-0.238320478407458,-0.00704904230179029,
-1.51495));
#52160=CARTESIAN_POINT('Ctrl Pts',(-0.237836107021191,-0.00195869766834203,
-1.51495));
#52161=CARTESIAN_POINT('Ctrl Pts',(-0.236971804892792,0.00712440638305752,
-1.51495));
#52162=CARTESIAN_POINT('Ctrl Pts',(-0.235592459223133,0.0161619095527178,
-1.51495));
#52163=CARTESIAN_POINT('Ctrl Pts',(-0.23371173453278,0.0251065661509408,
-1.51495));
#52164=CARTESIAN_POINT('Ctrl Pts',(-0.232387557061457,0.0314043048985863,
-1.51495));
#52165=CARTESIAN_POINT('Ctrl Pts',(-0.230814689799066,0.0376559832384288,
-1.51495));
#52166=CARTESIAN_POINT('Ctrl Pts',(-0.228996136394989,0.0438440137987597,
-1.51495));
#52167=CARTESIAN_POINT('Ctrl Pts',(-0.227643249260427,0.0484475117848916,
-1.51495));
#52168=CARTESIAN_POINT('Ctrl Pts',(-0.226156705072274,0.0530074190901877,
-1.51495));
#52169=CARTESIAN_POINT('Ctrl Pts',(-0.224540759462049,0.0575117578727007,
-1.51495));
#52170=CARTESIAN_POINT('Ctrl Pts',(-0.219610975017165,0.0712531976365204,
-1.51495));
#52171=CARTESIAN_POINT('Ctrl Pts',(-0.213475147483757,0.0844959874752671,
-1.51495));
#52172=CARTESIAN_POINT('Ctrl Pts',(-0.206180399857752,0.097038108714997,
-1.51495));
#52173=CARTESIAN_POINT('Ctrl Pts',(-0.202999684165652,0.102506827289607,
-1.51495));
#52174=CARTESIAN_POINT('Ctrl Pts',(-0.199598120417428,0.107841928421567,
-1.51495));
#52175=CARTESIAN_POINT('Ctrl Pts',(-0.195977474949733,0.113024282643653,
-1.51495));
#52176=CARTESIAN_POINT('Ctrl Pts',(-0.193573374376874,0.116465354371122,
-1.51495));
#52177=CARTESIAN_POINT('Ctrl Pts',(-0.191072657180778,0.119839047867209,
-1.51495));
#52178=CARTESIAN_POINT('Ctrl Pts',(-0.188475578155228,0.123139297813982,
-1.51495));
#52179=CARTESIAN_POINT('Ctrl Pts',(-0.185966834432807,0.126327295273794,
-1.51495));
#52180=CARTESIAN_POINT('Ctrl Pts',(-0.183373651456097,0.129439708498115,
-1.51495));
#52181=CARTESIAN_POINT('Ctrl Pts',(-0.180699002448782,0.132469932176183,
-1.51495));
#52182=CARTESIAN_POINT('Ctrl Pts',(-0.175543696738069,0.138310597396014,
-1.51495));
#52183=CARTESIAN_POINT('Ctrl Pts',(-0.170083756237131,0.1438489438949,-1.51495));
#52184=CARTESIAN_POINT('Ctrl Pts',(-0.164325079865127,0.149051084203145,
-1.51495));
#52185=CARTESIAN_POINT('Ctrl Pts',(-0.153833986014853,0.158528286718191,
-1.51495));
#52186=CARTESIAN_POINT('Ctrl Pts',(-0.142351819020326,0.166892632944104,
-1.51495));
#52187=CARTESIAN_POINT('Ctrl Pts',(-0.130079371647154,0.174079981710603,
-1.51495));
#52188=CARTESIAN_POINT('Ctrl Pts',(-0.125535356483719,0.176741180474532,
-1.51495));
#52189=CARTESIAN_POINT('Ctrl Pts',(-0.120878783344098,0.179242125924473,
-1.51495));
#52190=CARTESIAN_POINT('Ctrl Pts',(-0.116145488887229,0.181566320250997,
-1.51495));
#52191=CARTESIAN_POINT('Ctrl Pts',(-0.104698309453902,0.187187240254196,
-1.51495));
#52192=CARTESIAN_POINT('Ctrl Pts',(-0.0927779625431565,0.191793755001339,
-1.51495));
#52193=CARTESIAN_POINT('Ctrl Pts',(-0.0805361366432621,0.195346249694064,
-1.51495));
#52194=CARTESIAN_POINT('Ctrl Pts',(-0.0695096699048282,0.198546055416519,
-1.51495));
#52195=CARTESIAN_POINT('Ctrl Pts',(-0.0582215637403063,0.20089035007889,
-1.51495));
#52196=CARTESIAN_POINT('Ctrl Pts',(-0.0467843784263279,0.202323822435583,
-1.51495));
#52197=CARTESIAN_POINT('Ctrl Pts',(-0.0426471497538938,0.202842359363371,
-1.51495));
#52198=CARTESIAN_POINT('Ctrl Pts',(-0.0384978685117633,0.203240408900611,
-1.51495));
#52199=CARTESIAN_POINT('Ctrl Pts',(-0.0343490085389219,0.20351577767736,
-1.51495));
#52200=CARTESIAN_POINT('Ctrl Pts',(-0.0213910546068069,0.204375825002844,
-1.51495));
#52201=CARTESIAN_POINT('Ctrl Pts',(-0.0084143667936003,0.204045484383494,
-1.51495));
#52202=CARTESIAN_POINT('Ctrl Pts',(0.0044149276201895,0.202455455781444,
-1.51495));
#52203=CARTESIAN_POINT('Ctrl Pts',(0.0139437527039043,0.201274478563339,
-1.51495));
#52204=CARTESIAN_POINT('Ctrl Pts',(0.0233913223400742,0.199397635842591,
-1.51495));
#52205=CARTESIAN_POINT('Ctrl Pts',(0.0326814423280607,0.196779569448552,
-1.51495));
#52206=CARTESIAN_POINT('Origin',(0.,0.,-1.51495));
#52207=CARTESIAN_POINT('Origin',(0.,0.,-1.69285451186048));
#52208=CARTESIAN_POINT('Ctrl Pts',(0.0326814423280649,0.196779569448552,
-1.51495));
#52209=CARTESIAN_POINT('Ctrl Pts',(-0.0328441439546247,0.207662155862942,
-1.51071024239301));
#52210=CARTESIAN_POINT('Ctrl Pts',(-0.15586916575445,0.16506957102402,-1.50334507967983));
#52211=CARTESIAN_POINT('Ctrl Pts',(-0.19892022304172,0.0488485439360305,
-1.49597991696666));
#52212=CARTESIAN_POINT('Ctrl Pts',(-0.199405781844198,-0.000173944371801573,
-1.49285451186048));
#52213=CARTESIAN_POINT('Ctrl Pts',(0.0401483265697123,0.241738731637385,
-1.54126273851832));
#52214=CARTESIAN_POINT('Ctrl Pts',(-0.0403482014090971,0.2551077142209,
-1.53702298091132));
#52215=CARTESIAN_POINT('Ctrl Pts',(-0.214347846184126,0.194867167024894,
-1.52854346569733));
#52216=CARTESIAN_POINT('Ctrl Pts',(-0.280010781085592,-0.0753312380677012,
-1.51582419287635));
#52217=CARTESIAN_POINT('Ctrl Pts',(-0.0881075174888988,-0.275964967577725,
-1.50310492005536));
#52218=CARTESIAN_POINT('Ctrl Pts',(0.184340118489057,-0.223572751555067,
-1.49038564723437));
#52219=CARTESIAN_POINT('Ctrl Pts',(0.28778640445331,0.0340957051198576,
-1.47766637441339));
#52220=CARTESIAN_POINT('Ctrl Pts',(0.127058169441575,0.260417170385679,
-1.4649471015924));
#52221=CARTESIAN_POINT('Ctrl Pts',(-0.150222375650171,0.247794607963362,
-1.45222782877142));
#52222=CARTESIAN_POINT('Ctrl Pts',(-0.289672761002644,0.00776434744478158,
-1.43950855595043));
#52223=CARTESIAN_POINT('Ctrl Pts',(-0.163289491859137,-0.239382486652227,
-1.42678928312944));
#52224=CARTESIAN_POINT('Ctrl Pts',(0.11293188259826,-0.266861686500435,
-1.41407001030846));
#52225=CARTESIAN_POINT('Ctrl Pts',(0.285523362567467,-0.0494498753666089,
-1.40135073748747));
#52226=CARTESIAN_POINT('Ctrl Pts',(0.196099310106758,0.213338956448214,
-1.38863146466649));
#52227=CARTESIAN_POINT('Ctrl Pts',(-0.0732765984215447,0.280355495930703,
-1.3759121918455));
#52228=CARTESIAN_POINT('Ctrl Pts',(-0.275409880441213,0.0901002704077519,
-1.36319291902451));
#52229=CARTESIAN_POINT('Ctrl Pts',(-0.224809881733275,-0.182836322382666,
-1.35047364620353));
#52230=CARTESIAN_POINT('Ctrl Pts',(0.0320893441203098,-0.287991164877318,
-1.33775437338254));
#52231=CARTESIAN_POINT('Ctrl Pts',(0.259541485891461,-0.128867571492712,
-1.32503510056156));
#52232=CARTESIAN_POINT('Ctrl Pts',(0.248822377267493,0.148512797676952,
-1.31231582774057));
#52233=CARTESIAN_POINT('Ctrl Pts',(0.00976858664482186,0.289608712370884,
-1.29959655491958));
#52234=CARTESIAN_POINT('Ctrl Pts',(-0.238249469334144,0.164941871833619,
-1.2868772820986));
#52235=CARTESIAN_POINT('Ctrl Pts',(-0.267635168780419,-0.111085760740929,
-1.27415800927761));
#52236=CARTESIAN_POINT('Ctrl Pts',(-0.0514223964570787,-0.285174276017006,
-1.26143873645663));
#52237=CARTESIAN_POINT('Ctrl Pts',(0.211978727731969,-0.197569353324888,
-1.24871946363564));
#52238=CARTESIAN_POINT('Ctrl Pts',(0.280855146490056,0.0713373462265733,
-1.23600019081465));
#52239=CARTESIAN_POINT('Ctrl Pts',(0.0920016273185971,0.274780514150071,
-1.22328091799367));
#52240=CARTESIAN_POINT('Ctrl Pts',(-0.18127823792608,0.226068199461604,
-1.21056164517268));
#52241=CARTESIAN_POINT('Ctrl Pts',(-0.288206054094843,-0.030098184743108,
-1.1978423723517));
#52242=CARTESIAN_POINT('Ctrl Pts',(-0.130658287529358,-0.258644625417178,
-1.18512309953071));
#52243=CARTESIAN_POINT('Ctrl Pts',(0.146789551427754,-0.249842866504755,
-1.17240382670972));
#52244=CARTESIAN_POINT('Ctrl Pts',(0.289534279139855,-0.011769942801552,
-1.15968455388874));
#52245=CARTESIAN_POINT('Ctrl Pts',(0.166584563160005,0.237103803574601,
-1.14696528106775));
#52246=CARTESIAN_POINT('Ctrl Pts',(-0.109233383036356,0.268396531986266,
-1.13424600824676));
#52247=CARTESIAN_POINT('Ctrl Pts',(-0.284812065591009,0.0533921122033667,
-1.12152673542578));
#52248=CARTESIAN_POINT('Ctrl Pts',(-0.199029697734655,-0.210608190181913,
-1.10880746260479));
#52249=CARTESIAN_POINT('Ctrl Pts',(0.0693945492688924,-0.281341477360996,
-1.09608818978381));
#52250=CARTESIAN_POINT('Ctrl Pts',(0.274138094219812,-0.0938985391229988,
-1.08336891696282));
#52251=CARTESIAN_POINT('Ctrl Pts',(0.22731568070417,0.17971146779753,-1.07064964414184));
#52252=CARTESIAN_POINT('Ctrl Pts',(-0.0281055678388845,0.288407190285495,
-1.05793037132085));
#52253=CARTESIAN_POINT('Ctrl Pts',(-0.257735420509811,0.132442755054978,
-1.04521109849987));
#52254=CARTESIAN_POINT('Ctrl Pts',(-0.250851415900536,-0.145059289577135,
-1.03249182567888));
#52255=CARTESIAN_POINT('Ctrl Pts',(-0.0137707395979083,-0.289446017562602,
-1.01977255285789));
#52256=CARTESIAN_POINT('Ctrl Pts',(0.23594681344234,-0.168219296093908,
-1.00705328003691));
#52257=CARTESIAN_POINT('Ctrl Pts',(0.269145073752699,0.107375786966052,
-0.994334007215921));
#52258=CARTESIAN_POINT('Ctrl Pts',(0.0553592779511471,0.28443625067254,
-0.981614734394934));
#52259=CARTESIAN_POINT('Ctrl Pts',(-0.209227592605962,0.200480534826297,
-0.968895461573949));
#52260=CARTESIAN_POINT('Ctrl Pts',(-0.281814369117759,-0.0674484374221064,
-0.956176188752962));
#52261=CARTESIAN_POINT('Ctrl Pts',(-0.0957909656814833,-0.273482579419117,
-0.943456915931977));
#52262=CARTESIAN_POINT('Ctrl Pts',(0.178136113319103,-0.228552303605735,
-0.93073764311099));
#52263=CARTESIAN_POINT('Ctrl Pts',(0.288594549947327,0.0261116083883038,
-0.918018370290005));
#52264=CARTESIAN_POINT('Ctrl Pts',(0.134220896119848,0.256813904212193,
-0.905299097469018));
#52265=CARTESIAN_POINT('Ctrl Pts',(-0.143322098600399,0.25184798272907,
-0.892579824648033));
#52266=CARTESIAN_POINT('Ctrl Pts',(-0.289343929848329,0.0157708786010744,
-0.879860551827046));
#52267=CARTESIAN_POINT('Ctrl Pts',(-0.16984599360104,-0.234778552703606,
-0.867141279006061));
#52268=CARTESIAN_POINT('Ctrl Pts',(0.105513061815336,-0.269880759110903,
-0.854422006185075));
#52269=CARTESIAN_POINT('Ctrl Pts',(0.284046848923501,-0.0573237993206493,
-0.841702733364088));
#52270=CARTESIAN_POINT('Ctrl Pts',(0.201921795448932,0.207837000735201,
-0.828983460543103));
#52271=CARTESIAN_POINT('Ctrl Pts',(-0.0654991037270535,0.282273799285157,
-0.816264187722116));
#52272=CARTESIAN_POINT('Ctrl Pts',(-0.27281400101847,0.0976788165377675,
-0.803544914901131));
#52273=CARTESIAN_POINT('Ctrl Pts',(-0.22977800911779,-0.176552249710359,
-0.790825642080144));
#52274=CARTESIAN_POINT('Ctrl Pts',(0.0241164016494981,-0.288768124147047,
-0.778106369259159));
#52275=CARTESIAN_POINT('Ctrl Pts',(0.255880120536876,-0.135992625777865,
-0.765387096438172));
#52276=CARTESIAN_POINT('Ctrl Pts',(0.252832519389947,0.141578061474426,
-0.752667823617187));
#52277=CARTESIAN_POINT('Ctrl Pts',(0.017770264267596,0.28922802087589,-0.7399485507962));
#52278=CARTESIAN_POINT('Ctrl Pts',(-0.233599077162506,0.171464577976764,
-0.727229277975216));
#52279=CARTESIAN_POINT('Ctrl Pts',(-0.270603552919432,-0.103645296561416,
-0.714510005154228));
#52280=CARTESIAN_POINT('Ctrl Pts',(-0.0592855824712138,-0.283643878945013,
-0.701790732333244));
#52281=CARTESIAN_POINT('Ctrl Pts',(0.206436480994706,-0.203353410756857,
-0.689071459512256));
#52282=CARTESIAN_POINT('Ctrl Pts',(0.282719745917391,0.0635466412985803,
-0.676352186691271));
#52283=CARTESIAN_POINT('Ctrl Pts',(0.0995620015137612,0.272132390954289,
-0.663632913870285));
#52284=CARTESIAN_POINT('Ctrl Pts',(-0.174959952628603,0.230992738691331,
-0.650913641049299));
#52285=CARTESIAN_POINT('Ctrl Pts',(-0.288927904593446,-0.0221200429286395,
-0.638194368228313));
#52286=CARTESIAN_POINT('Ctrl Pts',(-0.137757859397795,-0.254934114088448,
-0.625475095407327));
#52287=CARTESIAN_POINT('Ctrl Pts',(0.139827261507635,-0.253804978854237,
-0.612755822586341));
#52288=CARTESIAN_POINT('Ctrl Pts',(0.289098296181977,-0.0197688010916725,
-0.600036549765355));
#52289=CARTESIAN_POINT('Ctrl Pts',(0.173074971905226,0.23240844315973,-0.587317276944369));
#52290=CARTESIAN_POINT('Ctrl Pts',(-0.101772580422917,0.271313420652177,
-0.574598004123382));
#52291=CARTESIAN_POINT('Ctrl Pts',(-0.283227359985977,0.0612445336932068,
-0.561878731302398));
#52292=CARTESIAN_POINT('Ctrl Pts',(-0.204775312365271,-0.205026100283915,
-0.54915945848141));
#52293=CARTESIAN_POINT('Ctrl Pts',(0.0615911434010899,-0.283152187712668,
-0.536440185660426));
#52294=CARTESIAN_POINT('Ctrl Pts',(0.271437781785443,-0.101440430654277,
-0.523720912839439));
#52295=CARTESIAN_POINT('Ctrl Pts',(0.232196434301655,0.173359298134017,
-0.511001640018453));
#52296=CARTESIAN_POINT('Ctrl Pts',(-0.0201226275869376,0.289073883654192,
-0.498282367197468));
#52297=CARTESIAN_POINT('Ctrl Pts',(-0.253975930055376,0.139516512658715,
-0.48556309437648));
#52298=CARTESIAN_POINT('Ctrl Pts',(-0.25476531466985,-0.138069782331531,
-0.472843821555496));
#52299=CARTESIAN_POINT('Ctrl Pts',(-0.0217663936081401,-0.288954761963176,
-0.460124548734509));
#52300=CARTESIAN_POINT('Ctrl Pts',(0.231206707569178,-0.174677098461904,
-0.447405275913524));
#52301=CARTESIAN_POINT('Ctrl Pts',(0.272010328400097,0.0998950028551257,
-0.434686003092537));
#52302=CARTESIAN_POINT('Ctrl Pts',(0.0632005594130015,0.28279731194215,
-0.421966730271552));
#52303=CARTESIAN_POINT('Ctrl Pts',(-0.203605925974667,0.206187432354038,
-0.409247457450565));
#52304=CARTESIAN_POINT('Ctrl Pts',(-0.283571104011678,-0.0596327034452211,
-0.39652818462958));
#52305=CARTESIAN_POINT('Ctrl Pts',(-0.103314014236298,-0.270730206689346,
-0.383808911808593));
#52306=CARTESIAN_POINT('Ctrl Pts',(0.171750362695484,-0.23338903845568,
-0.371089638987607));
#52307=CARTESIAN_POINT('Ctrl Pts',(0.28920605433811,0.0181242510447194,
-0.358370366166621));
#52308=CARTESIAN_POINT('Ctrl Pts',(0.141268501588536,0.253005614191318,
-0.345651093345636));
#52309=CARTESIAN_POINT('Ctrl Pts',(-0.136305707962405,0.255713480995264,
-0.332931820524649));
#52310=CARTESIAN_POINT('Ctrl Pts',(-0.288797424950404,0.0237629463370206,
-0.320212547703663));
#52311=CARTESIAN_POINT('Ctrl Pts',(-0.176270881356031,-0.229993927680813,
-0.307493274882677));
#52312=CARTESIAN_POINT('Ctrl Pts',(0.0980126540007645,-0.272694243090937,
-0.294774002061692));
#52313=CARTESIAN_POINT('Ctrl Pts',(0.282353754487939,-0.0651535657817629,
-0.282054729240705));
#52314=CARTESIAN_POINT('Ctrl Pts',(0.207589704923852,0.202176025115757,
-0.26933545641972));
#52315=CARTESIAN_POINT('Ctrl Pts',(-0.0576714181337695,0.283976476308512,
-0.256616183598733));
#52316=CARTESIAN_POINT('Ctrl Pts',(-0.270009693456009,0.10518265989541,
-0.243896910777747));
#52317=CARTESIAN_POINT('Ctrl Pts',(-0.234570505638583,-0.170133217702001,
-0.231177637956762));
#52318=CARTESIAN_POINT('Ctrl Pts',(0.0161250305881685,-0.289324420749436,
-0.218458365135775));
#52319=CARTESIAN_POINT('Ctrl Pts',(0.25202317124219,-0.143013722643587,
-0.20573909231479));
#52320=CARTESIAN_POINT('Ctrl Pts',(0.256649511832594,0.134535084822825,
-0.193019819493804));
#52321=CARTESIAN_POINT('Ctrl Pts',(0.0257582127796514,0.288626364785306,
-0.180300546672817));
#52322=CARTESIAN_POINT('Ctrl Pts',(-0.228769873386647,0.177856106989376,
-0.167581273851832));
#52323=CARTESIAN_POINT('Ctrl Pts',(-0.273365681038595,-0.0961253617725913,
-0.154862001030846));
#52324=CARTESIAN_POINT('Ctrl Pts',(-0.0671024131868596,-0.281897208169119,
-0.14214272820986));
#52325=CARTESIAN_POINT('Ctrl Pts',(0.200734471793731,-0.20898111135007,
-0.129423455388874));
#52326=CARTESIAN_POINT('Ctrl Pts',(0.284372086079907,0.0557055671966431,
-0.116704182567887));
#52327=CARTESIAN_POINT('Ctrl Pts',(0.107039034186323,0.269279733812547,
-0.103984909746902));
#52328=CARTESIAN_POINT('Ctrl Pts',(-0.168494133032722,0.235734189686348,
-0.0912656369259156));
#52329=CARTESIAN_POINT('Ctrl Pts',(-0.289455297174828,-0.014112499183932,
-0.0785463641049299));
#52330=CARTESIAN_POINT('Ctrl Pts',(-0.144701892960455,-0.251052617385527,
-0.0658270912839438));
#52331=CARTESIAN_POINT('Ctrl Pts',(0.132662010889486,-0.257527452585136,
-0.0531078184629578));
#52332=CARTESIAN_POINT('Ctrl Pts',(0.288627233657158,-0.0278415686410112,
-0.0403885456419716));
#52333=CARTESIAN_POINT('Ctrl Pts',(0.17905539955801,0.227722146128134,-0.0276692728209858));
#52334=CARTESIAN_POINT('Ctrl Pts',(-0.00252611781081248,0.258266416594894,
-0.0191897576069951));
#52335=CARTESIAN_POINT('Ctrl Pts',(-0.0796899944392906,0.231730462577249,
-0.0149499999999998));
#52336=CARTESIAN_POINT('Ctrl Pts',(0.0376593651558298,0.226752344241107,
-1.53249182567888));
#52337=CARTESIAN_POINT('Ctrl Pts',(-0.0378468489242729,0.239292528101581,
-1.52825206807188));
#52338=CARTESIAN_POINT('Ctrl Pts',(-0.201059533472651,0.182786542475944,
-1.51977255285789));
#52339=CARTESIAN_POINT('Ctrl Pts',(-0.262651750482346,-0.0706611419309478,
-1.50705328003691));
#52340=CARTESIAN_POINT('Ctrl Pts',(-0.0826453667583571,-0.258856753747412,
-1.49433400721592));
#52341=CARTESIAN_POINT('Ctrl Pts',(0.172912109375083,-0.209712548668413,
-1.48161473439494));
#52342=CARTESIAN_POINT('Ctrl Pts',(0.269945330682025,0.0319819708332,-1.46889546157395));
#52343=CARTESIAN_POINT('Ctrl Pts',(0.119181306118034,0.244272829039931,
-1.45617618875296));
#52344=CARTESIAN_POINT('Ctrl Pts',(-0.140909467032535,0.23243279165658,
-1.44345691593198));
#52345=CARTESIAN_POINT('Ctrl Pts',(-0.271714744158876,0.00728300331800845,
-1.43073764311099));
#52346=CARTESIAN_POINT('Ctrl Pts',(-0.153166498468018,-0.224542172663008,
-1.41801837029));
#52347=CARTESIAN_POINT('Ctrl Pts',(0.105930766432288,-0.250317822850489,
-1.40529909746902));
#52348=CARTESIAN_POINT('Ctrl Pts',(0.267822584156242,-0.0463842723334394,
-1.39257982464803));
#52349=CARTESIAN_POINT('Ctrl Pts',(0.183942299893718,0.200113188999222,
-1.37986055182705));
#52350=CARTESIAN_POINT('Ctrl Pts',(-0.0687338779249646,0.262975095023348,
-1.36714127900606));
#52351=CARTESIAN_POINT('Ctrl Pts',(-0.258336078766579,0.0845145806521449,
-1.35442200618507));
#52352=CARTESIAN_POINT('Ctrl Pts',(-0.210872984011728,-0.171501539831365,
-1.34170273336409));
#52353=CARTESIAN_POINT('Ctrl Pts',(0.0300999924801246,-0.270137397157419,
-1.3289834605431));
#52354=CARTESIAN_POINT('Ctrl Pts',(0.243451431862348,-0.120878535825459,
-1.31626418772212));
#52355=CARTESIAN_POINT('Ctrl Pts',(0.233396845275428,0.139305872894083,
-1.30354491490113));
#52356=CARTESIAN_POINT('Ctrl Pts',(0.009162991410735,0.271654666167656,
-1.29082564208014));
#52357=CARTESIAN_POINT('Ctrl Pts',(-0.223479395791461,0.154716440549094,
-1.27810636925916));
#52358=CARTESIAN_POINT('Ctrl Pts',(-0.251043353753325,-0.104199093331874,
-1.26538709643817));
#52359=CARTESIAN_POINT('Ctrl Pts',(-0.048234508653865,-0.267495138930051,
-1.25266782361719));
#52360=CARTESIAN_POINT('Ctrl Pts',(0.198837286507208,-0.185321209030822,
-1.2399485507962));
#52361=CARTESIAN_POINT('Ctrl Pts',(0.26344377017055,0.0669148480231117,
-1.22722927797521));
#52362=CARTESIAN_POINT('Ctrl Pts',(0.0862980645558325,0.257745729504231,
-1.21451000515423));
#52363=CARTESIAN_POINT('Ctrl Pts',(-0.170040047497623,0.212053293400986,
-1.20179073233324));
#52364=CARTESIAN_POINT('Ctrl Pts',(-0.270338964500376,-0.0282322733377271,
-1.18907145951226));
#52365=CARTESIAN_POINT('Ctrl Pts',(-0.122558237941992,-0.242610171491602,
-1.17635218669127));
#52366=CARTESIAN_POINT('Ctrl Pts',(0.137689457832816,-0.234354070148971,
-1.16363291387029));
#52367=CARTESIAN_POINT('Ctrl Pts',(0.271584847361581,-0.011040275191973,
-1.1509136410493));
#52368=CARTESIAN_POINT('Ctrl Pts',(0.156257294621586,0.222404754607843,
-1.13819436822831));
#52369=CARTESIAN_POINT('Ctrl Pts',(-0.102461552210156,0.251757516893735,
-1.12547509540732));
#52370=CARTESIAN_POINT('Ctrl Pts',(-0.267155383431844,0.0500821135450386,
-1.11275582258634));
#52371=CARTESIAN_POINT('Ctrl Pts',(-0.186691020628951,-0.19755171426878,
-1.10003654976535));
#52372=CARTESIAN_POINT('Ctrl Pts',(0.0650924931131031,-0.263899951372112,
-1.08731727694437));
#52373=CARTESIAN_POINT('Ctrl Pts',(0.25714313585204,-0.0880773789236763,
-1.07459800412338));
#52374=CARTESIAN_POINT('Ctrl Pts',(0.213223438103214,0.168570407952775,
-1.0618787313024));
#52375=CARTESIAN_POINT('Ctrl Pts',(-0.0263631870264576,0.270527631423682,
-1.04915945848141));
#52376=CARTESIAN_POINT('Ctrl Pts',(-0.241757331970419,0.124232078918636,
-1.03644018566043));
#52377=CARTESIAN_POINT('Ctrl Pts',(-0.235300095381367,-0.13606646209638,
-1.02372091283944));
#52378=CARTESIAN_POINT('Ctrl Pts',(-0.0129170342899085,-0.271502057485862,
-1.01100164001845));
#52379=CARTESIAN_POINT('Ctrl Pts',(0.221319491096378,-0.15779068367538,
-0.998282367197467));
#52380=CARTESIAN_POINT('Ctrl Pts',(0.252459653448979,0.100719116230859,
-0.985563094376481));
#52381=CARTESIAN_POINT('Ctrl Pts',(0.0519273265226976,0.266802866840123,
-0.972843821555495));
#52382=CARTESIAN_POINT('Ctrl Pts',(-0.19625670566722,0.188051914307071,
-0.96012454873451));
#52383=CARTESIAN_POINT('Ctrl Pts',(-0.264343526605969,-0.0632670288177248,
-0.947405275913523));
#52384=CARTESIAN_POINT('Ctrl Pts',(-0.0898524861046148,-0.256528259134786,
-0.934686003092538));
#52385=CARTESIAN_POINT('Ctrl Pts',(0.167092716237531,-0.21438339761807,
-0.921966730271551));
#52386=CARTESIAN_POINT('Ctrl Pts',(0.270703375882375,0.0244928413988521,
-0.909247457450566));
#52387=CARTESIAN_POINT('Ctrl Pts',(0.125899985638092,0.240892944293169,
-0.896528184629579));
#52388=CARTESIAN_POINT('Ctrl Pts',(-0.134436966799118,0.236234880895597,
-0.883808911808593));
#52389=CARTESIAN_POINT('Ctrl Pts',(-0.271406298612747,0.014793176373984,
-0.871089638987608));
#52390=CARTESIAN_POINT('Ctrl Pts',(-0.159316535451862,-0.220223655690117,
-0.858370366166621));
#52391=CARTESIAN_POINT('Ctrl Pts',(0.0989718691441357,-0.253149730618106,
-0.845651093345636));
#52392=CARTESIAN_POINT('Ctrl Pts',(0.266437605721858,-0.0537700590580635,
-0.832931820524649));
#52393=CARTESIAN_POINT('Ctrl Pts',(0.189403825201247,0.194952322358671,
-0.820212547703663));
#52394=CARTESIAN_POINT('Ctrl Pts',(-0.0614385424098267,0.264774474790263,
-0.807493274882678));
#52395=CARTESIAN_POINT('Ctrl Pts',(-0.255901128684366,0.0916233012501255,
-0.794774002061691));
#52396=CARTESIAN_POINT('Ctrl Pts',(-0.215533116557709,-0.16560704290828,
-0.782054729240706));
#52397=CARTESIAN_POINT('Ctrl Pts',(0.0226213258075957,-0.270866189496973,
-0.769335456419719));
#52398=CARTESIAN_POINT('Ctrl Pts',(0.240017049743885,-0.127561878420417,
-0.756616183598734));
#52399=CARTESIAN_POINT('Ctrl Pts',(0.237158382042199,0.132801049773826,
-0.743896910777747));
#52400=CARTESIAN_POINT('Ctrl Pts',(0.016668611823881,0.271297575318631,
-0.731177637956762));
#52401=CARTESIAN_POINT('Ctrl Pts',(-0.21911730073364,0.160834777063628,
-0.718458365135776));
#52402=CARTESIAN_POINT('Ctrl Pts',(-0.253827715438233,-0.097219894411127,
-0.70573909231479));
#52403=CARTESIAN_POINT('Ctrl Pts',(-0.0556102231280499,-0.266059617525005,
-0.693019819493804));
#52404=CARTESIAN_POINT('Ctrl Pts',(0.193638626650242,-0.190746688733808,
-0.680300546672818));
#52405=CARTESIAN_POINT('Ctrl Pts',(0.265192775339705,0.0596071212316804,
-0.667581273851832));
#52406=CARTESIAN_POINT('Ctrl Pts',(0.0933897397726324,0.255261774457328,
-0.654862001030846));
#52407=CARTESIAN_POINT('Ctrl Pts',(-0.164113458932014,0.216672540002821,
-0.64214272820986));
#52408=CARTESIAN_POINT('Ctrl Pts',(-0.271016064490275,-0.0207487296504358,
-0.629423455388874));
#52409=CARTESIAN_POINT('Ctrl Pts',(-0.129217677881022,-0.239129690161929,
-0.616704182567888));
#52410=CARTESIAN_POINT('Ctrl Pts',(0.131158789164291,-0.23807055470776,
-0.603984909746902));
#52411=CARTESIAN_POINT('Ctrl Pts',(0.271175892796963,-0.0185432510545995,
-0.591265636925916));
#52412=CARTESIAN_POINT('Ctrl Pts',(0.162345335987956,0.218000479074844,
-0.57854636410493));
#52413=CARTESIAN_POINT('Ctrl Pts',(-0.0954632757194232,0.254493575523668,
-0.565827091283944));
#52414=CARTESIAN_POINT('Ctrl Pts',(-0.265668920305149,0.0574477308324719,
-0.553107818462958));
#52415=CARTESIAN_POINT('Ctrl Pts',(-0.19208044075941,-0.192315681293997,
-0.540388545641972));
#52416=CARTESIAN_POINT('Ctrl Pts',(0.0577728527658405,-0.265598408273091,
-0.527669272820986));
#52417=CARTESIAN_POINT('Ctrl Pts',(0.254610226994079,-0.0951517172936434,
-0.51495));
#52418=CARTESIAN_POINT('Ctrl Pts',(0.217801613525897,0.16261203565363,-0.502230727179015));
#52419=CARTESIAN_POINT('Ctrl Pts',(-0.0188751423767444,0.271152993703107,
-0.489511454358028));
#52420=CARTESIAN_POINT('Ctrl Pts',(-0.238230907934349,0.130867304926385,
-0.476792181537042));
#52421=CARTESIAN_POINT('Ctrl Pts',(-0.238971355319949,-0.129510263417352,
-0.464072908716056));
#52422=CARTESIAN_POINT('Ctrl Pts',(-0.0204170045192572,-0.271041256860175,
-0.45135363589507));
#52423=CARTESIAN_POINT('Ctrl Pts',(0.216873244061779,-0.163848140069192,
-0.438634363074084));
#52424=CARTESIAN_POINT('Ctrl Pts',(0.255147279067533,0.0937020969786091,
-0.425915090253098));
#52425=CARTESIAN_POINT('Ctrl Pts',(0.0592824943987202,0.265265532724626,
-0.413195817432112));
#52426=CARTESIAN_POINT('Ctrl Pts',(-0.190983549485114,0.193405017568571,
-0.400476544611126));
#52427=CARTESIAN_POINT('Ctrl Pts',(-0.265991354211865,-0.0559358246320336,
-0.38775727179014));
#52428=CARTESIAN_POINT('Ctrl Pts',(-0.0969091496524436,-0.25394651741523,
-0.375037998969154));
#52429=CARTESIAN_POINT('Ctrl Pts',(0.161102844801386,-0.218920283198089,
-0.362318726148168));
#52430=CARTESIAN_POINT('Ctrl Pts',(0.271276970577709,0.0170006534913469,
-0.349599453327182));
#52431=CARTESIAN_POINT('Ctrl Pts',(0.132510680790197,0.237320745978342,
-0.336880180506196));
#52432=CARTESIAN_POINT('Ctrl Pts',(-0.127855551340783,0.239860740879152,
-0.32416090768521));
#52433=CARTESIAN_POINT('Ctrl Pts',(-0.270893673821908,0.0222897826570762,
-0.311441634864224));
#52434=CARTESIAN_POINT('Ctrl Pts',(-0.165343117746152,-0.215735649432766,
-0.298722362043238));
#52435=CARTESIAN_POINT('Ctrl Pts',(0.0919364427430842,-0.255788795047858,
-0.286003089222253));
#52436=CARTESIAN_POINT('Ctrl Pts',(0.264849473238144,-0.0611144257960386,
-0.273283816401266));
#52437=CARTESIAN_POINT('Ctrl Pts',(0.194720357441154,0.189642294115757,
-0.260564543580281));
#52438=CARTESIAN_POINT('Ctrl Pts',(-0.0540961275380471,0.266371595797377,
-0.247845270759294));
#52439=CARTESIAN_POINT('Ctrl Pts',(-0.253270671787972,0.0986619502106732,
-0.235125997938308));
#52440=CARTESIAN_POINT('Ctrl Pts',(-0.220028506326227,-0.159585953338581,
-0.222406725117323));
#52441=CARTESIAN_POINT('Ctrl Pts',(0.0151253730093691,-0.271387998963875,
-0.209687452296336));
#52442=CARTESIAN_POINT('Ctrl Pts',(0.236399208745608,-0.134147708347888,
-0.196968179475351));
#52443=CARTESIAN_POINT('Ctrl Pts',(0.240738743279549,0.126194696479222,
-0.184248906654364));
#52444=CARTESIAN_POINT('Ctrl Pts',(0.0241613542508698,0.27073321838649,
-0.171529633833378));
#52445=CARTESIAN_POINT('Ctrl Pts',(-0.214587479345165,0.166830068662447,
-0.158810361012393));
#52446=CARTESIAN_POINT('Ctrl Pts',(-0.2564186077701,-0.0901661515940091,
-0.146091088191407));
#52447=CARTESIAN_POINT('Ctrl Pts',(-0.0629424560611133,-0.264421230120684,
-0.133371815370421));
#52448=CARTESIAN_POINT('Ctrl Pts',(0.188290108667841,-0.196025504807486,
-0.120652542549435));
#52449=CARTESIAN_POINT('Ctrl Pts',(0.266742680076926,0.0522521478604723,
-0.107933269728448));
#52450=CARTESIAN_POINT('Ctrl Pts',(0.100403240153755,0.252585965372765,
-0.0952139969074626));
#52451=CARTESIAN_POINT('Ctrl Pts',(-0.158048482331552,0.221120048769588,
-0.0824947240864768));
#52452=CARTESIAN_POINT('Ctrl Pts',(-0.271510761816407,-0.013237606780604,
-0.0697754512654906));
#52453=CARTESIAN_POINT('Ctrl Pts',(-0.135731221979467,-0.235488823551147,
-0.0570561784445049));
#52454=CARTESIAN_POINT('Ctrl Pts',(0.124437742173868,-0.241562256840637,
-0.0443369056235188));
#52455=CARTESIAN_POINT('Ctrl Pts',(0.270734033393368,-0.0261155542346787,
-0.0316176328025325));
#52456=CARTESIAN_POINT('Ctrl Pts',(0.167955012106663,0.213604705048369,
-0.0188983599815468));
#52457=CARTESIAN_POINT('Ctrl Pts',(-0.00236951328217672,0.2422554094041,
-0.0104188447675561));
#52458=CARTESIAN_POINT('Ctrl Pts',(-0.0747496809025027,0.217364529322868,
-0.00617908716056078));
#52459=CARTESIAN_POINT('Ctrl Pts',(0.0351704037419473,0.21176595684483,
-1.52372091283944));
#52460=CARTESIAN_POINT('Ctrl Pts',(-0.0353454964394489,0.223477341982261,
-1.51948115523244));
#52461=CARTESIAN_POINT('Ctrl Pts',(-0.187771220761176,0.170705917926994,
-1.51100164001845));
#52462=CARTESIAN_POINT('Ctrl Pts',(-0.2452927198791,-0.0659910457941944,
-1.49828236719747));
#52463=CARTESIAN_POINT('Ctrl Pts',(-0.0771832160278151,-0.2417485399171,
-1.48556309437648));
#52464=CARTESIAN_POINT('Ctrl Pts',(0.161484100261109,-0.19585234578176,
-1.47284382155549));
#52465=CARTESIAN_POINT('Ctrl Pts',(0.252104256910741,0.0298682365465424,
-1.46012454873451));
#52466=CARTESIAN_POINT('Ctrl Pts',(0.111304442794493,0.228128487694183,
-1.44740527591352));
#52467=CARTESIAN_POINT('Ctrl Pts',(-0.131596558414898,0.217070975349797,
-1.43468600309254));
#52468=CARTESIAN_POINT('Ctrl Pts',(-0.253756727315109,0.00680165919123546,
-1.42196673027155));
#52469=CARTESIAN_POINT('Ctrl Pts',(-0.143043505076898,-0.209701858673789,
-1.40924745745057));
#52470=CARTESIAN_POINT('Ctrl Pts',(0.0989296502663155,-0.233773959200543,
-1.39652818462958));
#52471=CARTESIAN_POINT('Ctrl Pts',(0.250121805745017,-0.04331866930027,
-1.38380891180859));
#52472=CARTESIAN_POINT('Ctrl Pts',(0.171785289680678,0.18688742155023,-1.37108963898761));
#52473=CARTESIAN_POINT('Ctrl Pts',(-0.0641911574283849,0.245594694115993,
-1.35837036616662));
#52474=CARTESIAN_POINT('Ctrl Pts',(-0.241262277091944,0.0789288908965379,
-1.34565109334564));
#52475=CARTESIAN_POINT('Ctrl Pts',(-0.196936086290182,-0.160166757280064,
-1.33293182052465));
#52476=CARTESIAN_POINT('Ctrl Pts',(0.0281106408399401,-0.25228362943752,
-1.32021254770367));
#52477=CARTESIAN_POINT('Ctrl Pts',(0.227361377833234,-0.112889500158205,
-1.30749327488268));
#52478=CARTESIAN_POINT('Ctrl Pts',(0.217971313283363,0.130098948111214,
-1.29477400206169));
#52479=CARTESIAN_POINT('Ctrl Pts',(0.00855739617664794,0.253700619964428,
-1.2820547292407));
#52480=CARTESIAN_POINT('Ctrl Pts',(-0.208709322248779,0.14449100926457,
-1.26933545641972));
#52481=CARTESIAN_POINT('Ctrl Pts',(-0.234451538726231,-0.0973124259228192,
-1.25661618359873));
#52482=CARTESIAN_POINT('Ctrl Pts',(-0.0450466208506513,-0.249816001843096,
-1.24389691077775));
#52483=CARTESIAN_POINT('Ctrl Pts',(0.185695845282446,-0.173073064736756,
-1.23117763795676));
#52484=CARTESIAN_POINT('Ctrl Pts',(0.246032393851044,0.0624923498196499,
-1.21845836513578));
#52485=CARTESIAN_POINT('Ctrl Pts',(0.0805945017930683,0.240710944858392,
-1.20573909231479));
#52486=CARTESIAN_POINT('Ctrl Pts',(-0.158801857069166,0.198038387340367,
-1.19301981949381));
#52487=CARTESIAN_POINT('Ctrl Pts',(-0.252471874905908,-0.026366361932346,
-1.18030054667282));
#52488=CARTESIAN_POINT('Ctrl Pts',(-0.114458188354627,-0.226575717566026,
-1.16758127385183));
#52489=CARTESIAN_POINT('Ctrl Pts',(0.128589364237878,-0.218865273793187,
-1.15486200103085));
#52490=CARTESIAN_POINT('Ctrl Pts',(0.253635415583305,-0.0103106075823939,
-1.14214272820986));
#52491=CARTESIAN_POINT('Ctrl Pts',(0.145930026083168,0.207705705641086,
-1.12942345538887));
#52492=CARTESIAN_POINT('Ctrl Pts',(-0.0956897213839561,0.235118501801203,
-1.11670418256789));
#52493=CARTESIAN_POINT('Ctrl Pts',(-0.24949870127268,0.0467721148867109,
-1.1039849097469));
#52494=CARTESIAN_POINT('Ctrl Pts',(-0.174352343523248,-0.184495238355647,
-1.09126563692592));
#52495=CARTESIAN_POINT('Ctrl Pts',(0.0607904369573136,-0.246458425383229,
-1.07854636410493));
#52496=CARTESIAN_POINT('Ctrl Pts',(0.240148177484268,-0.0822562187243539,
-1.06582709128394));
#52497=CARTESIAN_POINT('Ctrl Pts',(0.199131195502257,0.15742934810802,-1.05310781846296));
#52498=CARTESIAN_POINT('Ctrl Pts',(-0.0246208062140303,0.252648072561869,
-1.04038854564197));
#52499=CARTESIAN_POINT('Ctrl Pts',(-0.225779243431027,0.116021402782294,
-1.02766927282099));
#52500=CARTESIAN_POINT('Ctrl Pts',(-0.219748774862197,-0.127073634615625,
-1.01495));
#52501=CARTESIAN_POINT('Ctrl Pts',(-0.0120633289819088,-0.253558097409122,
-1.00223072717902));
#52502=CARTESIAN_POINT('Ctrl Pts',(0.206692168750416,-0.147362071256852,
-0.989511454358028));
#52503=CARTESIAN_POINT('Ctrl Pts',(0.235774233145259,0.0940624454956667,
-0.976792181537043));
#52504=CARTESIAN_POINT('Ctrl Pts',(0.0484953750942479,0.249169483007708,
-0.964072908716057));
#52505=CARTESIAN_POINT('Ctrl Pts',(-0.183285818728479,0.175623293787844,
-0.951353635895069));
#52506=CARTESIAN_POINT('Ctrl Pts',(-0.24687268409418,-0.059085620213343,
-0.938634363074085));
#52507=CARTESIAN_POINT('Ctrl Pts',(-0.0839140065277464,-0.239573938850455,
-0.925915090253097));
#52508=CARTESIAN_POINT('Ctrl Pts',(0.15604931915596,-0.200214491630405,
-0.913195817432113));
#52509=CARTESIAN_POINT('Ctrl Pts',(0.252812201817423,0.0228740744094001,
-0.900476544611126));
#52510=CARTESIAN_POINT('Ctrl Pts',(0.117579075156335,0.224971984374146,
-0.887757271790141));
#52511=CARTESIAN_POINT('Ctrl Pts',(-0.125551834997836,0.220621779062123,
-0.875037998969154));
#52512=CARTESIAN_POINT('Ctrl Pts',(-0.253468667377166,0.0138154741468941,
-0.862318726148169));
#52513=CARTESIAN_POINT('Ctrl Pts',(-0.148787077302684,-0.205668758676629,
-0.849599453327182));
#52514=CARTESIAN_POINT('Ctrl Pts',(0.0924306764729358,-0.236418702125309,
-0.836880180506197));
#52515=CARTESIAN_POINT('Ctrl Pts',(0.248828362520214,-0.0502163187954781,
-0.82416090768521));
#52516=CARTESIAN_POINT('Ctrl Pts',(0.176885854953561,0.182067643982142,
-0.811441634864225));
#52517=CARTESIAN_POINT('Ctrl Pts',(-0.0573779810926002,0.247275150295369,
-0.798722362043238));
#52518=CARTESIAN_POINT('Ctrl Pts',(-0.238988256350262,0.0855677859624836,
-0.786003089222252));
#52519=CARTESIAN_POINT('Ctrl Pts',(-0.201288223997627,-0.1546618361062,
-0.773283816401267));
#52520=CARTESIAN_POINT('Ctrl Pts',(0.0211262499656935,-0.252964254846899,
-0.76056454358028));
#52521=CARTESIAN_POINT('Ctrl Pts',(0.224153978950893,-0.11913113106297,
-0.747845270759295));
#52522=CARTESIAN_POINT('Ctrl Pts',(0.22148424469445,0.124024038073226,-0.735125997938308));
#52523=CARTESIAN_POINT('Ctrl Pts',(0.0155669593801661,0.253367129761373,
-0.722406725117323));
#52524=CARTESIAN_POINT('Ctrl Pts',(-0.204635524304775,0.150204976150491,
-0.709687452296336));
#52525=CARTESIAN_POINT('Ctrl Pts',(-0.237051877957034,-0.0907944922608373,
-0.696968179475351));
#52526=CARTESIAN_POINT('Ctrl Pts',(-0.0519348637848862,-0.248475356104998,
-0.684248906654364));
#52527=CARTESIAN_POINT('Ctrl Pts',(0.180840772305777,-0.178139966710758,
-0.671529633833379));
#52528=CARTESIAN_POINT('Ctrl Pts',(0.24766580476202,0.0556676011647803,
-0.658810361012393));
#52529=CARTESIAN_POINT('Ctrl Pts',(0.0872174780315035,0.238391157960366,
-0.646091088191407));
#52530=CARTESIAN_POINT('Ctrl Pts',(-0.153266965235425,0.202352341314311,
-0.633371815370422));
#52531=CARTESIAN_POINT('Ctrl Pts',(-0.253104224387104,-0.019377416372232,
-0.620652542549434));
#52532=CARTESIAN_POINT('Ctrl Pts',(-0.120677496364249,-0.22332526623541,
-0.60793326972845));
#52533=CARTESIAN_POINT('Ctrl Pts',(0.122490316820947,-0.222336130561283,
-0.595213996907462));
#52534=CARTESIAN_POINT('Ctrl Pts',(0.253253489411948,-0.0173177010175265,
-0.582494724086478));
#52535=CARTESIAN_POINT('Ctrl Pts',(0.151615700070685,0.203592514989958,
-0.569775451265491));
#52536=CARTESIAN_POINT('Ctrl Pts',(-0.0891539710159297,0.237673730395159,
-0.557056178444505));
#52537=CARTESIAN_POINT('Ctrl Pts',(-0.248110480624322,0.0536509279717373,
-0.544336905623519));
#52538=CARTESIAN_POINT('Ctrl Pts',(-0.17938556915355,-0.179605262304078,
-0.531617632802533));
#52539=CARTESIAN_POINT('Ctrl Pts',(0.0539545621305916,-0.248044628833514,
-0.518898359981547));
#52540=CARTESIAN_POINT('Ctrl Pts',(0.237782672202715,-0.0888630039330099,
-0.506179087160561));
#52541=CARTESIAN_POINT('Ctrl Pts',(0.203406792750139,0.151864773173242,
-0.493459814339576));
#52542=CARTESIAN_POINT('Ctrl Pts',(-0.0176276571665515,0.253232103752022,
-0.480740541518589));
#52543=CARTESIAN_POINT('Ctrl Pts',(-0.222485885813322,0.122218097194056,
-0.468021268697603));
#52544=CARTESIAN_POINT('Ctrl Pts',(-0.223177395970049,-0.120950744503174,
-0.455301995876617));
#52545=CARTESIAN_POINT('Ctrl Pts',(-0.0190676154303742,-0.253127751757173,
-0.442582723055631));
#52546=CARTESIAN_POINT('Ctrl Pts',(0.20253978055438,-0.15301918167648,-0.429863450234645));
#52547=CARTESIAN_POINT('Ctrl Pts',(0.238284229734968,0.0875091911020926,
-0.417144177413659));
#52548=CARTESIAN_POINT('Ctrl Pts',(0.055364429384439,0.247733753507101,
-0.404424904592674));
#52549=CARTESIAN_POINT('Ctrl Pts',(-0.178361172995562,0.180622602783104,
-0.391705631771686));
#52550=CARTESIAN_POINT('Ctrl Pts',(-0.248411604412052,-0.0522389458188462,
-0.378986358950701));
#52551=CARTESIAN_POINT('Ctrl Pts',(-0.0905042850685891,-0.237162828141114,
-0.366267086129715));
#52552=CARTESIAN_POINT('Ctrl Pts',(0.150455326907289,-0.204451527940497,
-0.353547813308729));
#52553=CARTESIAN_POINT('Ctrl Pts',(0.253347886817307,0.0158770559379742,
-0.340828540487743));
#52554=CARTESIAN_POINT('Ctrl Pts',(0.123752859991858,0.221635877765367,
-0.328109267666758));
#52555=CARTESIAN_POINT('Ctrl Pts',(-0.119405394719161,0.22400800076304,
-0.315389994845771));
#52556=CARTESIAN_POINT('Ctrl Pts',(-0.25298992269341,0.0208166189771321,
-0.302670722024786));
#52557=CARTESIAN_POINT('Ctrl Pts',(-0.154415354136274,-0.201477371184718,
-0.289951449203799));
#52558=CARTESIAN_POINT('Ctrl Pts',(0.085860231485404,-0.238883347004778,
-0.277232176382814));
#52559=CARTESIAN_POINT('Ctrl Pts',(0.247345191988348,-0.0570752858103143,
-0.264512903561827));
#52560=CARTESIAN_POINT('Ctrl Pts',(0.181851009958456,0.177108563115757,
-0.251793630740842));
#52561=CARTESIAN_POINT('Ctrl Pts',(-0.0505208369423248,0.248766715286243,
-0.239074357919855));
#52562=CARTESIAN_POINT('Ctrl Pts',(-0.236531650119936,0.0921412405259361,
-0.22635508509887));
#52563=CARTESIAN_POINT('Ctrl Pts',(-0.20548650701387,-0.149038688975162,
-0.213635812277883));
#52564=CARTESIAN_POINT('Ctrl Pts',(0.0141257154305693,-0.253451577178313,
-0.200916539456898));
#52565=CARTESIAN_POINT('Ctrl Pts',(0.220775246249027,-0.12528169405219,
-0.188197266635911));
#52566=CARTESIAN_POINT('Ctrl Pts',(0.224827974726504,0.11785430813562,-0.175477993814926));
#52567=CARTESIAN_POINT('Ctrl Pts',(0.0225644957220879,0.252840071987673,
-0.162758720993939));
#52568=CARTESIAN_POINT('Ctrl Pts',(-0.200405085303683,0.155804030335518,
-0.150039448172954));
#52569=CARTESIAN_POINT('Ctrl Pts',(-0.239471534501604,-0.0842069414154272,
-0.137320175351968));
#52570=CARTESIAN_POINT('Ctrl Pts',(-0.0587824989353668,-0.246945252072248,
-0.124600902530982));
#52571=CARTESIAN_POINT('Ctrl Pts',(0.17584574554195,-0.183069898264903,
-0.111881629709996));
#52572=CARTESIAN_POINT('Ctrl Pts',(0.249113274073944,0.048798728524302,
-0.0991623568890095));
#52573=CARTESIAN_POINT('Ctrl Pts',(0.0937674461211858,0.235892196932982,
-0.0864430840680236));
#52574=CARTESIAN_POINT('Ctrl Pts',(-0.147602831630382,0.206505907852829,
-0.0737238112470377));
#52575=CARTESIAN_POINT('Ctrl Pts',(-0.253566226457987,-0.0123627143772766,
-0.0610045384260517));
#52576=CARTESIAN_POINT('Ctrl Pts',(-0.126760550998478,-0.219925029716766,
-0.0482852656050658));
#52577=CARTESIAN_POINT('Ctrl Pts',(0.116213473458248,-0.225597061096139,
-0.0355659927840799));
#52578=CARTESIAN_POINT('Ctrl Pts',(0.252840833129579,-0.0243895398283461,
-0.0228467199630935));
#52579=CARTESIAN_POINT('Ctrl Pts',(0.156854624655317,0.199487263968605,
-0.0101274471421078));
#52580=CARTESIAN_POINT('Ctrl Pts',(-0.00221290875354078,0.226244402213306,
-0.00164793192811709));
#52581=CARTESIAN_POINT('Ctrl Pts',(-0.0698093673657148,0.202998596068486,
0.00259182567887824));
#52582=CARTESIAN_POINT('Ctrl Pts',(0.0326814423280649,0.196779569448552,
-1.51495));
#52583=CARTESIAN_POINT('Ctrl Pts',(-0.0328441439546247,0.207662155862942,
-1.51071024239301));
#52584=CARTESIAN_POINT('Ctrl Pts',(-0.174482908049702,0.158625293378044,
-1.50223072717901));
#52585=CARTESIAN_POINT('Ctrl Pts',(-0.227933689275854,-0.061320949657441,
-1.48951145435803));
#52586=CARTESIAN_POINT('Ctrl Pts',(-0.0717210652972735,-0.224640326086787,
-1.47679218153704));
#52587=CARTESIAN_POINT('Ctrl Pts',(0.150056091147136,-0.181992142895108,
-1.46407290871606));
#52588=CARTESIAN_POINT('Ctrl Pts',(0.234263183139456,0.0277545022598852,
-1.45135363589507));
#52589=CARTESIAN_POINT('Ctrl Pts',(0.103427579470953,0.211984146348435,
-1.43863436307408));
#52590=CARTESIAN_POINT('Ctrl Pts',(-0.122283649797262,0.201709159043015,
-1.4259150902531));
#52591=CARTESIAN_POINT('Ctrl Pts',(-0.235798710471342,0.00632031506446229,
-1.41319581743211));
#52592=CARTESIAN_POINT('Ctrl Pts',(-0.132920511685779,-0.194861544684569,
-1.40047654461113));
#52593=CARTESIAN_POINT('Ctrl Pts',(0.0919285341003431,-0.217230095550597,
-1.38775727179014));
#52594=CARTESIAN_POINT('Ctrl Pts',(0.232421027333792,-0.0402530662671006,
-1.37503799896916));
#52595=CARTESIAN_POINT('Ctrl Pts',(0.159628279467637,0.173661654101238,
-1.36231872614817));
#52596=CARTESIAN_POINT('Ctrl Pts',(-0.059648436931805,0.228214293208638,
-1.34959945332718));
#52597=CARTESIAN_POINT('Ctrl Pts',(-0.224188475417309,0.0733432011409307,
-1.3368801805062));
#52598=CARTESIAN_POINT('Ctrl Pts',(-0.182999188568635,-0.148831974728763,
-1.32416090768521));
#52599=CARTESIAN_POINT('Ctrl Pts',(0.0261212891997552,-0.23442986171762,
-1.31144163486423));
#52600=CARTESIAN_POINT('Ctrl Pts',(0.211271323804121,-0.104900464490951,
-1.29872236204324));
#52601=CARTESIAN_POINT('Ctrl Pts',(0.202545781291298,0.120892023328345,
-1.28600308922225));
#52602=CARTESIAN_POINT('Ctrl Pts',(0.00795180094256099,0.2357465737612,
-1.27328381640127));
#52603=CARTESIAN_POINT('Ctrl Pts',(-0.193939248706097,0.134265577980045,
-1.26056454358028));
#52604=CARTESIAN_POINT('Ctrl Pts',(-0.217859723699137,-0.0904257585137644,
-1.24784527075929));
#52605=CARTESIAN_POINT('Ctrl Pts',(-0.0418587330474375,-0.232136864756142,
-1.23512599793831));
#52606=CARTESIAN_POINT('Ctrl Pts',(0.172554404057684,-0.16082492044269,
-1.22240672511732));
#52607=CARTESIAN_POINT('Ctrl Pts',(0.228621017531538,0.0580698516161886,
-1.20968745229634));
#52608=CARTESIAN_POINT('Ctrl Pts',(0.0748909390303039,0.223676160212552,
-1.19696817947535));
#52609=CARTESIAN_POINT('Ctrl Pts',(-0.147563666640709,0.18402348127975,
-1.18424890665437));
#52610=CARTESIAN_POINT('Ctrl Pts',(-0.234604785311441,-0.0245004505269651,
-1.17152963383338));
#52611=CARTESIAN_POINT('Ctrl Pts',(-0.106358138767262,-0.21054126364045,
-1.15881036101239));
#52612=CARTESIAN_POINT('Ctrl Pts',(0.11948927064294,-0.203376477437402,
-1.14609108819141));
#52613=CARTESIAN_POINT('Ctrl Pts',(0.23568598380503,-0.00958093997281493,
-1.13337181537042));
#52614=CARTESIAN_POINT('Ctrl Pts',(0.13560275754475,0.193006656674328,-1.12065254254944));
#52615=CARTESIAN_POINT('Ctrl Pts',(-0.0889178905577564,0.218479486708672,
-1.10793326972845));
#52616=CARTESIAN_POINT('Ctrl Pts',(-0.231842019113515,0.0434621162283831,
-1.09521399690746));
#52617=CARTESIAN_POINT('Ctrl Pts',(-0.162013666417545,-0.171438762442514,
-1.08249472408648));
#52618=CARTESIAN_POINT('Ctrl Pts',(0.0564883808015244,-0.229016899394345,
-1.06977545126549));
#52619=CARTESIAN_POINT('Ctrl Pts',(0.223153219116496,-0.0764350585250314,
-1.0570561784445));
#52620=CARTESIAN_POINT('Ctrl Pts',(0.1850389529013,0.146288288263266,-1.04433690562352));
#52621=CARTESIAN_POINT('Ctrl Pts',(-0.022878425401603,0.234768513700057,
-1.03161763280253));
#52622=CARTESIAN_POINT('Ctrl Pts',(-0.209801154891635,0.107810726645952,
-1.01889835998155));
#52623=CARTESIAN_POINT('Ctrl Pts',(-0.204197454343028,-0.118080807134871,
-1.00617908716056));
#52624=CARTESIAN_POINT('Ctrl Pts',(-0.011209623673909,-0.235614137332382,
-0.993459814339576));
#52625=CARTESIAN_POINT('Ctrl Pts',(0.192064846404454,-0.136933458838324,
-0.980740541518589));
#52626=CARTESIAN_POINT('Ctrl Pts',(0.219088812841539,0.0874057747604746,
-0.968021268697603));
#52627=CARTESIAN_POINT('Ctrl Pts',(0.045063423665798,0.231536099175291,
-0.955301995876618));
#52628=CARTESIAN_POINT('Ctrl Pts',(-0.170314931789737,0.163194673268617,
-0.942582723055631));
#52629=CARTESIAN_POINT('Ctrl Pts',(-0.22940184158239,-0.0549042116089614,
-0.929863450234646));
#52630=CARTESIAN_POINT('Ctrl Pts',(-0.0779755269508779,-0.222619618566124,
-0.917144177413659));
#52631=CARTESIAN_POINT('Ctrl Pts',(0.145005922074389,-0.186045585642739,
-0.904424904592673));
#52632=CARTESIAN_POINT('Ctrl Pts',(0.234921027752471,0.0212553074199478,
-0.891705631771688));
#52633=CARTESIAN_POINT('Ctrl Pts',(0.109258164674579,0.209051024455123,
-0.878986358950702));
#52634=CARTESIAN_POINT('Ctrl Pts',(-0.116666703196555,0.20500867722865,
-0.866267086129715));
#52635=CARTESIAN_POINT('Ctrl Pts',(-0.235531036141585,0.0128377719198042,
-0.853547813308731));
#52636=CARTESIAN_POINT('Ctrl Pts',(-0.138257619153505,-0.19111386166314,
-0.840828540487742));
#52637=CARTESIAN_POINT('Ctrl Pts',(0.0858894838017356,-0.219687673632512,
-0.828109267666759));
#52638=CARTESIAN_POINT('Ctrl Pts',(0.23121911931857,-0.0466625785328924,
-0.81538999484577));
#52639=CARTESIAN_POINT('Ctrl Pts',(0.164367884705876,0.169182965605612,
-0.802670722024787));
#52640=CARTESIAN_POINT('Ctrl Pts',(-0.0533174197753734,0.229775825800475,
-0.789951449203798));
#52641=CARTESIAN_POINT('Ctrl Pts',(-0.222075384016159,0.0795122706748416,
-0.777232176382814));
#52642=CARTESIAN_POINT('Ctrl Pts',(-0.187043331437545,-0.143716629304121,
-0.764512903561827));
#52643=CARTESIAN_POINT('Ctrl Pts',(0.0196311741237908,-0.235062320196826,
-0.751793630740842));
#52644=CARTESIAN_POINT('Ctrl Pts',(0.208290908157902,-0.110700383705523,
-0.739074357919856));
#52645=CARTESIAN_POINT('Ctrl Pts',(0.205810107346701,0.115247026372627,
-0.726355085098869));
#52646=CARTESIAN_POINT('Ctrl Pts',(0.0144653069364513,0.235436684204114,
-0.713635812277884));
#52647=CARTESIAN_POINT('Ctrl Pts',(-0.190153747875909,0.139575175237355,
-0.700916539456897));
#52648=CARTESIAN_POINT('Ctrl Pts',(-0.220276040475835,-0.0843690901105478,
-0.688197266635912));
#52649=CARTESIAN_POINT('Ctrl Pts',(-0.0482595044417223,-0.23089109468499,
-0.675477993814925));
#52650=CARTESIAN_POINT('Ctrl Pts',(0.168042917961313,-0.165533244687709,
-0.662758720993941));
#52651=CARTESIAN_POINT('Ctrl Pts',(0.230138834184335,0.0517280810978802,
-0.650039448172953));
#52652=CARTESIAN_POINT('Ctrl Pts',(0.0810452162903746,0.221520541463405,
-0.637320175351968));
#52653=CARTESIAN_POINT('Ctrl Pts',(-0.142420471538835,0.1880321426258,-0.624600902530982));
#52654=CARTESIAN_POINT('Ctrl Pts',(-0.235192384283932,-0.018006103094028,
-0.611881629709995));
#52655=CARTESIAN_POINT('Ctrl Pts',(-0.112137314847476,-0.207520842308891,
-0.599162356889011));
#52656=CARTESIAN_POINT('Ctrl Pts',(0.113821844477603,-0.206601706414806,
-0.586443084068023));
#52657=CARTESIAN_POINT('Ctrl Pts',(0.235331086026933,-0.0160921509804536,
-0.573723811247038));
#52658=CARTESIAN_POINT('Ctrl Pts',(0.140886064153414,0.189184550905072,
-0.561004538426052));
#52659=CARTESIAN_POINT('Ctrl Pts',(-0.0828446663124362,0.22085388526665,
-0.548285265605067));
#52660=CARTESIAN_POINT('Ctrl Pts',(-0.230552040943494,0.0498541251110027,
-0.535565992784079));
#52661=CARTESIAN_POINT('Ctrl Pts',(-0.16669069754769,-0.16689484331416,
-0.522846719963095));
#52662=CARTESIAN_POINT('Ctrl Pts',(0.0501362714953425,-0.230490849393937,
-0.510127447142107));
#52663=CARTESIAN_POINT('Ctrl Pts',(0.220955117411352,-0.0825742905723761,
-0.497408174321123));
#52664=CARTESIAN_POINT('Ctrl Pts',(0.189011971974381,0.141117510692855,
-0.484688901500136));
#52665=CARTESIAN_POINT('Ctrl Pts',(-0.0163801719563586,0.235311213800938,
-0.47196962867915));
#52666=CARTESIAN_POINT('Ctrl Pts',(-0.206740863692295,0.113568889461726,
-0.459250355858164));
#52667=CARTESIAN_POINT('Ctrl Pts',(-0.207383436620149,-0.112391225588995,
-0.446531083037178));
#52668=CARTESIAN_POINT('Ctrl Pts',(-0.0177182263414914,-0.235214246654171,
-0.433811810216192));
#52669=CARTESIAN_POINT('Ctrl Pts',(0.188206317046981,-0.142190223283767,
-0.421092537395206));
#52670=CARTESIAN_POINT('Ctrl Pts',(0.221421180402404,0.081316285225576,
-0.40837326457422));
#52671=CARTESIAN_POINT('Ctrl Pts',(0.051446364370158,0.230201974289577,
-0.395653991753234));
#52672=CARTESIAN_POINT('Ctrl Pts',(-0.165738796506009,0.167840187997636,
-0.382934718932248));
#52673=CARTESIAN_POINT('Ctrl Pts',(-0.230831854612239,-0.048542067005659,
-0.370215446111262));
#52674=CARTESIAN_POINT('Ctrl Pts',(-0.0840994204847348,-0.220379138866998,
-0.357496173290276));
#52675=CARTESIAN_POINT('Ctrl Pts',(0.139807809013192,-0.189982772682906,
-0.344776900469291));
#52676=CARTESIAN_POINT('Ctrl Pts',(0.235418803056905,0.014753458384602,
-0.332057627648304));
#52677=CARTESIAN_POINT('Ctrl Pts',(0.11499503919352,0.205951009552392,-0.319338354827319));
#52678=CARTESIAN_POINT('Ctrl Pts',(-0.110955238097539,0.208155260646928,
-0.306619082006331));
#52679=CARTESIAN_POINT('Ctrl Pts',(-0.235086171564913,0.0193434552971877,
-0.293899809185347));
#52680=CARTESIAN_POINT('Ctrl Pts',(-0.143487590526395,-0.18721909293667,
-0.28118053636436));
#52681=CARTESIAN_POINT('Ctrl Pts',(0.0797840202277238,-0.221977898961698,
-0.268461263543375));
#52682=CARTESIAN_POINT('Ctrl Pts',(0.229840910738551,-0.0530361458245903,
-0.255741990722388));
#52683=CARTESIAN_POINT('Ctrl Pts',(0.168981662475758,0.164574832115758,
-0.243022717901402));
#52684=CARTESIAN_POINT('Ctrl Pts',(-0.0469455463466026,0.231161834775108,
-0.230303445080416));
#52685=CARTESIAN_POINT('Ctrl Pts',(-0.219792628451899,0.0856205308411988,
-0.217584172259431));
#52686=CARTESIAN_POINT('Ctrl Pts',(-0.190944507701513,-0.138491424611743,
-0.204864899438444));
#52687=CARTESIAN_POINT('Ctrl Pts',(0.0131260578517699,-0.235515155392752,
-0.192145626617459));
#52688=CARTESIAN_POINT('Ctrl Pts',(0.205151283752445,-0.116415679756492,
-0.179426353796472));
#52689=CARTESIAN_POINT('Ctrl Pts',(0.208917206173459,0.109513919792018,
-0.166707080975487));
#52690=CARTESIAN_POINT('Ctrl Pts',(0.0209676371933062,0.234946925588856,
-0.1539878081545));
#52691=CARTESIAN_POINT('Ctrl Pts',(-0.186222691262201,0.144777992008589,
-0.141268535333515));
#52692=CARTESIAN_POINT('Ctrl Pts',(-0.222524461233109,-0.078247731236845,
-0.128549262512529));
#52693=CARTESIAN_POINT('Ctrl Pts',(-0.0546225418096208,-0.229469274023813,
-0.115829989691543));
#52694=CARTESIAN_POINT('Ctrl Pts',(0.16340138241606,-0.170114291722319,
-0.103110716870557));
#52695=CARTESIAN_POINT('Ctrl Pts',(0.231483868070962,0.0453453091881316,
-0.0903914440495704));
#52696=CARTESIAN_POINT('Ctrl Pts',(0.0871316520886174,0.219198428493199,
-0.0776721712285846));
#52697=CARTESIAN_POINT('Ctrl Pts',(-0.137157180929212,0.191891766936069,
-0.0649528984075987));
#52698=CARTESIAN_POINT('Ctrl Pts',(-0.235621691099566,-0.0114878219739488,
-0.0522336255866127));
#52699=CARTESIAN_POINT('Ctrl Pts',(-0.117789880017489,-0.204361235882386,
-0.0395143527656268));
#52700=CARTESIAN_POINT('Ctrl Pts',(0.10798920474263,-0.20963186535164,-0.0267950799446408));
#52701=CARTESIAN_POINT('Ctrl Pts',(0.23494763286579,-0.0226635254220135,
-0.0140758071236545));
#52702=CARTESIAN_POINT('Ctrl Pts',(0.14575423720397,0.18536982288884,-0.00135653430266873));
#52703=CARTESIAN_POINT('Ctrl Pts',(-0.00205630422490502,0.210233395022512,
0.00712298091132193));
#52704=CARTESIAN_POINT('Ctrl Pts',(-0.0648690538289269,0.188632662814105,
0.0113627385183173));
#52705=CARTESIAN_POINT('Ctrl Pts',(-0.0796899944392906,0.231730462577249,
-0.0149499999999998));
#52706=CARTESIAN_POINT('Ctrl Pts',(-0.00252611781081202,0.258266416594894,
-0.0191897576069952));
#52707=CARTESIAN_POINT('Ctrl Pts',(0.0882646408735982,0.242994281361514,
-0.0234295152139904));
#52708=CARTESIAN_POINT('Ctrl Pts',(0.151921992565662,0.1927642612833,-0.0276692728209858));
#52709=CARTESIAN_POINT('Ctrl Pts',(0.215579344257725,0.142534241205086,
-0.031909030427981));
#52710=CARTESIAN_POINT('Ctrl Pts',(0.252103288957442,0.0573463362820363,
-0.0361487880349764));
#52711=CARTESIAN_POINT('Ctrl Pts',(0.244371057512688,-0.0235285968368411,
-0.0403885456419717));
#52712=CARTESIAN_POINT('Ctrl Pts',(0.236638826067934,-0.10440352995572,
-0.0446283032489671));
#52713=CARTESIAN_POINT('Ctrl Pts',(0.184650418478711,-0.180965491270427,
-0.0488680608559624));
#52714=CARTESIAN_POINT('Ctrl Pts',(0.112428897375775,-0.218167332727847,
-0.0531078184629578));
#52715=CARTESIAN_POINT('Ctrl Pts',(0.0402073762728397,-0.255369174185266,
-0.0573475760699531));
#52716=CARTESIAN_POINT('Ctrl Pts',(-0.0522472583438086,-0.253210895785397,
-0.0615873336769485));
#52717=CARTESIAN_POINT('Ctrl Pts',(-0.122600143021194,-0.212641736885196,
-0.0658270912839438));
#52718=CARTESIAN_POINT('Ctrl Pts',(-0.19295302769858,-0.172072577984995,
-0.0700668488909392));
#52719=CARTESIAN_POINT('Ctrl Pts',(-0.241204162436703,-0.0930925385844643,
-0.0743066064979345));
#52720=CARTESIAN_POINT('Ctrl Pts',(-0.245169535782081,-0.0119614040724845,
-0.0785463641049298));
#52721=CARTESIAN_POINT('Ctrl Pts',(-0.245363103914123,-0.00800101981856802,
-0.0787533261962178));
#52722=CARTESIAN_POINT('Ctrl Pts',(-0.245451145027683,-0.00403550979405535,
-0.0789602882875058));
#52723=CARTESIAN_POINT('Ctrl Pts',(-0.245435813781494,-6.93175206961383E-5,
-0.0791672503787938));
#52724=CARTESIAN_POINT('Origin',(0.425436949301274,-0.075016012752114,0.04));
#52725=CARTESIAN_POINT('',(0.418820640002835,-0.0722099128071448,0.04));
#52726=CARTESIAN_POINT('',(0.418259909571329,-0.0753899731090502,0.04));
#52727=CARTESIAN_POINT('Origin',(0.,0.,0.04));
#52728=CARTESIAN_POINT('',(0.412634448512115,-0.0727585864424439,0.04));
#52729=CARTESIAN_POINT('',(0.439454987334101,-0.0703797847906986,0.04));
#52730=CARTESIAN_POINT('',(0.412634448512115,-0.0727585864424439,0.04));
#52731=CARTESIAN_POINT('Origin',(0.412634448512115,-0.0727585864424439,
0.04));
#52732=CARTESIAN_POINT('',(0.418259909571329,-0.0753899731090502,0.485));
#52733=CARTESIAN_POINT('',(0.418259909571329,-0.0753899731090502,0.2425));
#52734=CARTESIAN_POINT('',(0.412634448512115,-0.0727585864424439,0.491));
#52735=CARTESIAN_POINT('',(0.412634448512115,-0.0727585864424439,0.04));
#52736=CARTESIAN_POINT('Ctrl Pts',(0.41825990957133,-0.0753899731090502,
0.485));
#52737=CARTESIAN_POINT('Ctrl Pts',(0.415427183327153,-0.0740649265056499,
0.488022849530655));
#52738=CARTESIAN_POINT('Ctrl Pts',(0.412634448512115,-0.0727585864424439,
0.491));
#52739=CARTESIAN_POINT('Origin',(0.439454987334101,-0.0703797847906986,
0.04));
#52740=CARTESIAN_POINT('',(0.418820640002835,-0.0722099128071448,0.485));
#52741=CARTESIAN_POINT('',(0.418820640002835,-0.0722099128071448,0.2425));
#52742=CARTESIAN_POINT('Ctrl Pts',(0.412634448512115,-0.0727585864424439,
0.491));
#52743=CARTESIAN_POINT('Ctrl Pts',(0.415705555425236,-0.0724861998865247,
0.488022849530686));
#52744=CARTESIAN_POINT('Ctrl Pts',(0.418820640002835,-0.0722099128071448,
0.485));
#52745=CARTESIAN_POINT('Origin',(0.405947212179512,-0.147752701916689,0.04));
#52746=CARTESIAN_POINT('',(0.399918693627878,-0.143840322882602,0.04));
#52747=CARTESIAN_POINT('',(0.398814270275285,-0.146874701105371,0.04));
#52748=CARTESIAN_POINT('Origin',(0.,0.,0.04));
#52749=CARTESIAN_POINT('',(0.393731208109296,-0.143306440053456,0.04));
#52750=CARTESIAN_POINT('',(0.420557357253009,-0.145621115434422,0.04));
#52751=CARTESIAN_POINT('',(0.393731208109296,-0.143306440053456,0.04));
#52752=CARTESIAN_POINT('Origin',(0.393731208109296,-0.143306440053456,0.04));
#52753=CARTESIAN_POINT('',(0.398814270275285,-0.146874701105371,0.485));
#52754=CARTESIAN_POINT('',(0.398814270275285,-0.146874701105371,0.2425));
#52755=CARTESIAN_POINT('',(0.393731208109296,-0.143306440053456,0.491));
#52756=CARTESIAN_POINT('',(0.393731208109296,-0.143306440053456,0.04));
#52757=CARTESIAN_POINT('Ctrl Pts',(0.398814270275285,-0.146874701105371,
0.485));
#52758=CARTESIAN_POINT('Ctrl Pts',(0.396254671435792,-0.14507788718706,
0.488022849530738));
#52759=CARTESIAN_POINT('Ctrl Pts',(0.393731208109296,-0.143306440053456,
0.491));
#52760=CARTESIAN_POINT('Origin',(0.420557357253009,-0.145621115434422,0.04));
#52761=CARTESIAN_POINT('',(0.399918693627878,-0.143840322882602,0.485));
#52762=CARTESIAN_POINT('',(0.399918693627878,-0.143840322882602,0.2425));
#52763=CARTESIAN_POINT('Ctrl Pts',(0.393731208109296,-0.143306440053456,
0.491));
#52764=CARTESIAN_POINT('Ctrl Pts',(0.396802957436579,-0.143571483780241,
0.488022849530825));
#52765=CARTESIAN_POINT('Ctrl Pts',(0.399918693627878,-0.143840322882602,
0.485));
#52766=CARTESIAN_POINT('Origin',(0.374122974434878,-0.216,0.04));
#52767=CARTESIAN_POINT('',(0.368865420115662,-0.211100217533986,0.04));
#52768=CARTESIAN_POINT('',(0.367250861186684,-0.21389671563079,0.04));
#52769=CARTESIAN_POINT('Origin',(0.,0.,0.04));
#52770=CARTESIAN_POINT('',(0.36286464418568,-0.2095,0.04));
#52771=CARTESIAN_POINT('',(0.388881304684075,-0.216437822173509,0.04));
#52772=CARTESIAN_POINT('',(0.36286464418568,-0.2095,0.04));
#52773=CARTESIAN_POINT('Origin',(0.36286464418568,-0.2095,0.04));
#52774=CARTESIAN_POINT('',(0.367250861186684,-0.21389671563079,0.485));
#52775=CARTESIAN_POINT('',(0.367250861186684,-0.21389671563079,0.2425));
#52776=CARTESIAN_POINT('',(0.36286464418568,-0.2095,0.491));
#52777=CARTESIAN_POINT('',(0.36286464418568,-0.2095,0.04));
#52778=CARTESIAN_POINT('Ctrl Pts',(0.367250861186684,-0.21389671563079,
0.485));
#52779=CARTESIAN_POINT('Ctrl Pts',(0.365042161867486,-0.211682729679295,
0.488022849530718));
#52780=CARTESIAN_POINT('Ctrl Pts',(0.36286464418568,-0.2095,0.491));
#52781=CARTESIAN_POINT('Origin',(0.388881304684075,-0.216437822173509,0.04));
#52782=CARTESIAN_POINT('',(0.368865420115662,-0.211100217533986,0.485));
#52783=CARTESIAN_POINT('',(0.368865420115662,-0.211100217533986,0.2425));
#52784=CARTESIAN_POINT('Ctrl Pts',(0.36286464418568,-0.2095,0.491));
#52785=CARTESIAN_POINT('Ctrl Pts',(0.365843702378499,-0.210294420790001,
0.488022849530667));
#52786=CARTESIAN_POINT('Ctrl Pts',(0.368865420115662,-0.211100217533986,
0.485));
#52787=CARTESIAN_POINT('Origin',(0.330931199427399,-0.277684247384585,0.04));
#52788=CARTESIAN_POINT('',(0.32660435746814,-0.271945938897464,0.04));
#52789=CARTESIAN_POINT('',(0.324528720518828,-0.274419586688728,0.04));
#52790=CARTESIAN_POINT('Origin',(0.,0.,0.04));
#52791=CARTESIAN_POINT('',(0.320972621666852,-0.26932800845866,0.04));
#52792=CARTESIAN_POINT('',(0.345389290455751,-0.280678175208677,0.04));
#52793=CARTESIAN_POINT('',(0.320972621666852,-0.26932800845866,0.04));
#52794=CARTESIAN_POINT('Origin',(0.320972621666852,-0.26932800845866,0.04));
#52795=CARTESIAN_POINT('',(0.324528720518828,-0.274419586688728,0.485));
#52796=CARTESIAN_POINT('',(0.324528720518828,-0.274419586688728,0.2425));
#52797=CARTESIAN_POINT('',(0.320972621666852,-0.26932800845866,0.491));
#52798=CARTESIAN_POINT('',(0.320972621666852,-0.26932800845866,0.04));
#52799=CARTESIAN_POINT('Ctrl Pts',(0.324528720518828,-0.274419586688728,
0.485));
#52800=CARTESIAN_POINT('Ctrl Pts',(0.322738030931108,-0.271855699546901,
0.488022849530649));
#52801=CARTESIAN_POINT('Ctrl Pts',(0.320972621666852,-0.26932800845866,
0.491));
#52802=CARTESIAN_POINT('Origin',(0.345389290455751,-0.280678175208677,0.04));
#52803=CARTESIAN_POINT('',(0.32660435746814,-0.271945938897464,0.485));
#52804=CARTESIAN_POINT('',(0.32660435746814,-0.271945938897464,0.2425));
#52805=CARTESIAN_POINT('Ctrl Pts',(0.320972621666852,-0.26932800845866,
0.491));
#52806=CARTESIAN_POINT('Ctrl Pts',(0.323768471549298,-0.270627668238139,
0.4880228495307));
#52807=CARTESIAN_POINT('Ctrl Pts',(0.32660435746814,-0.271945938897464,
0.485));
#52808=CARTESIAN_POINT('Origin',(0.277684247384585,-0.330931199427399,0.04));
#52809=CARTESIAN_POINT('',(0.274419586688728,-0.324528720518828,0.04));
#52810=CARTESIAN_POINT('',(0.271945938897464,-0.32660435746814,0.04));
#52811=CARTESIAN_POINT('Origin',(0.,0.,0.04));
#52812=CARTESIAN_POINT('',(0.26932800845866,-0.320972621666852,0.04));
#52813=CARTESIAN_POINT('',(0.291402797412343,-0.33639026392014,0.04));
#52814=CARTESIAN_POINT('',(0.26932800845866,-0.320972621666852,0.04));
#52815=CARTESIAN_POINT('Origin',(0.26932800845866,-0.320972621666852,0.04));
#52816=CARTESIAN_POINT('',(0.271945938897464,-0.32660435746814,0.485));
#52817=CARTESIAN_POINT('',(0.271945938897464,-0.32660435746814,0.2425));
#52818=CARTESIAN_POINT('',(0.26932800845866,-0.320972621666852,0.491));
#52819=CARTESIAN_POINT('',(0.26932800845866,-0.320972621666852,0.04));
#52820=CARTESIAN_POINT('Ctrl Pts',(0.271945938897464,-0.32660435746814,
0.485));
#52821=CARTESIAN_POINT('Ctrl Pts',(0.270627668238179,-0.323768471549385,
0.488022849530608));
#52822=CARTESIAN_POINT('Ctrl Pts',(0.26932800845866,-0.320972621666852,
0.491));
#52823=CARTESIAN_POINT('Origin',(0.291402797412343,-0.33639026392014,0.04));
#52824=CARTESIAN_POINT('',(0.274419586688728,-0.324528720518828,0.485));
#52825=CARTESIAN_POINT('',(0.274419586688728,-0.324528720518828,0.2425));
#52826=CARTESIAN_POINT('Ctrl Pts',(0.26932800845866,-0.320972621666852,
0.491));
#52827=CARTESIAN_POINT('Ctrl Pts',(0.271855699546945,-0.322738030931138,
0.488022849530598));
#52828=CARTESIAN_POINT('Ctrl Pts',(0.274419586688728,-0.324528720518828,
0.485));
#52829=CARTESIAN_POINT('Origin',(0.216,-0.374122974434878,0.04));
#52830=CARTESIAN_POINT('',(0.21389671563079,-0.367250861186684,0.04));
#52831=CARTESIAN_POINT('',(0.211100217533986,-0.368865420115662,0.04));
#52832=CARTESIAN_POINT('Origin',(0.,0.,0.04));
#52833=CARTESIAN_POINT('',(0.2095,-0.36286464418568,0.04));
#52834=CARTESIAN_POINT('',(0.228562177826491,-0.381881304684075,0.04));
#52835=CARTESIAN_POINT('',(0.2095,-0.36286464418568,0.04));
#52836=CARTESIAN_POINT('Origin',(0.2095,-0.36286464418568,0.04));
#52837=CARTESIAN_POINT('',(0.211100217533986,-0.368865420115662,0.485));
#52838=CARTESIAN_POINT('',(0.211100217533986,-0.368865420115662,0.2425));
#52839=CARTESIAN_POINT('',(0.2095,-0.36286464418568,0.491));
#52840=CARTESIAN_POINT('',(0.2095,-0.36286464418568,0.04));
#52841=CARTESIAN_POINT('Ctrl Pts',(0.211100217533986,-0.368865420115662,
0.485));
#52842=CARTESIAN_POINT('Ctrl Pts',(0.210294420789968,-0.365843702378377,
0.488022849530788));
#52843=CARTESIAN_POINT('Ctrl Pts',(0.2095,-0.36286464418568,0.491));
#52844=CARTESIAN_POINT('Origin',(0.228562177826491,-0.381881304684075,0.04));
#52845=CARTESIAN_POINT('',(0.21389671563079,-0.367250861186684,0.485));
#52846=CARTESIAN_POINT('',(0.21389671563079,-0.367250861186684,0.2425));
#52847=CARTESIAN_POINT('Ctrl Pts',(0.2095,-0.36286464418568,0.491));
#52848=CARTESIAN_POINT('Ctrl Pts',(0.211682729679329,-0.36504216186752,
0.488022849530672));
#52849=CARTESIAN_POINT('Ctrl Pts',(0.21389671563079,-0.367250861186684,
0.485));
#52850=CARTESIAN_POINT('Origin',(0.147752701916689,-0.405947212179513,0.04));
#52851=CARTESIAN_POINT('',(0.146874701105371,-0.398814270275285,0.04));
#52852=CARTESIAN_POINT('',(0.143840322882601,-0.399918693627879,0.04));
#52853=CARTESIAN_POINT('Origin',(0.,0.,0.04));
#52854=CARTESIAN_POINT('',(0.143306440053455,-0.393731208109296,0.04));
#52855=CARTESIAN_POINT('',(0.158776812125424,-0.41576907524645,0.04));
#52856=CARTESIAN_POINT('',(0.143306440053455,-0.393731208109296,0.04));
#52857=CARTESIAN_POINT('Origin',(0.143306440053455,-0.393731208109296,0.04));
#52858=CARTESIAN_POINT('',(0.143840322882601,-0.399918693627878,0.485));
#52859=CARTESIAN_POINT('',(0.143840322882601,-0.399918693627878,0.2425));
#52860=CARTESIAN_POINT('',(0.143306440053455,-0.393731208109296,0.491));
#52861=CARTESIAN_POINT('',(0.143306440053455,-0.393731208109296,0.04));
#52862=CARTESIAN_POINT('Ctrl Pts',(0.143840322882601,-0.399918693627879,
0.485));
#52863=CARTESIAN_POINT('Ctrl Pts',(0.143571483780255,-0.396802957436743,
0.488022849530666));
#52864=CARTESIAN_POINT('Ctrl Pts',(0.143306440053455,-0.393731208109296,
0.491));
#52865=CARTESIAN_POINT('Origin',(0.158776812125424,-0.41576907524645,0.04));
#52866=CARTESIAN_POINT('',(0.146874701105371,-0.398814270275285,0.485));
#52867=CARTESIAN_POINT('',(0.146874701105371,-0.398814270275285,0.2425));
#52868=CARTESIAN_POINT('Ctrl Pts',(0.143306440053455,-0.393731208109296,
0.491));
#52869=CARTESIAN_POINT('Ctrl Pts',(0.145077887187091,-0.396254671435837,
0.488022849530685));
#52870=CARTESIAN_POINT('Ctrl Pts',(0.146874701105371,-0.398814270275285,
0.485));
#52871=CARTESIAN_POINT('Origin',(0.0750160127521138,-0.425436949301274,
0.04));
#52872=CARTESIAN_POINT('',(0.07538997310905,-0.418259909571329,0.04));
#52873=CARTESIAN_POINT('',(0.0722099128071446,-0.418820640002835,0.04));
#52874=CARTESIAN_POINT('Origin',(0.,0.,0.04));
#52875=CARTESIAN_POINT('',(0.0727585864424437,-0.412634448512115,0.04));
#52876=CARTESIAN_POINT('',(0.0841670933328693,-0.437023912846764,0.04));
#52877=CARTESIAN_POINT('',(0.0727585864424437,-0.412634448512115,0.04));
#52878=CARTESIAN_POINT('Origin',(0.0727585864424437,-0.412634448512115,
0.04));
#52879=CARTESIAN_POINT('',(0.0722099128071446,-0.418820640002835,0.485));
#52880=CARTESIAN_POINT('',(0.0722099128071446,-0.418820640002835,0.2425));
#52881=CARTESIAN_POINT('',(0.0727585864424437,-0.412634448512115,0.491));
#52882=CARTESIAN_POINT('',(0.0727585864424437,-0.412634448512115,0.04));
#52883=CARTESIAN_POINT('Ctrl Pts',(0.0722099128071446,-0.418820640002835,
0.485));
#52884=CARTESIAN_POINT('Ctrl Pts',(0.0724861998865257,-0.415705555425222,
0.488022849530699));
#52885=CARTESIAN_POINT('Ctrl Pts',(0.0727585864424437,-0.412634448512115,
0.491));
#52886=CARTESIAN_POINT('Origin',(0.0841670933328693,-0.437023912846764,
0.04));
#52887=CARTESIAN_POINT('',(0.07538997310905,-0.418259909571329,0.485));
#52888=CARTESIAN_POINT('',(0.07538997310905,-0.418259909571329,0.2425));
#52889=CARTESIAN_POINT('Ctrl Pts',(0.0727585864424437,-0.412634448512115,
0.491));
#52890=CARTESIAN_POINT('Ctrl Pts',(0.0740649265056506,-0.415427183327155,
0.488022849530653));
#52891=CARTESIAN_POINT('Ctrl Pts',(0.07538997310905,-0.41825990957133,0.485));
#52892=CARTESIAN_POINT('Origin',(-6.93889390390723E-17,-0.432,0.04));
#52893=CARTESIAN_POINT('',(0.00161455892897798,-0.424996933164776,0.04));
#52894=CARTESIAN_POINT('',(-0.00161455892897815,-0.424996933164776,0.04));
#52895=CARTESIAN_POINT('Origin',(0.,0.,0.04));
#52896=CARTESIAN_POINT('',(-9.71445146547012E-17,-0.419,0.04));
#52897=CARTESIAN_POINT('',(0.00699999999999992,-0.445,0.04));
#52898=CARTESIAN_POINT('',(-9.71445146547012E-17,-0.419,0.04));
#52899=CARTESIAN_POINT('Origin',(-9.71445146547012E-17,-0.419,0.04));
#52900=CARTESIAN_POINT('',(-0.00161455892897816,-0.424996933164776,0.485));
#52901=CARTESIAN_POINT('',(-0.00161455892897816,-0.424996933164776,0.2425));
#52902=CARTESIAN_POINT('',(-9.71445146547012E-17,-0.419,0.491));
#52903=CARTESIAN_POINT('',(-9.71445146547012E-17,-0.419,0.04));
#52904=CARTESIAN_POINT('Ctrl Pts',(-0.00161455892897818,-0.424996933164776,
0.485));
#52905=CARTESIAN_POINT('Ctrl Pts',(-0.000801540510914313,-0.42197715046911,
0.48802284953089));
#52906=CARTESIAN_POINT('Ctrl Pts',(-9.71445146547012E-17,-0.419,0.491));
#52907=CARTESIAN_POINT('Origin',(0.00699999999999992,-0.445,0.04));
#52908=CARTESIAN_POINT('',(0.00161455892897797,-0.424996933164776,0.485));
#52909=CARTESIAN_POINT('',(0.00161455892897797,-0.424996933164776,0.2425));
#52910=CARTESIAN_POINT('Ctrl Pts',(-9.71445146547012E-17,-0.419,0.491));
#52911=CARTESIAN_POINT('Ctrl Pts',(0.000801540510959919,-0.42197715046928,
0.48802284953072));
#52912=CARTESIAN_POINT('Ctrl Pts',(0.00161455892897797,-0.424996933164776,
0.485));
#52913=CARTESIAN_POINT('Origin',(-0.0750160127521139,-0.425436949301274,
0.04));
#52914=CARTESIAN_POINT('',(-0.0722099128071448,-0.418820640002835,0.04));
#52915=CARTESIAN_POINT('',(-0.0753899731090502,-0.418259909571329,0.04));
#52916=CARTESIAN_POINT('Origin',(0.,0.,0.04));
#52917=CARTESIAN_POINT('',(-0.0727585864424438,-0.412634448512115,0.04));
#52918=CARTESIAN_POINT('',(-0.0703797847906986,-0.439454987334101,0.04));
#52919=CARTESIAN_POINT('',(-0.0727585864424438,-0.412634448512115,0.04));
#52920=CARTESIAN_POINT('Origin',(-0.0727585864424438,-0.412634448512115,
0.04));
#52921=CARTESIAN_POINT('',(-0.0753899731090502,-0.418259909571329,0.485));
#52922=CARTESIAN_POINT('',(-0.0753899731090502,-0.418259909571329,0.2425));
#52923=CARTESIAN_POINT('',(-0.0727585864424438,-0.412634448512115,0.491));
#52924=CARTESIAN_POINT('',(-0.0727585864424438,-0.412634448512115,0.04));
#52925=CARTESIAN_POINT('Ctrl Pts',(-0.0753899731090501,-0.41825990957133,
0.485));
#52926=CARTESIAN_POINT('Ctrl Pts',(-0.0740649265055902,-0.415427183327025,
0.488022849530791));
#52927=CARTESIAN_POINT('Ctrl Pts',(-0.0727585864424438,-0.412634448512115,
0.491));
#52928=CARTESIAN_POINT('Origin',(-0.0703797847906986,-0.439454987334101,
0.04));
#52929=CARTESIAN_POINT('',(-0.0722099128071448,-0.418820640002835,0.485));
#52930=CARTESIAN_POINT('',(-0.0722099128071448,-0.418820640002835,0.2425));
#52931=CARTESIAN_POINT('Ctrl Pts',(-0.0727585864424438,-0.412634448512115,
0.491));
#52932=CARTESIAN_POINT('Ctrl Pts',(-0.0724861998865248,-0.415705555425234,
0.488022849530688));
#52933=CARTESIAN_POINT('Ctrl Pts',(-0.0722099128071448,-0.418820640002835,
0.485));
#52934=CARTESIAN_POINT('Origin',(-0.147752701916689,-0.405947212179512,
0.04));
#52935=CARTESIAN_POINT('',(-0.143840322882602,-0.399918693627878,0.04));
#52936=CARTESIAN_POINT('',(-0.146874701105371,-0.398814270275285,0.04));
#52937=CARTESIAN_POINT('Origin',(0.,0.,0.04));
#52938=CARTESIAN_POINT('',(-0.143306440053455,-0.393731208109296,0.04));
#52939=CARTESIAN_POINT('',(-0.145621115434422,-0.420557357253009,0.04));
#52940=CARTESIAN_POINT('',(-0.143306440053455,-0.393731208109296,0.04));
#52941=CARTESIAN_POINT('Origin',(-0.143306440053455,-0.393731208109296,
0.04));
#52942=CARTESIAN_POINT('',(-0.146874701105371,-0.398814270275285,0.485));
#52943=CARTESIAN_POINT('',(-0.146874701105371,-0.398814270275285,0.2425));
#52944=CARTESIAN_POINT('',(-0.143306440053455,-0.393731208109296,0.491));
#52945=CARTESIAN_POINT('',(-0.143306440053455,-0.393731208109296,0.04));
#52946=CARTESIAN_POINT('Ctrl Pts',(-0.146874701105371,-0.398814270275285,
0.485));
#52947=CARTESIAN_POINT('Ctrl Pts',(-0.145077887187028,-0.396254671435746,
0.488022849530792));
#52948=CARTESIAN_POINT('Ctrl Pts',(-0.143306440053455,-0.393731208109296,
0.491));
#52949=CARTESIAN_POINT('Origin',(-0.145621115434422,-0.420557357253009,
0.04));
#52950=CARTESIAN_POINT('',(-0.143840322882602,-0.399918693627878,0.485));
#52951=CARTESIAN_POINT('',(-0.143840322882602,-0.399918693627878,0.2425));
#52952=CARTESIAN_POINT('Ctrl Pts',(-0.143306440053455,-0.393731208109296,
0.491));
#52953=CARTESIAN_POINT('Ctrl Pts',(-0.14357148378024,-0.396802957436561,
0.488022849530842));
#52954=CARTESIAN_POINT('Ctrl Pts',(-0.143840322882602,-0.399918693627878,
0.485));
#52955=CARTESIAN_POINT('Origin',(-0.216,-0.374122974434878,0.04));
#52956=CARTESIAN_POINT('',(-0.211100217533986,-0.368865420115662,0.04));
#52957=CARTESIAN_POINT('',(-0.21389671563079,-0.367250861186684,0.04));
#52958=CARTESIAN_POINT('Origin',(0.,0.,0.04));
#52959=CARTESIAN_POINT('',(-0.2095,-0.36286464418568,0.04));
#52960=CARTESIAN_POINT('',(-0.216437822173509,-0.388881304684075,0.04));
#52961=CARTESIAN_POINT('',(-0.2095,-0.36286464418568,0.04));
#52962=CARTESIAN_POINT('Origin',(-0.2095,-0.36286464418568,0.04));
#52963=CARTESIAN_POINT('',(-0.21389671563079,-0.367250861186684,0.485));
#52964=CARTESIAN_POINT('',(-0.21389671563079,-0.367250861186684,0.2425));
#52965=CARTESIAN_POINT('',(-0.2095,-0.36286464418568,0.491));
#52966=CARTESIAN_POINT('',(-0.2095,-0.36286464418568,0.04));
#52967=CARTESIAN_POINT('Ctrl Pts',(-0.21389671563079,-0.367250861186684,
0.485));
#52968=CARTESIAN_POINT('Ctrl Pts',(-0.211682729679295,-0.365042161867486,
0.488022849530718));
#52969=CARTESIAN_POINT('Ctrl Pts',(-0.2095,-0.36286464418568,0.491));
#52970=CARTESIAN_POINT('Origin',(-0.216437822173509,-0.388881304684075,
0.04));
#52971=CARTESIAN_POINT('',(-0.211100217533986,-0.368865420115662,0.485));
#52972=CARTESIAN_POINT('',(-0.211100217533986,-0.368865420115662,0.2425));
#52973=CARTESIAN_POINT('Ctrl Pts',(-0.2095,-0.36286464418568,0.491));
#52974=CARTESIAN_POINT('Ctrl Pts',(-0.210294420790001,-0.365843702378499,
0.488022849530667));
#52975=CARTESIAN_POINT('Ctrl Pts',(-0.211100217533986,-0.368865420115662,
0.485));
#52976=CARTESIAN_POINT('Origin',(-0.277684247384585,-0.330931199427399,
0.04));
#52977=CARTESIAN_POINT('',(-0.271945938897464,-0.32660435746814,0.04));
#52978=CARTESIAN_POINT('',(-0.274419586688728,-0.324528720518828,0.04));
#52979=CARTESIAN_POINT('Origin',(0.,0.,0.04));
#52980=CARTESIAN_POINT('',(-0.26932800845866,-0.320972621666852,0.04));
#52981=CARTESIAN_POINT('',(-0.280678175208677,-0.345389290455751,0.04));
#52982=CARTESIAN_POINT('',(-0.26932800845866,-0.320972621666852,0.04));
#52983=CARTESIAN_POINT('Origin',(-0.26932800845866,-0.320972621666852,0.04));
#52984=CARTESIAN_POINT('',(-0.274419586688728,-0.324528720518828,0.485));
#52985=CARTESIAN_POINT('',(-0.274419586688728,-0.324528720518828,0.2425));
#52986=CARTESIAN_POINT('',(-0.26932800845866,-0.320972621666852,0.491));
#52987=CARTESIAN_POINT('',(-0.26932800845866,-0.320972621666852,0.04));
#52988=CARTESIAN_POINT('Ctrl Pts',(-0.274419586688728,-0.324528720518828,
0.485));
#52989=CARTESIAN_POINT('Ctrl Pts',(-0.27185569954683,-0.322738030931058,
0.488022849530733));
#52990=CARTESIAN_POINT('Ctrl Pts',(-0.26932800845866,-0.320972621666852,
0.491));
#52991=CARTESIAN_POINT('Origin',(-0.280678175208677,-0.345389290455751,
0.04));
#52992=CARTESIAN_POINT('',(-0.271945938897464,-0.32660435746814,0.485));
#52993=CARTESIAN_POINT('',(-0.271945938897464,-0.32660435746814,0.2425));
#52994=CARTESIAN_POINT('Ctrl Pts',(-0.26932800845866,-0.320972621666852,
0.491));
#52995=CARTESIAN_POINT('Ctrl Pts',(-0.270627668238136,-0.323768471549293,
0.488022849530706));
#52996=CARTESIAN_POINT('Ctrl Pts',(-0.271945938897464,-0.32660435746814,
0.485));
#52997=CARTESIAN_POINT('Origin',(-0.330931199427399,-0.277684247384585,
0.04));
#52998=CARTESIAN_POINT('',(-0.324528720518828,-0.274419586688728,0.04));
#52999=CARTESIAN_POINT('',(-0.32660435746814,-0.271945938897464,0.04));
#53000=CARTESIAN_POINT('Origin',(0.,0.,0.04));
#53001=CARTESIAN_POINT('',(-0.320972621666852,-0.26932800845866,0.04));
#53002=CARTESIAN_POINT('',(-0.33639026392014,-0.291402797412343,0.04));
#53003=CARTESIAN_POINT('',(-0.320972621666852,-0.26932800845866,0.04));
#53004=CARTESIAN_POINT('Origin',(-0.320972621666852,-0.26932800845866,0.04));
#53005=CARTESIAN_POINT('',(-0.32660435746814,-0.271945938897464,0.485));
#53006=CARTESIAN_POINT('',(-0.32660435746814,-0.271945938897464,0.2425));
#53007=CARTESIAN_POINT('',(-0.320972621666852,-0.26932800845866,0.491));
#53008=CARTESIAN_POINT('',(-0.320972621666852,-0.26932800845866,0.04));
#53009=CARTESIAN_POINT('Ctrl Pts',(-0.32660435746814,-0.271945938897464,
0.485));
#53010=CARTESIAN_POINT('Ctrl Pts',(-0.32376847154923,-0.270627668238107,
0.488022849530773));
#53011=CARTESIAN_POINT('Ctrl Pts',(-0.320972621666852,-0.26932800845866,
0.491));
#53012=CARTESIAN_POINT('Origin',(-0.33639026392014,-0.291402797412343,0.04));
#53013=CARTESIAN_POINT('',(-0.324528720518828,-0.274419586688728,0.485));
#53014=CARTESIAN_POINT('',(-0.324528720518828,-0.274419586688728,0.2425));
#53015=CARTESIAN_POINT('Ctrl Pts',(-0.320972621666852,-0.26932800845866,
0.491));
#53016=CARTESIAN_POINT('Ctrl Pts',(-0.322738030931081,-0.271855699546863,
0.488022849530694));
#53017=CARTESIAN_POINT('Ctrl Pts',(-0.324528720518828,-0.274419586688728,
0.485));
#53018=CARTESIAN_POINT('Origin',(-0.374122974434878,-0.216,0.04));
#53019=CARTESIAN_POINT('',(-0.367250861186684,-0.21389671563079,0.04));
#53020=CARTESIAN_POINT('',(-0.368865420115662,-0.211100217533986,0.04));
#53021=CARTESIAN_POINT('Origin',(0.,0.,0.04));
#53022=CARTESIAN_POINT('',(-0.36286464418568,-0.2095,0.04));
#53023=CARTESIAN_POINT('',(-0.381881304684075,-0.228562177826491,0.04));
#53024=CARTESIAN_POINT('',(-0.36286464418568,-0.2095,0.04));
#53025=CARTESIAN_POINT('Origin',(-0.36286464418568,-0.2095,0.04));
#53026=CARTESIAN_POINT('',(-0.368865420115662,-0.211100217533986,0.485));
#53027=CARTESIAN_POINT('',(-0.368865420115662,-0.211100217533986,0.2425));
#53028=CARTESIAN_POINT('',(-0.36286464418568,-0.2095,0.491));
#53029=CARTESIAN_POINT('',(-0.36286464418568,-0.2095,0.04));
#53030=CARTESIAN_POINT('Ctrl Pts',(-0.368865420115662,-0.211100217533986,
0.485));
#53031=CARTESIAN_POINT('Ctrl Pts',(-0.365843702378239,-0.210294420789931,
0.488022849530926));
#53032=CARTESIAN_POINT('Ctrl Pts',(-0.36286464418568,-0.2095,0.491));
#53033=CARTESIAN_POINT('Origin',(-0.381881304684075,-0.228562177826491,
0.04));
#53034=CARTESIAN_POINT('',(-0.367250861186684,-0.21389671563079,0.485));
#53035=CARTESIAN_POINT('',(-0.367250861186684,-0.21389671563079,0.2425));
#53036=CARTESIAN_POINT('Ctrl Pts',(-0.36286464418568,-0.2095,0.491));
#53037=CARTESIAN_POINT('Ctrl Pts',(-0.365042161867381,-0.211682729679189,
0.488022849530862));
#53038=CARTESIAN_POINT('Ctrl Pts',(-0.367250861186684,-0.21389671563079,
0.485));
#53039=CARTESIAN_POINT('Origin',(-0.405947212179513,-0.147752701916689,
0.04));
#53040=CARTESIAN_POINT('',(-0.398814270275285,-0.146874701105371,0.04));
#53041=CARTESIAN_POINT('',(-0.399918693627878,-0.143840322882602,0.04));
#53042=CARTESIAN_POINT('Origin',(0.,0.,0.04));
#53043=CARTESIAN_POINT('',(-0.393731208109296,-0.143306440053455,0.04));
#53044=CARTESIAN_POINT('',(-0.41576907524645,-0.158776812125424,0.04));
#53045=CARTESIAN_POINT('',(-0.393731208109296,-0.143306440053455,0.04));
#53046=CARTESIAN_POINT('Origin',(-0.393731208109296,-0.143306440053455,
0.04));
#53047=CARTESIAN_POINT('',(-0.399918693627878,-0.143840322882602,0.485));
#53048=CARTESIAN_POINT('',(-0.399918693627878,-0.143840322882602,0.2425));
#53049=CARTESIAN_POINT('',(-0.393731208109296,-0.143306440053455,0.491));
#53050=CARTESIAN_POINT('',(-0.393731208109296,-0.143306440053455,0.04));
#53051=CARTESIAN_POINT('Ctrl Pts',(-0.399918693627879,-0.143840322882602,
0.485));
#53052=CARTESIAN_POINT('Ctrl Pts',(-0.396802957436534,-0.143571483780237,
0.488022849530868));
#53053=CARTESIAN_POINT('Ctrl Pts',(-0.393731208109296,-0.143306440053455,
0.491));
#53054=CARTESIAN_POINT('Origin',(-0.41576907524645,-0.158776812125424,0.04));
#53055=CARTESIAN_POINT('',(-0.398814270275285,-0.146874701105371,0.485));
#53056=CARTESIAN_POINT('',(-0.398814270275285,-0.146874701105371,0.2425));
#53057=CARTESIAN_POINT('Ctrl Pts',(-0.393731208109296,-0.143306440053455,
0.491));
#53058=CARTESIAN_POINT('Ctrl Pts',(-0.39625467143586,-0.145077887187107,
0.488022849530658));
#53059=CARTESIAN_POINT('Ctrl Pts',(-0.398814270275285,-0.146874701105371,
0.485));
#53060=CARTESIAN_POINT('Origin',(-0.425436949301274,-0.0750160127521138,
0.04));
#53061=CARTESIAN_POINT('',(-0.418259909571329,-0.07538997310905,0.04));
#53062=CARTESIAN_POINT('',(-0.418820640002835,-0.0722099128071447,0.04));
#53063=CARTESIAN_POINT('Origin',(0.,0.,0.04));
#53064=CARTESIAN_POINT('',(-0.412634448512115,-0.0727585864424437,0.04));
#53065=CARTESIAN_POINT('',(-0.437023912846764,-0.0841670933328693,0.04));
#53066=CARTESIAN_POINT('',(-0.412634448512115,-0.0727585864424437,0.04));
#53067=CARTESIAN_POINT('Origin',(-0.412634448512115,-0.0727585864424437,
0.04));
#53068=CARTESIAN_POINT('',(-0.418820640002835,-0.0722099128071447,0.485));
#53069=CARTESIAN_POINT('',(-0.418820640002835,-0.0722099128071447,0.2425));
#53070=CARTESIAN_POINT('',(-0.412634448512115,-0.0727585864424437,0.491));
#53071=CARTESIAN_POINT('',(-0.412634448512115,-0.0727585864424437,0.04));
#53072=CARTESIAN_POINT('Ctrl Pts',(-0.418820640002835,-0.0722099128071447,
0.485));
#53073=CARTESIAN_POINT('Ctrl Pts',(-0.415705555425184,-0.0724861998865291,
0.488022849530736));
#53074=CARTESIAN_POINT('Ctrl Pts',(-0.412634448512115,-0.0727585864424437,
0.491));
#53075=CARTESIAN_POINT('Origin',(-0.437023912846764,-0.0841670933328693,
0.04));
#53076=CARTESIAN_POINT('',(-0.418259909571329,-0.07538997310905,0.485));
#53077=CARTESIAN_POINT('',(-0.418259909571329,-0.07538997310905,0.2425));
#53078=CARTESIAN_POINT('Ctrl Pts',(-0.412634448512115,-0.0727585864424437,
0.491));
#53079=CARTESIAN_POINT('Ctrl Pts',(-0.415427183326978,-0.0740649265055678,
0.488022849530841));
#53080=CARTESIAN_POINT('Ctrl Pts',(-0.41825990957133,-0.0753899731090501,
0.485));
#53081=CARTESIAN_POINT('Origin',(-0.432,5.55111512312578E-17,0.04));
#53082=CARTESIAN_POINT('',(-0.424996933164776,-0.00161455892897799,0.04));
#53083=CARTESIAN_POINT('',(-0.425,-5.20474889637625E-17,0.04));
#53084=CARTESIAN_POINT('Origin',(0.,0.,0.04));
#53085=CARTESIAN_POINT('',(-0.419,5.55111512312578E-17,0.04));
#53086=CARTESIAN_POINT('',(-0.445,-0.00699999999999995,0.04));
#53087=CARTESIAN_POINT('',(-0.424996933164776,0.0016145589289781,0.04));
#53088=CARTESIAN_POINT('',(-0.419,5.55111512312578E-17,0.04));
#53089=CARTESIAN_POINT('Origin',(0.,0.,0.04));
#53090=CARTESIAN_POINT('Origin',(-0.419,5.55111512312578E-17,0.04));
#53091=CARTESIAN_POINT('',(-0.424996933164776,0.0016145589289781,0.485));
#53092=CARTESIAN_POINT('',(-0.424996933164776,0.0016145589289781,0.2425));
#53093=CARTESIAN_POINT('',(-0.419,5.55111512312578E-17,0.491));
#53094=CARTESIAN_POINT('',(-0.419,5.55111512312578E-17,0.04));
#53095=CARTESIAN_POINT('Ctrl Pts',(-0.424996933164776,0.00161455892897809,
0.485));
#53096=CARTESIAN_POINT('Ctrl Pts',(-0.421977150469231,0.000801540510946881,
0.488022849530769));
#53097=CARTESIAN_POINT('Ctrl Pts',(-0.419,5.55111512312578E-17,0.491));
#53098=CARTESIAN_POINT('Origin',(-0.445,-0.00699999999999995,0.04));
#53099=CARTESIAN_POINT('',(-0.424996933164776,-0.00161455892897801,0.485));
#53100=CARTESIAN_POINT('',(-0.424996933164776,-0.00161455892897801,0.2425));
#53101=CARTESIAN_POINT('Ctrl Pts',(-0.419,5.55111512312578E-17,0.491));
#53102=CARTESIAN_POINT('Ctrl Pts',(-0.421977150469289,-0.000801540510962467,
0.488022849530711));
#53103=CARTESIAN_POINT('Ctrl Pts',(-0.424996933164776,-0.001614558928978,
0.485));
#53104=CARTESIAN_POINT('Origin',(-0.425436949301274,0.0750160127521141,
0.04));
#53105=CARTESIAN_POINT('',(-0.418820640002835,0.072209912807145,0.04));
#53106=CARTESIAN_POINT('',(-0.418259909571329,0.0753899731090504,0.04));
#53107=CARTESIAN_POINT('Origin',(0.,0.,0.04));
#53108=CARTESIAN_POINT('',(-0.412634448512115,0.072758586442444,0.04));
#53109=CARTESIAN_POINT('',(-0.439454987334101,0.0703797847906988,0.04));
#53110=CARTESIAN_POINT('',(-0.412634448512115,0.072758586442444,0.04));
#53111=CARTESIAN_POINT('Origin',(-0.412634448512115,0.072758586442444,0.04));
#53112=CARTESIAN_POINT('',(-0.418259909571329,0.0753899731090503,0.485));
#53113=CARTESIAN_POINT('',(-0.418259909571329,0.0753899731090503,0.2425));
#53114=CARTESIAN_POINT('',(-0.412634448512115,0.072758586442444,0.491));
#53115=CARTESIAN_POINT('',(-0.412634448512115,0.072758586442444,0.04));
#53116=CARTESIAN_POINT('Ctrl Pts',(-0.418259909571329,0.0753899731090504,
0.485));
#53117=CARTESIAN_POINT('Ctrl Pts',(-0.415427183327084,0.0740649265056179,
0.488022849530728));
#53118=CARTESIAN_POINT('Ctrl Pts',(-0.412634448512115,0.072758586442444,
0.491));
#53119=CARTESIAN_POINT('Origin',(-0.439454987334101,0.0703797847906988,
0.04));
#53120=CARTESIAN_POINT('',(-0.418820640002835,0.072209912807145,0.485));
#53121=CARTESIAN_POINT('',(-0.418820640002835,0.072209912807145,0.2425));
#53122=CARTESIAN_POINT('Ctrl Pts',(-0.412634448512115,0.072758586442444,
0.491));
#53123=CARTESIAN_POINT('Ctrl Pts',(-0.415705555425073,0.0724861998865393,
0.488022849530844));
#53124=CARTESIAN_POINT('Ctrl Pts',(-0.418820640002835,0.072209912807145,
0.485));
#53125=CARTESIAN_POINT('Origin',(-0.405947212179513,0.147752701916689,0.04));
#53126=CARTESIAN_POINT('',(-0.399918693627878,0.143840322882602,0.04));
#53127=CARTESIAN_POINT('',(-0.398814270275285,0.146874701105371,0.04));
#53128=CARTESIAN_POINT('Origin',(0.,0.,0.04));
#53129=CARTESIAN_POINT('',(-0.393731208109296,0.143306440053455,0.04));
#53130=CARTESIAN_POINT('',(-0.420557357253009,0.145621115434421,0.04));
#53131=CARTESIAN_POINT('',(-0.393731208109296,0.143306440053455,0.04));
#53132=CARTESIAN_POINT('Origin',(-0.393731208109296,0.143306440053455,0.04));
#53133=CARTESIAN_POINT('',(-0.398814270275285,0.146874701105371,0.485));
#53134=CARTESIAN_POINT('',(-0.398814270275285,0.146874701105371,0.2425));
#53135=CARTESIAN_POINT('',(-0.393731208109296,0.143306440053455,0.491));
#53136=CARTESIAN_POINT('',(-0.393731208109296,0.143306440053455,0.04));
#53137=CARTESIAN_POINT('Ctrl Pts',(-0.398814270275285,0.146874701105371,
0.485));
#53138=CARTESIAN_POINT('Ctrl Pts',(-0.396254671435729,0.145077887187016,
0.488022849530812));
#53139=CARTESIAN_POINT('Ctrl Pts',(-0.393731208109296,0.143306440053455,
0.491));
#53140=CARTESIAN_POINT('Origin',(-0.420557357253009,0.145621115434421,0.04));
#53141=CARTESIAN_POINT('',(-0.399918693627878,0.143840322882602,0.485));
#53142=CARTESIAN_POINT('',(-0.399918693627878,0.143840322882602,0.2425));
#53143=CARTESIAN_POINT('Ctrl Pts',(-0.393731208109296,0.143306440053455,
0.491));
#53144=CARTESIAN_POINT('Ctrl Pts',(-0.396802957436554,0.143571483780239,
0.488022849530849));
#53145=CARTESIAN_POINT('Ctrl Pts',(-0.399918693627878,0.143840322882602,
0.485));
#53146=CARTESIAN_POINT('Origin',(-0.374122974434878,0.216,0.04));
#53147=CARTESIAN_POINT('',(-0.368865420115662,0.211100217533986,0.04));
#53148=CARTESIAN_POINT('',(-0.367250861186684,0.21389671563079,0.04));
#53149=CARTESIAN_POINT('Origin',(0.,0.,0.04));
#53150=CARTESIAN_POINT('',(-0.36286464418568,0.2095,0.04));
#53151=CARTESIAN_POINT('',(-0.388881304684075,0.216437822173509,0.04));
#53152=CARTESIAN_POINT('',(-0.36286464418568,0.2095,0.04));
#53153=CARTESIAN_POINT('Origin',(-0.36286464418568,0.2095,0.04));
#53154=CARTESIAN_POINT('',(-0.367250861186684,0.21389671563079,0.485));
#53155=CARTESIAN_POINT('',(-0.367250861186684,0.21389671563079,0.2425));
#53156=CARTESIAN_POINT('',(-0.36286464418568,0.2095,0.491));
#53157=CARTESIAN_POINT('',(-0.36286464418568,0.2095,0.04));
#53158=CARTESIAN_POINT('Ctrl Pts',(-0.367250861186684,0.21389671563079,
0.485));
#53159=CARTESIAN_POINT('Ctrl Pts',(-0.365042161867489,0.211682729679298,
0.488022849530715));
#53160=CARTESIAN_POINT('Ctrl Pts',(-0.36286464418568,0.2095,0.491));
#53161=CARTESIAN_POINT('Origin',(-0.388881304684075,0.216437822173509,0.04));
#53162=CARTESIAN_POINT('',(-0.368865420115662,0.211100217533986,0.485));
#53163=CARTESIAN_POINT('',(-0.368865420115662,0.211100217533986,0.2425));
#53164=CARTESIAN_POINT('Ctrl Pts',(-0.36286464418568,0.2095,0.491));
#53165=CARTESIAN_POINT('Ctrl Pts',(-0.365843702378652,0.210294420790042,
0.488022849530513));
#53166=CARTESIAN_POINT('Ctrl Pts',(-0.368865420115662,0.211100217533986,
0.485));
#53167=CARTESIAN_POINT('Origin',(-0.330931199427399,0.277684247384585,0.04));
#53168=CARTESIAN_POINT('',(-0.32660435746814,0.271945938897464,0.04));
#53169=CARTESIAN_POINT('',(-0.324528720518828,0.274419586688728,0.04));
#53170=CARTESIAN_POINT('Origin',(0.,0.,0.04));
#53171=CARTESIAN_POINT('',(-0.320972621666852,0.26932800845866,0.04));
#53172=CARTESIAN_POINT('',(-0.345389290455751,0.280678175208677,0.04));
#53173=CARTESIAN_POINT('',(-0.320972621666852,0.26932800845866,0.04));
#53174=CARTESIAN_POINT('Origin',(-0.320972621666852,0.26932800845866,0.04));
#53175=CARTESIAN_POINT('',(-0.324528720518828,0.274419586688728,0.485));
#53176=CARTESIAN_POINT('',(-0.324528720518828,0.274419586688728,0.2425));
#53177=CARTESIAN_POINT('',(-0.320972621666852,0.26932800845866,0.491));
#53178=CARTESIAN_POINT('',(-0.320972621666852,0.26932800845866,0.04));
#53179=CARTESIAN_POINT('Ctrl Pts',(-0.324528720518828,0.274419586688728,
0.485));
#53180=CARTESIAN_POINT('Ctrl Pts',(-0.322738030931058,0.27185569954683,
0.488022849530733));
#53181=CARTESIAN_POINT('Ctrl Pts',(-0.320972621666852,0.26932800845866,
0.491));
#53182=CARTESIAN_POINT('Origin',(-0.345389290455751,0.280678175208677,0.04));
#53183=CARTESIAN_POINT('',(-0.32660435746814,0.271945938897464,0.485));
#53184=CARTESIAN_POINT('',(-0.32660435746814,0.271945938897464,0.2425));
#53185=CARTESIAN_POINT('Ctrl Pts',(-0.320972621666852,0.26932800845866,
0.491));
#53186=CARTESIAN_POINT('Ctrl Pts',(-0.323768471549293,0.270627668238136,
0.488022849530706));
#53187=CARTESIAN_POINT('Ctrl Pts',(-0.32660435746814,0.271945938897464,
0.485));
#53188=CARTESIAN_POINT('Origin',(-0.277684247384585,0.330931199427399,0.04));
#53189=CARTESIAN_POINT('',(-0.274419586688728,0.324528720518828,0.04));
#53190=CARTESIAN_POINT('',(-0.271945938897464,0.32660435746814,0.04));
#53191=CARTESIAN_POINT('Origin',(0.,0.,0.04));
#53192=CARTESIAN_POINT('',(-0.26932800845866,0.320972621666852,0.04));
#53193=CARTESIAN_POINT('',(-0.291402797412343,0.336390263920139,0.04));
#53194=CARTESIAN_POINT('',(-0.26932800845866,0.320972621666852,0.04));
#53195=CARTESIAN_POINT('Origin',(-0.26932800845866,0.320972621666852,0.04));
#53196=CARTESIAN_POINT('',(-0.271945938897464,0.32660435746814,0.485));
#53197=CARTESIAN_POINT('',(-0.271945938897464,0.32660435746814,0.2425));
#53198=CARTESIAN_POINT('',(-0.26932800845866,0.320972621666852,0.491));
#53199=CARTESIAN_POINT('',(-0.26932800845866,0.320972621666852,0.04));
#53200=CARTESIAN_POINT('Ctrl Pts',(-0.271945938897464,0.32660435746814,
0.485));
#53201=CARTESIAN_POINT('Ctrl Pts',(-0.270627668238091,0.323768471549197,
0.488022849530808));
#53202=CARTESIAN_POINT('Ctrl Pts',(-0.26932800845866,0.320972621666852,
0.491));
#53203=CARTESIAN_POINT('Origin',(-0.291402797412343,0.336390263920139,0.04));
#53204=CARTESIAN_POINT('',(-0.274419586688728,0.324528720518828,0.485));
#53205=CARTESIAN_POINT('',(-0.274419586688728,0.324528720518828,0.2425));
#53206=CARTESIAN_POINT('Ctrl Pts',(-0.26932800845866,0.320972621666852,
0.491));
#53207=CARTESIAN_POINT('Ctrl Pts',(-0.271855699546817,0.322738030931049,
0.488022849530749));
#53208=CARTESIAN_POINT('Ctrl Pts',(-0.274419586688728,0.324528720518828,
0.485));
#53209=CARTESIAN_POINT('Origin',(-0.216,0.374122974434878,0.04));
#53210=CARTESIAN_POINT('',(-0.21389671563079,0.367250861186684,0.04));
#53211=CARTESIAN_POINT('',(-0.211100217533986,0.368865420115662,0.04));
#53212=CARTESIAN_POINT('Origin',(0.,0.,0.04));
#53213=CARTESIAN_POINT('',(-0.2095,0.36286464418568,0.04));
#53214=CARTESIAN_POINT('',(-0.228562177826491,0.381881304684075,0.04));
#53215=CARTESIAN_POINT('',(-0.2095,0.36286464418568,0.04));
#53216=CARTESIAN_POINT('Origin',(-0.2095,0.36286464418568,0.04));
#53217=CARTESIAN_POINT('',(-0.211100217533986,0.368865420115662,0.485));
#53218=CARTESIAN_POINT('',(-0.211100217533986,0.368865420115662,0.2425));
#53219=CARTESIAN_POINT('',(-0.2095,0.36286464418568,0.491));
#53220=CARTESIAN_POINT('',(-0.2095,0.36286464418568,0.04));
#53221=CARTESIAN_POINT('Ctrl Pts',(-0.211100217533986,0.368865420115662,
0.485));
#53222=CARTESIAN_POINT('Ctrl Pts',(-0.210294420789963,0.365843702378358,
0.488022849530807));
#53223=CARTESIAN_POINT('Ctrl Pts',(-0.2095,0.36286464418568,0.491));
#53224=CARTESIAN_POINT('Origin',(-0.228562177826491,0.381881304684075,0.04));
#53225=CARTESIAN_POINT('',(-0.21389671563079,0.367250861186684,0.485));
#53226=CARTESIAN_POINT('',(-0.21389671563079,0.367250861186684,0.2425));
#53227=CARTESIAN_POINT('Ctrl Pts',(-0.2095,0.36286464418568,0.491));
#53228=CARTESIAN_POINT('Ctrl Pts',(-0.211682729679243,0.365042161867435,
0.488022849530789));
#53229=CARTESIAN_POINT('Ctrl Pts',(-0.21389671563079,0.367250861186684,
0.485));
#53230=CARTESIAN_POINT('Origin',(-0.147752701916689,0.405947212179513,0.04));
#53231=CARTESIAN_POINT('',(-0.146874701105371,0.398814270275285,0.04));
#53232=CARTESIAN_POINT('',(-0.143840322882602,0.399918693627878,0.04));
#53233=CARTESIAN_POINT('Origin',(0.,0.,0.04));
#53234=CARTESIAN_POINT('',(-0.143306440053455,0.393731208109296,0.04));
#53235=CARTESIAN_POINT('',(-0.158776812125424,0.41576907524645,0.04));
#53236=CARTESIAN_POINT('',(-0.143306440053455,0.393731208109296,0.04));
#53237=CARTESIAN_POINT('Origin',(-0.143306440053455,0.393731208109296,0.04));
#53238=CARTESIAN_POINT('',(-0.143840322882602,0.399918693627878,0.485));
#53239=CARTESIAN_POINT('',(-0.143840322882602,0.399918693627878,0.2425));
#53240=CARTESIAN_POINT('',(-0.143306440053455,0.393731208109296,0.491));
#53241=CARTESIAN_POINT('',(-0.143306440053455,0.393731208109296,0.04));
#53242=CARTESIAN_POINT('Ctrl Pts',(-0.143840322882602,0.399918693627879,
0.485));
#53243=CARTESIAN_POINT('Ctrl Pts',(-0.143571483780237,0.396802957436534,
0.488022849530868));
#53244=CARTESIAN_POINT('Ctrl Pts',(-0.143306440053455,0.393731208109296,
0.491));
#53245=CARTESIAN_POINT('Origin',(-0.158776812125424,0.41576907524645,0.04));
#53246=CARTESIAN_POINT('',(-0.146874701105371,0.398814270275285,0.485));
#53247=CARTESIAN_POINT('',(-0.146874701105371,0.398814270275285,0.2425));
#53248=CARTESIAN_POINT('Ctrl Pts',(-0.143306440053455,0.393731208109296,
0.491));
#53249=CARTESIAN_POINT('Ctrl Pts',(-0.145077887187107,0.39625467143586,
0.488022849530658));
#53250=CARTESIAN_POINT('Ctrl Pts',(-0.146874701105371,0.398814270275285,
0.485));
#53251=CARTESIAN_POINT('Origin',(-0.0750160127521139,0.425436949301274,
0.04));
#53252=CARTESIAN_POINT('',(-0.0753899731090501,0.418259909571329,0.04));
#53253=CARTESIAN_POINT('',(-0.0722099128071448,0.418820640002835,0.04));
#53254=CARTESIAN_POINT('Origin',(0.,0.,0.04));
#53255=CARTESIAN_POINT('',(-0.0727585864424438,0.412634448512115,0.04));
#53256=CARTESIAN_POINT('',(-0.0841670933328695,0.437023912846764,0.04));
#53257=CARTESIAN_POINT('',(-0.0727585864424438,0.412634448512115,0.04));
#53258=CARTESIAN_POINT('Origin',(-0.0727585864424438,0.412634448512115,
0.04));
#53259=CARTESIAN_POINT('',(-0.0722099128071448,0.418820640002835,0.485));
#53260=CARTESIAN_POINT('',(-0.0722099128071448,0.418820640002835,0.2425));
#53261=CARTESIAN_POINT('',(-0.0727585864424438,0.412634448512115,0.491));
#53262=CARTESIAN_POINT('',(-0.0727585864424438,0.412634448512115,0.04));
#53263=CARTESIAN_POINT('Ctrl Pts',(-0.0722099128071449,0.418820640002835,
0.485));
#53264=CARTESIAN_POINT('Ctrl Pts',(-0.0724861998865278,0.4157055554252,
0.488022849530721));
#53265=CARTESIAN_POINT('Ctrl Pts',(-0.0727585864424438,0.412634448512115,
0.491));
#53266=CARTESIAN_POINT('Origin',(-0.0841670933328695,0.437023912846764,
0.04));
#53267=CARTESIAN_POINT('',(-0.0753899731090501,0.418259909571329,0.485));
#53268=CARTESIAN_POINT('',(-0.0753899731090501,0.418259909571329,0.2425));
#53269=CARTESIAN_POINT('Ctrl Pts',(-0.0727585864424438,0.412634448512115,
0.491));
#53270=CARTESIAN_POINT('Ctrl Pts',(-0.074064926505637,0.415427183327125,
0.488022849530684));
#53271=CARTESIAN_POINT('Ctrl Pts',(-0.0753899731090501,0.41825990957133,
0.485));
#53272=CARTESIAN_POINT('Origin',(2.77555756156289E-17,0.432,0.04));
#53273=CARTESIAN_POINT('',(-0.00161455892897801,0.424996933164776,0.04));
#53274=CARTESIAN_POINT('',(0.00161455892897809,0.424996933164776,0.04));
#53275=CARTESIAN_POINT('Origin',(0.,0.,0.04));
#53276=CARTESIAN_POINT('',(2.77555756156289E-17,0.419,0.04));
#53277=CARTESIAN_POINT('',(-0.00699999999999998,0.445,0.04));
#53278=CARTESIAN_POINT('',(2.77555756156289E-17,0.419,0.04));
#53279=CARTESIAN_POINT('Origin',(2.77555756156289E-17,0.419,0.04));
#53280=CARTESIAN_POINT('',(0.00161455892897809,0.424996933164776,0.485));
#53281=CARTESIAN_POINT('',(0.00161455892897809,0.424996933164776,0.2425));
#53282=CARTESIAN_POINT('',(2.77555756156289E-17,0.419,0.491));
#53283=CARTESIAN_POINT('',(2.77555756156289E-17,0.419,0.04));
#53284=CARTESIAN_POINT('Ctrl Pts',(0.00161455892897808,0.424996933164776,
0.485));
#53285=CARTESIAN_POINT('Ctrl Pts',(0.000801540510960544,0.421977150469282,
0.488022849530718));
#53286=CARTESIAN_POINT('Ctrl Pts',(2.77555756156289E-17,0.419,0.491));
#53287=CARTESIAN_POINT('Origin',(-0.00699999999999998,0.445,0.04));
#53288=CARTESIAN_POINT('',(-0.00161455892897802,0.424996933164776,0.485));
#53289=CARTESIAN_POINT('',(-0.00161455892897802,0.424996933164776,0.2425));
#53290=CARTESIAN_POINT('Ctrl Pts',(2.77555756156289E-17,0.419,0.491));
#53291=CARTESIAN_POINT('Ctrl Pts',(-0.000801540510964092,0.421977150469295,
0.488022849530705));
#53292=CARTESIAN_POINT('Ctrl Pts',(-0.00161455892897804,0.424996933164776,
0.485));
#53293=CARTESIAN_POINT('Origin',(0.075016012752114,0.425436949301274,0.04));
#53294=CARTESIAN_POINT('',(0.0722099128071449,0.418820640002835,0.04));
#53295=CARTESIAN_POINT('',(0.0753899731090502,0.418259909571329,0.04));
#53296=CARTESIAN_POINT('Origin',(0.,0.,0.04));
#53297=CARTESIAN_POINT('',(0.0727585864424439,0.412634448512115,0.04));
#53298=CARTESIAN_POINT('',(0.0703797847906986,0.439454987334101,0.04));
#53299=CARTESIAN_POINT('',(0.0727585864424439,0.412634448512115,0.04));
#53300=CARTESIAN_POINT('Origin',(0.0727585864424439,0.412634448512115,0.04));
#53301=CARTESIAN_POINT('',(0.0753899731090502,0.418259909571329,0.485));
#53302=CARTESIAN_POINT('',(0.0753899731090502,0.418259909571329,0.2425));
#53303=CARTESIAN_POINT('',(0.0727585864424439,0.412634448512115,0.491));
#53304=CARTESIAN_POINT('',(0.0727585864424439,0.412634448512115,0.04));
#53305=CARTESIAN_POINT('Ctrl Pts',(0.0753899731090502,0.41825990957133,
0.485));
#53306=CARTESIAN_POINT('Ctrl Pts',(0.0740649265056445,0.415427183327141,
0.488022849530667));
#53307=CARTESIAN_POINT('Ctrl Pts',(0.0727585864424439,0.412634448512115,
0.491));
#53308=CARTESIAN_POINT('Origin',(0.0703797847906986,0.439454987334101,0.04));
#53309=CARTESIAN_POINT('',(0.0722099128071449,0.418820640002835,0.485));
#53310=CARTESIAN_POINT('',(0.0722099128071449,0.418820640002835,0.2425));
#53311=CARTESIAN_POINT('Ctrl Pts',(0.0727585864424439,0.412634448512115,
0.491));
#53312=CARTESIAN_POINT('Ctrl Pts',(0.072486199886539,0.415705555425075,
0.488022849530842));
#53313=CARTESIAN_POINT('Ctrl Pts',(0.0722099128071449,0.418820640002835,
0.485));
#53314=CARTESIAN_POINT('Origin',(0.147752701916689,0.405947212179513,0.04));
#53315=CARTESIAN_POINT('',(0.143840322882602,0.399918693627878,0.04));
#53316=CARTESIAN_POINT('',(0.146874701105371,0.398814270275285,0.04));
#53317=CARTESIAN_POINT('Origin',(0.,0.,0.04));
#53318=CARTESIAN_POINT('',(0.143306440053455,0.393731208109296,0.04));
#53319=CARTESIAN_POINT('',(0.145621115434421,0.420557357253009,0.04));
#53320=CARTESIAN_POINT('',(0.143306440053455,0.393731208109296,0.04));
#53321=CARTESIAN_POINT('Origin',(0.143306440053455,0.393731208109296,0.04));
#53322=CARTESIAN_POINT('',(0.146874701105371,0.398814270275285,0.485));
#53323=CARTESIAN_POINT('',(0.146874701105371,0.398814270275285,0.2425));
#53324=CARTESIAN_POINT('',(0.143306440053455,0.393731208109296,0.491));
#53325=CARTESIAN_POINT('',(0.143306440053455,0.393731208109296,0.04));
#53326=CARTESIAN_POINT('Ctrl Pts',(0.146874701105371,0.398814270275285,
0.485));
#53327=CARTESIAN_POINT('Ctrl Pts',(0.145077887187016,0.396254671435729,
0.488022849530812));
#53328=CARTESIAN_POINT('Ctrl Pts',(0.143306440053455,0.393731208109296,
0.491));
#53329=CARTESIAN_POINT('Origin',(0.145621115434421,0.420557357253009,0.04));
#53330=CARTESIAN_POINT('',(0.143840322882602,0.399918693627878,0.485));
#53331=CARTESIAN_POINT('',(0.143840322882602,0.399918693627878,0.2425));
#53332=CARTESIAN_POINT('Ctrl Pts',(0.143306440053455,0.393731208109296,
0.491));
#53333=CARTESIAN_POINT('Ctrl Pts',(0.143571483780239,0.396802957436554,
0.488022849530849));
#53334=CARTESIAN_POINT('Ctrl Pts',(0.143840322882602,0.399918693627878,
0.485));
#53335=CARTESIAN_POINT('Origin',(0.216,0.374122974434878,0.04));
#53336=CARTESIAN_POINT('',(0.211100217533986,0.368865420115662,0.04));
#53337=CARTESIAN_POINT('',(0.21389671563079,0.367250861186684,0.04));
#53338=CARTESIAN_POINT('Origin',(0.,0.,0.04));
#53339=CARTESIAN_POINT('',(0.2095,0.36286464418568,0.04));
#53340=CARTESIAN_POINT('',(0.216437822173509,0.388881304684075,0.04));
#53341=CARTESIAN_POINT('',(0.2095,0.36286464418568,0.04));
#53342=CARTESIAN_POINT('Origin',(0.2095,0.36286464418568,0.04));
#53343=CARTESIAN_POINT('',(0.21389671563079,0.367250861186684,0.485));
#53344=CARTESIAN_POINT('',(0.21389671563079,0.367250861186684,0.2425));
#53345=CARTESIAN_POINT('',(0.2095,0.36286464418568,0.491));
#53346=CARTESIAN_POINT('',(0.2095,0.36286464418568,0.04));
#53347=CARTESIAN_POINT('Ctrl Pts',(0.21389671563079,0.367250861186684,0.485));
#53348=CARTESIAN_POINT('Ctrl Pts',(0.211682729679179,0.36504216186737,0.488022849530877));
#53349=CARTESIAN_POINT('Ctrl Pts',(0.2095,0.36286464418568,0.491));
#53350=CARTESIAN_POINT('Origin',(0.216437822173509,0.388881304684075,0.04));
#53351=CARTESIAN_POINT('',(0.211100217533986,0.368865420115662,0.485));
#53352=CARTESIAN_POINT('',(0.211100217533986,0.368865420115662,0.2425));
#53353=CARTESIAN_POINT('Ctrl Pts',(0.2095,0.36286464418568,0.491));
#53354=CARTESIAN_POINT('Ctrl Pts',(0.21029442079001,0.365843702378533,0.488022849530632));
#53355=CARTESIAN_POINT('Ctrl Pts',(0.211100217533986,0.368865420115662,
0.485));
#53356=CARTESIAN_POINT('Origin',(0.277684247384585,0.330931199427399,0.04));
#53357=CARTESIAN_POINT('',(0.271945938897464,0.32660435746814,0.04));
#53358=CARTESIAN_POINT('',(0.274419586688728,0.324528720518828,0.04));
#53359=CARTESIAN_POINT('Origin',(0.,0.,0.04));
#53360=CARTESIAN_POINT('',(0.26932800845866,0.320972621666852,0.04));
#53361=CARTESIAN_POINT('',(0.280678175208677,0.345389290455751,0.04));
#53362=CARTESIAN_POINT('',(0.26932800845866,0.320972621666852,0.04));
#53363=CARTESIAN_POINT('Origin',(0.26932800845866,0.320972621666852,0.04));
#53364=CARTESIAN_POINT('',(0.274419586688728,0.324528720518828,0.485));
#53365=CARTESIAN_POINT('',(0.274419586688728,0.324528720518828,0.2425));
#53366=CARTESIAN_POINT('',(0.26932800845866,0.320972621666852,0.491));
#53367=CARTESIAN_POINT('',(0.26932800845866,0.320972621666852,0.04));
#53368=CARTESIAN_POINT('Ctrl Pts',(0.274419586688728,0.324528720518828,
0.485));
#53369=CARTESIAN_POINT('Ctrl Pts',(0.271855699546927,0.322738030931126,
0.488022849530619));
#53370=CARTESIAN_POINT('Ctrl Pts',(0.26932800845866,0.320972621666852,0.491));
#53371=CARTESIAN_POINT('Origin',(0.280678175208677,0.345389290455751,0.04));
#53372=CARTESIAN_POINT('',(0.271945938897464,0.32660435746814,0.485));
#53373=CARTESIAN_POINT('',(0.271945938897464,0.32660435746814,0.2425));
#53374=CARTESIAN_POINT('Ctrl Pts',(0.26932800845866,0.320972621666852,0.491));
#53375=CARTESIAN_POINT('Ctrl Pts',(0.270627668238161,0.323768471549347,
0.488022849530649));
#53376=CARTESIAN_POINT('Ctrl Pts',(0.271945938897464,0.32660435746814,0.485));
#53377=CARTESIAN_POINT('Origin',(0.330931199427399,0.277684247384585,0.04));
#53378=CARTESIAN_POINT('',(0.324528720518828,0.274419586688728,0.04));
#53379=CARTESIAN_POINT('',(0.32660435746814,0.271945938897464,0.04));
#53380=CARTESIAN_POINT('Origin',(0.,0.,0.04));
#53381=CARTESIAN_POINT('',(0.320972621666852,0.26932800845866,0.04));
#53382=CARTESIAN_POINT('',(0.33639026392014,0.291402797412343,0.04));
#53383=CARTESIAN_POINT('',(0.320972621666852,0.26932800845866,0.04));
#53384=CARTESIAN_POINT('Origin',(0.320972621666852,0.26932800845866,0.04));
#53385=CARTESIAN_POINT('',(0.32660435746814,0.271945938897464,0.485));
#53386=CARTESIAN_POINT('',(0.32660435746814,0.271945938897464,0.2425));
#53387=CARTESIAN_POINT('',(0.320972621666852,0.26932800845866,0.491));
#53388=CARTESIAN_POINT('',(0.320972621666852,0.26932800845866,0.04));
#53389=CARTESIAN_POINT('Ctrl Pts',(0.32660435746814,0.271945938897464,0.485));
#53390=CARTESIAN_POINT('Ctrl Pts',(0.32376847154923,0.270627668238107,0.488022849530773));
#53391=CARTESIAN_POINT('Ctrl Pts',(0.320972621666852,0.26932800845866,0.491));
#53392=CARTESIAN_POINT('Origin',(0.33639026392014,0.291402797412343,0.04));
#53393=CARTESIAN_POINT('',(0.324528720518828,0.274419586688728,0.485));
#53394=CARTESIAN_POINT('',(0.324528720518828,0.274419586688728,0.2425));
#53395=CARTESIAN_POINT('Ctrl Pts',(0.320972621666852,0.26932800845866,0.491));
#53396=CARTESIAN_POINT('Ctrl Pts',(0.322738030931081,0.271855699546863,
0.488022849530694));
#53397=CARTESIAN_POINT('Ctrl Pts',(0.324528720518828,0.274419586688728,
0.485));
#53398=CARTESIAN_POINT('Origin',(0.374122974434878,0.216,0.04));
#53399=CARTESIAN_POINT('',(0.367250861186684,0.21389671563079,0.04));
#53400=CARTESIAN_POINT('',(0.368865420115662,0.211100217533986,0.04));
#53401=CARTESIAN_POINT('Origin',(0.,0.,0.04));
#53402=CARTESIAN_POINT('',(0.36286464418568,0.2095,0.04));
#53403=CARTESIAN_POINT('',(0.381881304684075,0.228562177826491,0.04));
#53404=CARTESIAN_POINT('',(0.36286464418568,0.2095,0.04));
#53405=CARTESIAN_POINT('Origin',(0.36286464418568,0.2095,0.04));
#53406=CARTESIAN_POINT('',(0.368865420115662,0.211100217533986,0.485));
#53407=CARTESIAN_POINT('',(0.368865420115662,0.211100217533986,0.2425));
#53408=CARTESIAN_POINT('',(0.36286464418568,0.2095,0.491));
#53409=CARTESIAN_POINT('',(0.36286464418568,0.2095,0.04));
#53410=CARTESIAN_POINT('Ctrl Pts',(0.368865420115662,0.211100217533986,
0.485));
#53411=CARTESIAN_POINT('Ctrl Pts',(0.365843702378372,0.210294420789967,
0.488022849530793));
#53412=CARTESIAN_POINT('Ctrl Pts',(0.36286464418568,0.2095,0.491));
#53413=CARTESIAN_POINT('Origin',(0.381881304684075,0.228562177826491,0.04));
#53414=CARTESIAN_POINT('',(0.367250861186684,0.21389671563079,0.485));
#53415=CARTESIAN_POINT('',(0.367250861186684,0.21389671563079,0.2425));
#53416=CARTESIAN_POINT('Ctrl Pts',(0.36286464418568,0.2095,0.491));
#53417=CARTESIAN_POINT('Ctrl Pts',(0.365042161867479,0.211682729679287,
0.488022849530729));
#53418=CARTESIAN_POINT('Ctrl Pts',(0.367250861186684,0.21389671563079,0.485));
#53419=CARTESIAN_POINT('Origin',(0.405947212179513,0.147752701916689,0.04));
#53420=CARTESIAN_POINT('',(0.398814270275285,0.146874701105371,0.04));
#53421=CARTESIAN_POINT('',(0.399918693627878,0.143840322882602,0.04));
#53422=CARTESIAN_POINT('Origin',(0.,0.,0.04));
#53423=CARTESIAN_POINT('',(0.393731208109296,0.143306440053455,0.04));
#53424=CARTESIAN_POINT('',(0.41576907524645,0.158776812125424,0.04));
#53425=CARTESIAN_POINT('',(0.393731208109296,0.143306440053455,0.04));
#53426=CARTESIAN_POINT('Origin',(0.393731208109296,0.143306440053455,0.04));
#53427=CARTESIAN_POINT('',(0.399918693627878,0.143840322882602,0.485));
#53428=CARTESIAN_POINT('',(0.399918693627878,0.143840322882602,0.2425));
#53429=CARTESIAN_POINT('',(0.393731208109296,0.143306440053455,0.491));
#53430=CARTESIAN_POINT('',(0.393731208109296,0.143306440053455,0.04));
#53431=CARTESIAN_POINT('Ctrl Pts',(0.399918693627879,0.143840322882602,
0.485));
#53432=CARTESIAN_POINT('Ctrl Pts',(0.396802957436534,0.143571483780237,
0.488022849530868));
#53433=CARTESIAN_POINT('Ctrl Pts',(0.393731208109296,0.143306440053455,
0.491));
#53434=CARTESIAN_POINT('Origin',(0.41576907524645,0.158776812125424,0.04));
#53435=CARTESIAN_POINT('',(0.398814270275285,0.146874701105371,0.485));
#53436=CARTESIAN_POINT('',(0.398814270275285,0.146874701105371,0.2425));
#53437=CARTESIAN_POINT('Ctrl Pts',(0.393731208109296,0.143306440053455,
0.491));
#53438=CARTESIAN_POINT('Ctrl Pts',(0.39625467143586,0.145077887187107,0.488022849530658));
#53439=CARTESIAN_POINT('Ctrl Pts',(0.398814270275285,0.146874701105371,
0.485));
#53440=CARTESIAN_POINT('Origin',(0.425436949301274,0.0750160127521139,0.04));
#53441=CARTESIAN_POINT('',(0.418259909571329,0.0753899731090502,0.04));
#53442=CARTESIAN_POINT('',(0.418820640002835,0.0722099128071448,0.04));
#53443=CARTESIAN_POINT('Origin',(0.,0.,0.04));
#53444=CARTESIAN_POINT('',(0.412634448512115,0.0727585864424438,0.04));
#53445=CARTESIAN_POINT('',(0.437023912846764,0.0841670933328695,0.04));
#53446=CARTESIAN_POINT('',(0.412634448512115,0.0727585864424438,0.04));
#53447=CARTESIAN_POINT('Origin',(0.412634448512115,0.0727585864424438,0.04));
#53448=CARTESIAN_POINT('',(0.418820640002835,0.0722099128071448,0.485));
#53449=CARTESIAN_POINT('',(0.418820640002835,0.0722099128071448,0.2425));
#53450=CARTESIAN_POINT('',(0.412634448512115,0.0727585864424438,0.491));
#53451=CARTESIAN_POINT('',(0.412634448512115,0.0727585864424438,0.04));
#53452=CARTESIAN_POINT('Ctrl Pts',(0.418820640002835,0.0722099128071448,
0.485));
#53453=CARTESIAN_POINT('Ctrl Pts',(0.415705555425232,0.072486199886525,
0.48802284953069));
#53454=CARTESIAN_POINT('Ctrl Pts',(0.412634448512115,0.0727585864424438,
0.491));
#53455=CARTESIAN_POINT('Origin',(0.437023912846764,0.0841670933328695,0.04));
#53456=CARTESIAN_POINT('',(0.418259909571329,0.0753899731090502,0.485));
#53457=CARTESIAN_POINT('',(0.418259909571329,0.0753899731090502,0.2425));
#53458=CARTESIAN_POINT('Ctrl Pts',(0.412634448512115,0.0727585864424438,
0.491));
#53459=CARTESIAN_POINT('Ctrl Pts',(0.41542718332698,0.074064926505569,0.488022849530839));
#53460=CARTESIAN_POINT('Ctrl Pts',(0.41825990957133,0.0753899731090502,
0.485));
#53461=CARTESIAN_POINT('Origin',(0.,0.,0.2425));
#53462=CARTESIAN_POINT('Origin',(0.,0.,0.485));
#53463=CARTESIAN_POINT('Origin',(0.,0.,0.485));
#53464=CARTESIAN_POINT('Origin',(0.,0.,0.485));
#53465=CARTESIAN_POINT('Origin',(0.,0.,0.485));
#53466=CARTESIAN_POINT('Origin',(0.,0.,0.485));
#53467=CARTESIAN_POINT('Origin',(0.,0.,0.485));
#53468=CARTESIAN_POINT('Origin',(0.,0.,0.485));
#53469=CARTESIAN_POINT('Origin',(0.,0.,0.485));
#53470=CARTESIAN_POINT('Origin',(0.,0.,0.485));
#53471=CARTESIAN_POINT('Origin',(0.,0.,0.485));
#53472=CARTESIAN_POINT('Origin',(0.,0.,0.485));
#53473=CARTESIAN_POINT('Origin',(0.,0.,0.485));
#53474=CARTESIAN_POINT('Origin',(0.,0.,0.485));
#53475=CARTESIAN_POINT('Origin',(0.,0.,0.485));
#53476=CARTESIAN_POINT('Origin',(0.,0.,0.485));
#53477=CARTESIAN_POINT('Origin',(0.,0.,0.485));
#53478=CARTESIAN_POINT('Origin',(0.,0.,0.485));
#53479=CARTESIAN_POINT('',(-0.425,-5.20474889637625E-17,0.));
#53480=CARTESIAN_POINT('',(-0.425,-5.20474889637625E-17,0.2425));
#53481=CARTESIAN_POINT('Origin',(0.,0.,0.));
#53482=CARTESIAN_POINT('Origin',(0.,0.,0.485));
#53483=CARTESIAN_POINT('Origin',(0.,0.,0.485));
#53484=CARTESIAN_POINT('Origin',(0.,0.,0.485));
#53485=CARTESIAN_POINT('Origin',(0.,0.,0.485));
#53486=CARTESIAN_POINT('Origin',(0.,0.,0.485));
#53487=CARTESIAN_POINT('Origin',(0.,0.,0.485));
#53488=CARTESIAN_POINT('Origin',(0.,0.,0.485));
#53489=CARTESIAN_POINT('Origin',(0.,0.,0.485));
#53490=CARTESIAN_POINT('Origin',(0.,0.,0.485));
#53491=CARTESIAN_POINT('Origin',(0.,0.,0.485));
#53492=CARTESIAN_POINT('Origin',(0.,0.,0.485));
#53493=CARTESIAN_POINT('Origin',(0.,0.,0.485));
#53494=CARTESIAN_POINT('Origin',(0.,0.,0.485));
#53495=CARTESIAN_POINT('Origin',(0.,0.,0.485));
#53496=CARTESIAN_POINT('Origin',(0.,0.,0.485));
#53497=CARTESIAN_POINT('Origin',(0.,0.,0.485));
#53498=CARTESIAN_POINT('Origin',(0.,0.,0.485));
#53499=CARTESIAN_POINT('',(0.424996933164776,0.00161455892897806,0.485));
#53500=CARTESIAN_POINT('Origin',(0.,0.,0.485));
#53501=CARTESIAN_POINT('',(0.424996933164776,0.00161455892897806,0.04));
#53502=CARTESIAN_POINT('',(0.424996933164776,0.00161455892897806,0.2425));
#53503=CARTESIAN_POINT('',(0.424996933164776,-0.00161455892897806,0.04));
#53504=CARTESIAN_POINT('Origin',(0.,0.,0.04));
#53505=CARTESIAN_POINT('',(0.424996933164776,-0.00161455892897806,0.485));
#53506=CARTESIAN_POINT('',(0.424996933164776,-0.00161455892897806,0.2425));
#53507=CARTESIAN_POINT('Origin',(0.,0.,0.485));
#53508=CARTESIAN_POINT('Origin',(0.419,0.,0.04));
#53509=CARTESIAN_POINT('',(0.419,8.67361737988404E-19,0.04));
#53510=CARTESIAN_POINT('',(0.419,0.,0.04));
#53511=CARTESIAN_POINT('',(0.419,8.67361737988404E-19,0.491));
#53512=CARTESIAN_POINT('',(0.419,8.67361737988404E-19,0.04));
#53513=CARTESIAN_POINT('Ctrl Pts',(0.424996933164776,-0.00161455892897809,
0.485));
#53514=CARTESIAN_POINT('Ctrl Pts',(0.421977150469257,-0.000801540510953786,
0.488022849530743));
#53515=CARTESIAN_POINT('Ctrl Pts',(0.419,8.67361737988404E-19,0.491));
#53516=CARTESIAN_POINT('Origin',(0.445,0.007,0.04));
#53517=CARTESIAN_POINT('Ctrl Pts',(0.419,8.67361737988404E-19,0.491));
#53518=CARTESIAN_POINT('Ctrl Pts',(0.421977150469257,0.000801540510953795,
0.488022849530743));
#53519=CARTESIAN_POINT('Ctrl Pts',(0.424996933164776,0.00161455892897809,
0.485));
#53520=CARTESIAN_POINT('',(0.445,0.007,0.04));
#53521=CARTESIAN_POINT('Origin',(0.432,0.,0.04));
#53522=CARTESIAN_POINT('Origin',(0.,0.,0.4925));
#53523=CARTESIAN_POINT('',(-0.41,-5.02105187650415E-17,0.5));
#53524=CARTESIAN_POINT('Origin',(0.,0.,0.5));
#53525=CARTESIAN_POINT('',(-0.4175,-5.1129003864402E-17,0.4925));
#53526=CARTESIAN_POINT('Origin',(0.,0.,0.192764973081037));
#53527=CARTESIAN_POINT('',(0.,0.,0.134529946162075));
#53528=CARTESIAN_POINT('',(-0.183165823577449,2.24313439557311E-17,0.25));
#53529=CARTESIAN_POINT('',(-0.0923760430703401,-1.1312802546399E-17,0.192764973081037));
#53530=CARTESIAN_POINT('Origin',(0.,0.,0.25));
#53531=CARTESIAN_POINT('Origin',(2.77555756156289E-17,0.23094010767585,
0.5));
#53532=CARTESIAN_POINT('',(1.41410031829988E-17,0.23094010767585,0.5));
#53533=CARTESIAN_POINT('',(0.2,0.115470053837925,0.5));
#53534=CARTESIAN_POINT('',(0.05,0.202072594216369,0.5));
#53535=CARTESIAN_POINT('',(2.77555756156289E-17,0.23094010767585,0.25));
#53536=CARTESIAN_POINT('',(1.41410031829988E-17,0.23094010767585,0.5));
#53537=CARTESIAN_POINT('',(0.2,0.115470053837925,0.25));
#53538=CARTESIAN_POINT('',(0.2,0.115470053837925,0.25));
#53539=CARTESIAN_POINT('',(0.2,0.115470053837925,0.5));
#53540=CARTESIAN_POINT('Origin',(-0.2,0.115470053837925,0.5));
#53541=CARTESIAN_POINT('',(-0.2,0.115470053837925,0.5));
#53542=CARTESIAN_POINT('',(-0.15,0.144337567297406,0.5));
#53543=CARTESIAN_POINT('',(-0.2,0.115470053837925,0.25));
#53544=CARTESIAN_POINT('',(-0.2,0.115470053837925,0.5));
#53545=CARTESIAN_POINT('',(1.41410031829988E-17,0.23094010767585,0.25));
#53546=CARTESIAN_POINT('Origin',(-0.2,-0.115470053837925,0.5));
#53547=CARTESIAN_POINT('',(-0.2,-0.115470053837925,0.5));
#53548=CARTESIAN_POINT('',(-0.2,-0.0577350269189626,0.5));
#53549=CARTESIAN_POINT('',(-0.2,-0.115470053837925,0.25));
#53550=CARTESIAN_POINT('',(-0.2,-0.115470053837925,0.5));
#53551=CARTESIAN_POINT('',(-0.2,0.115470053837925,0.25));
#53552=CARTESIAN_POINT('Origin',(-5.55111512312578E-17,-0.23094010767585,
0.5));
#53553=CARTESIAN_POINT('',(-4.24230095489963E-17,-0.23094010767585,0.5));
#53554=CARTESIAN_POINT('',(-0.0500000000000001,-0.202072594216369,0.5));
#53555=CARTESIAN_POINT('',(-5.55111512312578E-17,-0.23094010767585,0.25));
#53556=CARTESIAN_POINT('',(-4.24230095489963E-17,-0.23094010767585,0.5));
#53557=CARTESIAN_POINT('',(-0.2,-0.115470053837925,0.25));
#53558=CARTESIAN_POINT('Origin',(0.2,-0.115470053837925,0.5));
#53559=CARTESIAN_POINT('',(0.2,-0.115470053837925,0.5));
#53560=CARTESIAN_POINT('',(0.15,-0.144337567297407,0.5));
#53561=CARTESIAN_POINT('',(0.2,-0.115470053837925,0.25));
#53562=CARTESIAN_POINT('',(0.2,-0.115470053837925,0.5));
#53563=CARTESIAN_POINT('',(-4.24230095489963E-17,-0.23094010767585,0.25));
#53564=CARTESIAN_POINT('Origin',(0.2,0.115470053837925,0.5));
#53565=CARTESIAN_POINT('',(0.2,0.0577350269189625,0.5));
#53566=CARTESIAN_POINT('',(0.2,-0.115470053837925,0.25));
#53567=CARTESIAN_POINT('Origin',(0.,0.,0.25));
#53568=CARTESIAN_POINT('Origin',(0.19,0.,-1.6));
#53569=CARTESIAN_POINT('',(-0.19,-2.32682891837997E-17,-1.6));
#53570=CARTESIAN_POINT('Origin',(0.,0.,-1.6));
#53571=CARTESIAN_POINT('Origin',(0.,0.,-1.57));
#53572=CARTESIAN_POINT('',(-0.22,-2.69422295812418E-17,-1.57));
#53573=CARTESIAN_POINT('Origin',(0.,0.,-0.775));
#53574=CARTESIAN_POINT('Origin',(0.,0.,-0.0149499999999999));
#53575=CARTESIAN_POINT('Origin',(0.,0.,-0.005));
#53576=CARTESIAN_POINT('',(-0.26,-3.18408167778312E-17,-2.60208521396521E-18));
#53577=CARTESIAN_POINT('Origin',(0.,0.,0.));
#53578=CARTESIAN_POINT('',(-0.255,-3.12284933782575E-17,-0.005));
#53579=CARTESIAN_POINT('Origin',(0.425,0.,0.));
#53580=CARTESIAN_POINT('Origin',(0.,0.,0.5));
#53631=UNCERTAINTY_MEASURE_WITH_UNIT(LENGTH_MEASURE(0.001),#53651,
'DISTANCE_ACCURACY_VALUE',
'Maximum model space distance between geometric entities at asserted c
onnectivities');
#53632=UNCERTAINTY_MEASURE_WITH_UNIT(LENGTH_MEASURE(0.001),#53651,
'DISTANCE_ACCURACY_VALUE',
'Maximum model space distance between geometric entities at asserted c
onnectivities');
#53649=(
GEOMETRIC_REPRESENTATION_CONTEXT(3)
GLOBAL_UNCERTAINTY_ASSIGNED_CONTEXT((#53631))
GLOBAL_UNIT_ASSIGNED_CONTEXT((#53651,#53653,#53654))
REPRESENTATION_CONTEXT('','3D')
);
#53650=(
GEOMETRIC_REPRESENTATION_CONTEXT(3)
GLOBAL_UNCERTAINTY_ASSIGNED_CONTEXT((#53632))
GLOBAL_UNIT_ASSIGNED_CONTEXT((#53651,#53653,#53654))
REPRESENTATION_CONTEXT('','3D')
);
#53651=(
LENGTH_UNIT()
NAMED_UNIT(*)
SI_UNIT(.CENTI.,.METRE.)
);
#53653=(
NAMED_UNIT(*)
PLANE_ANGLE_UNIT()
SI_UNIT($,.RADIAN.)
);
#53654=(
NAMED_UNIT(*)
SI_UNIT($,.STERADIAN.)
SOLID_ANGLE_UNIT()
);
#53671=SHAPE_DEFINITION_REPRESENTATION(#53688,#53739);
#53688=PRODUCT_DEFINITION_SHAPE('',$,#53757);
#53739=SHAPE_REPRESENTATION('',(#25369),#53649);
#53740=PRODUCT_DEFINITION_CONTEXT('part definition',#53793,'design');
#53757=PRODUCT_DEFINITION('2026-10-18-22-45-13-086',
'16_ISO_4762_M5x16_A2',#53774,#53740);
#53774=PRODUCT_DEFINITION_FORMATION('',$,#53811);
#53793=APPLICATION_CONTEXT(
'Core Data for Automotive Mechanical Design Process');
#53794=PRODUCT_CONTEXT('part definition',#53793,'mechanical');
#53811=PRODUCT('2026-10-18-22-45-13-086','16_ISO_4762_M5x16_A2',$,(#53794));
#53959=COLOUR_RGB('Black',0.12,0.14,0.17);
#53960=FILL_AREA_STYLE_COLOUR('',#53959);
#53961=FILL_AREA_STYLE('',(#53960));
#53962=SURFACE_STYLE_FILL_AREA(#53961);
#53963=SURFACE_SIDE_STYLE('',(#53962));
#53964=SURFACE_STYLE_USAGE(.BOTH.,#53963);
#53965=PRESENTATION_STYLE_ASSIGNMENT((#53964));
ENDSEC;
END-ISO-10303-21;
